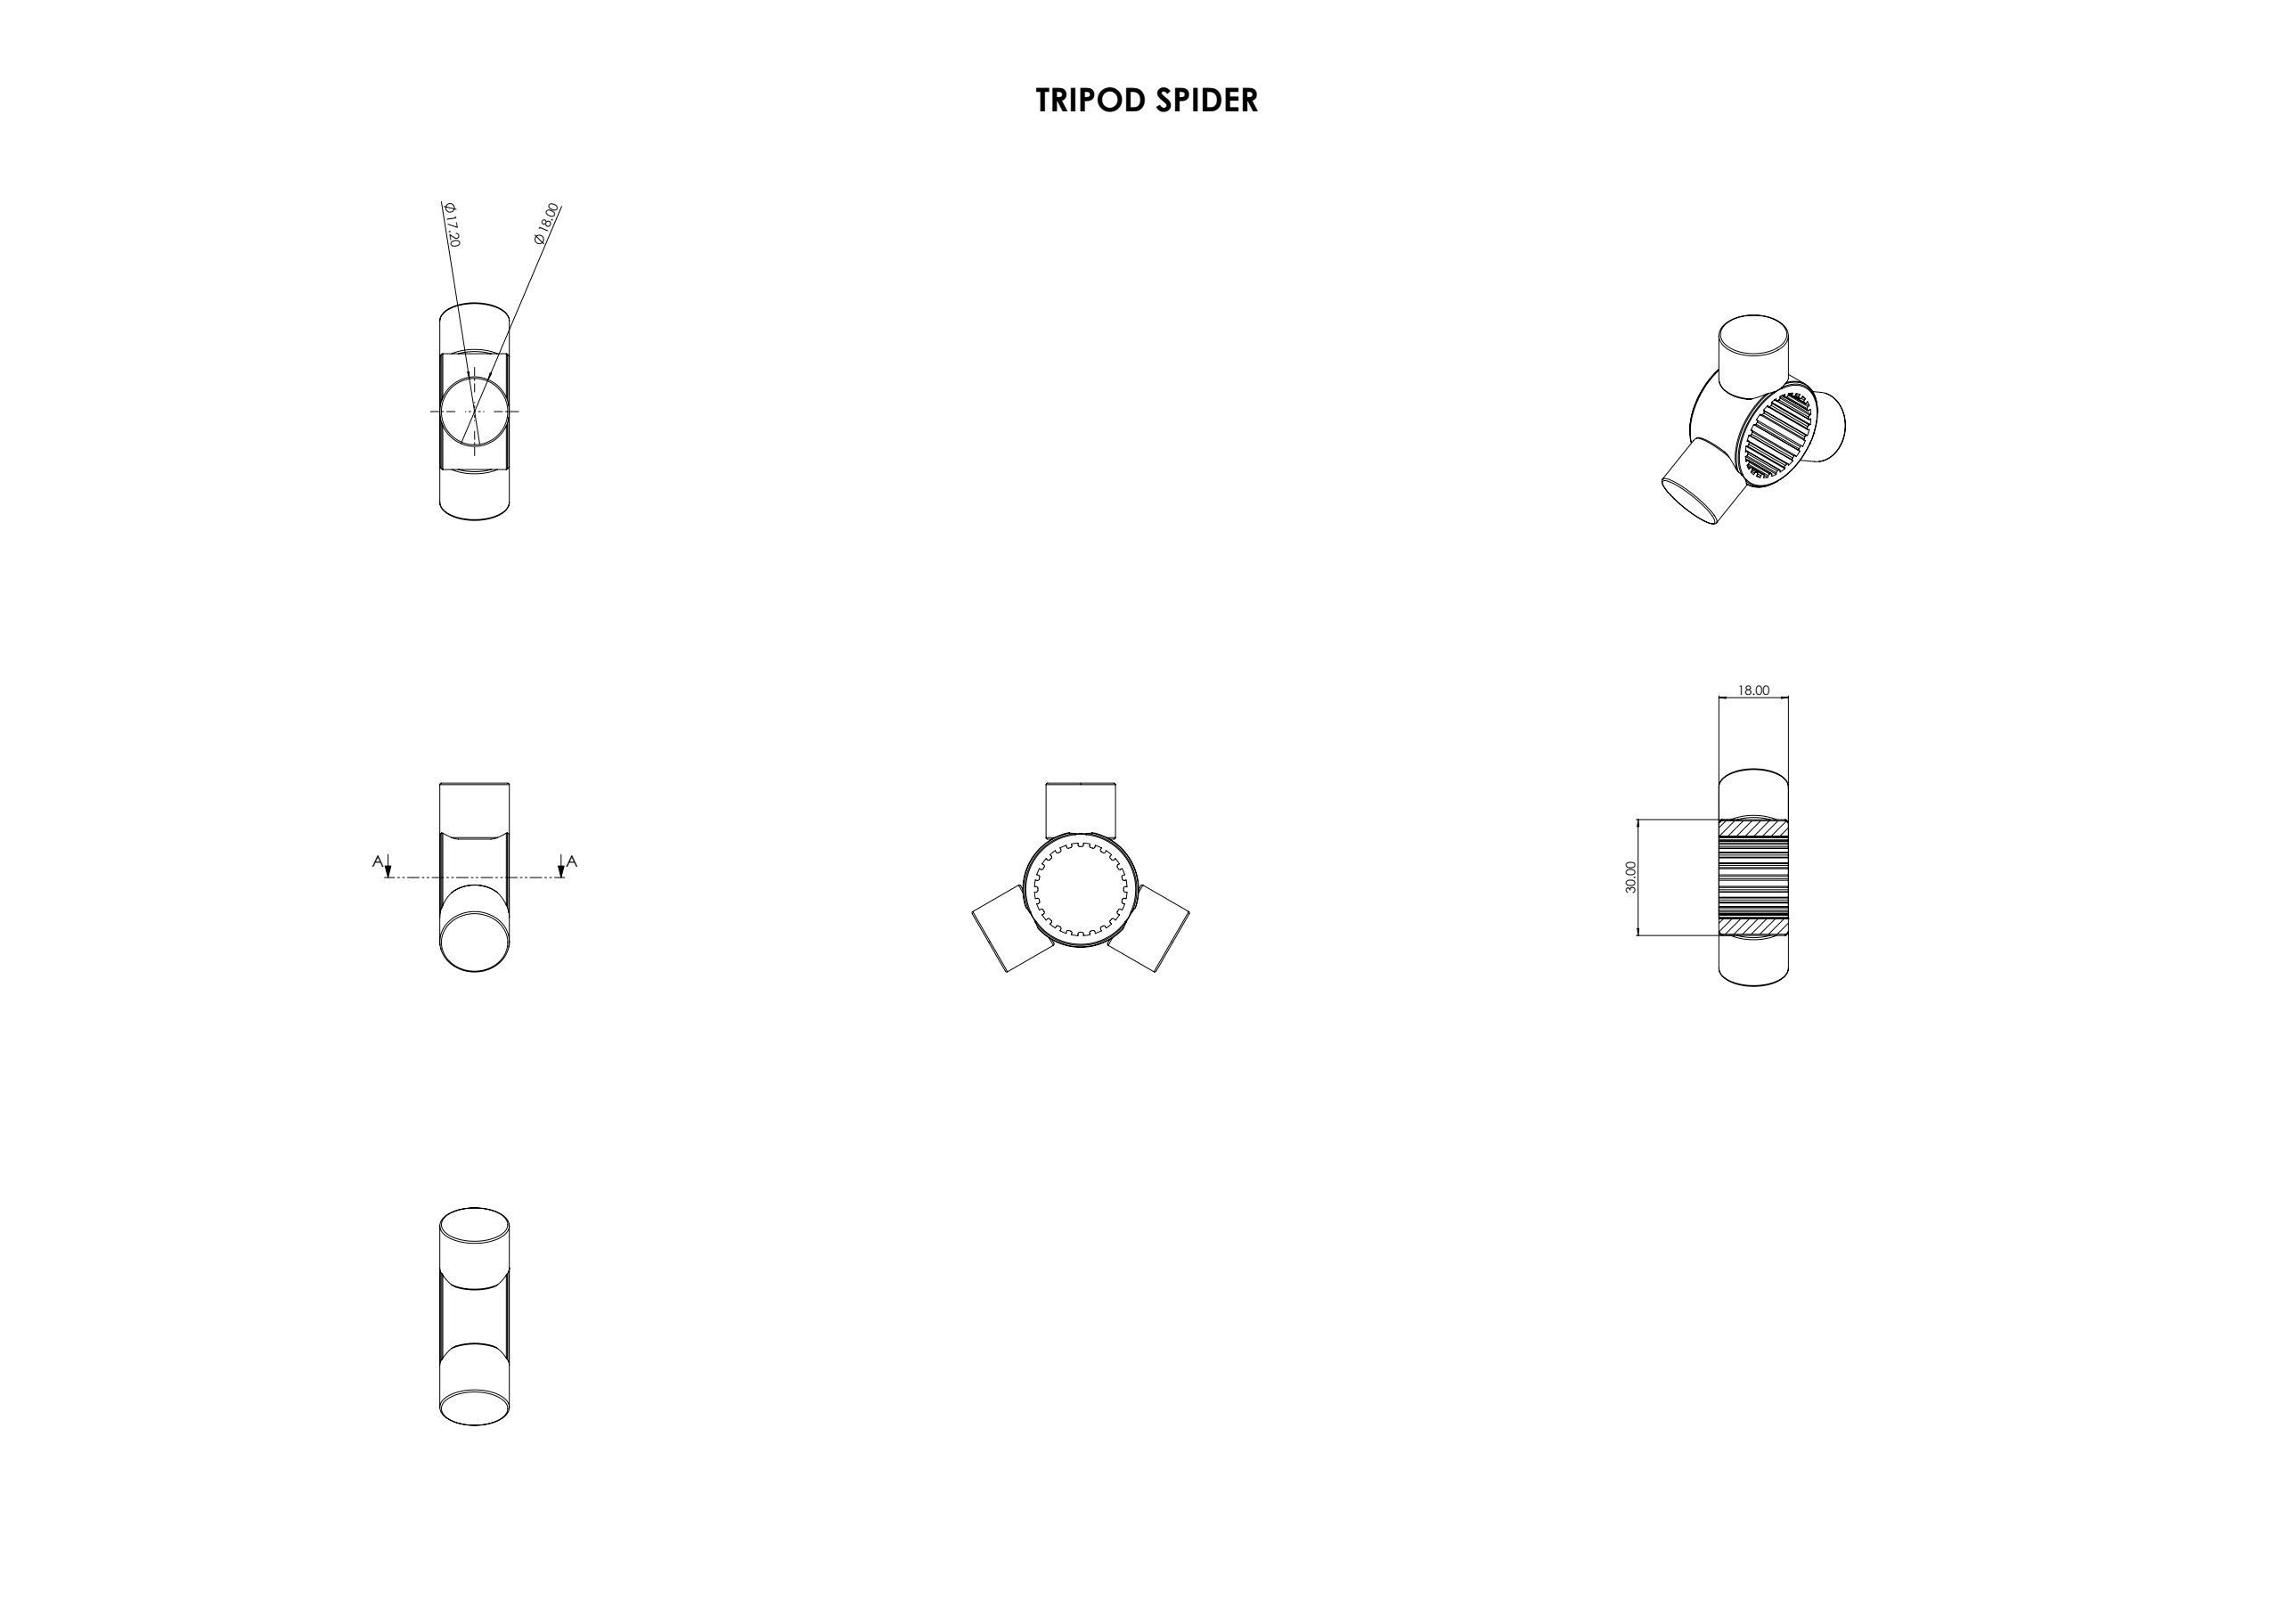
ISO-10303-21;
HEADER;
/* Generated by software containing ST-Developer
 * from STEP Tools, Inc. (www.steptools.com) 
 */

FILE_DESCRIPTION(
/* description */ (''),
/* implementation_level */ '2;1');

FILE_NAME(
/* name */ '14_Tripod_Spider.step',
/* time_stamp */ '2026-10-11T12:57:03-07:00',
/* author */ (''),
/* organization */ (''),
/* preprocessor_version */ 'ST-DEVELOPER v20.2',
/* originating_system */ 'Autodesk Translation Framework v15.15.0.0',
/* authorisation */ '');

FILE_SCHEMA (('AUTOMOTIVE_DESIGN { 1 0 10303 214 3 1 1 }'));
ENDSEC;

DATA;
#10=MECHANICAL_DESIGN_GEOMETRIC_PRESENTATION_REPRESENTATION('',(#269),#90374);
#235=SHAPE_REPRESENTATION_RELATIONSHIP('SRR','None',#90454,#252);
#252=ADVANCED_BREP_SHAPE_REPRESENTATION('',(#286),#90370);
#269=STYLED_ITEM('',(#90673),#286);
#286=MANIFOLD_SOLID_BREP('Body1',#40358);
#775=CONICAL_SURFACE('',#45071,14.7,0.78539816339743);
#776=CONICAL_SURFACE('',#45098,14.7,0.78539816339743);
#777=CONICAL_SURFACE('',#45102,14.7,0.78539816339743);
#778=CONICAL_SURFACE('',#45116,14.7,0.78539816339743);
#779=CONICAL_SURFACE('',#45117,14.7,0.78539816339743);
#780=CONICAL_SURFACE('',#45199,14.7,0.78539816339743);
#1010=TOROIDAL_SURFACE('',#44810,8.59999999999999,0.4);
#1011=TOROIDAL_SURFACE('',#44819,8.59999999999999,0.4);
#1012=TOROIDAL_SURFACE('',#44822,8.59999999999999,0.4);
#1013=TOROIDAL_SURFACE('',#44825,14.6,0.4);
#1014=TOROIDAL_SURFACE('',#44830,8.59999999999999,0.4);
#1015=TOROIDAL_SURFACE('',#44838,8.59999999999999,0.4);
#1016=TOROIDAL_SURFACE('',#44841,8.59999999999998,0.4);
#1017=TOROIDAL_SURFACE('',#44844,8.59999999999999,0.4);
#1018=TOROIDAL_SURFACE('',#44853,8.59999999999999,0.4);
#1019=TOROIDAL_SURFACE('',#44856,8.59999999999999,0.4);
#1020=TOROIDAL_SURFACE('',#45068,14.6,0.4);
#1021=TOROIDAL_SURFACE('',#45083,14.6,0.4);
#1022=TOROIDAL_SURFACE('',#45088,14.6,0.4);
#1023=TOROIDAL_SURFACE('',#45096,14.6,0.4);
#1024=TOROIDAL_SURFACE('',#45100,14.6,0.4);
#1025=TOROIDAL_SURFACE('',#45104,14.2343145750508,0.4);
#1026=TOROIDAL_SURFACE('',#45108,14.2343145750508,0.4);
#1027=TOROIDAL_SURFACE('',#45112,14.2343145750508,0.4);
#1028=TOROIDAL_SURFACE('',#45125,14.2343145750508,0.4);
#1029=TOROIDAL_SURFACE('',#45128,14.2343145750508,0.4);
#1030=TOROIDAL_SURFACE('',#45131,14.2343145750508,0.4);
#1108=FACE_BOUND('',#6808,.T.);
#1109=FACE_BOUND('',#6812,.T.);
#1736=PLANE('',#44818);
#1737=PLANE('',#44821);
#1738=PLANE('',#44824);
#1739=PLANE('',#44837);
#1740=PLANE('',#44840);
#1741=PLANE('',#44843);
#1742=PLANE('',#44852);
#1743=PLANE('',#44855);
#1744=PLANE('',#44858);
#1745=PLANE('',#44862);
#1746=PLANE('',#44863);
#1747=PLANE('',#44940);
#1748=PLANE('',#44941);
#1749=PLANE('',#45016);
#1750=PLANE('',#45019);
#1751=PLANE('',#45021);
#1752=PLANE('',#45023);
#1753=PLANE('',#45026);
#1754=PLANE('',#45029);
#1755=PLANE('',#45031);
#1756=PLANE('',#45033);
#1757=PLANE('',#45036);
#1758=PLANE('',#45039);
#1759=PLANE('',#45041);
#1760=PLANE('',#45043);
#1761=PLANE('',#45046);
#1762=PLANE('',#45049);
#1763=PLANE('',#45051);
#1764=PLANE('',#45053);
#1765=PLANE('',#45056);
#1766=PLANE('',#45059);
#1767=PLANE('',#45061);
#1768=PLANE('',#45063);
#1769=PLANE('',#45066);
#1770=PLANE('',#45074);
#1771=PLANE('',#45076);
#1772=PLANE('',#45078);
#1773=PLANE('',#45081);
#1774=PLANE('',#45093);
#1775=PLANE('',#45095);
#1776=PLANE('',#45119);
#1777=PLANE('',#45122);
#1778=PLANE('',#45124);
#1779=PLANE('',#45135);
#1780=PLANE('',#45137);
#1781=PLANE('',#45138);
#1782=PLANE('',#45141);
#1783=PLANE('',#45142);
#1784=PLANE('',#45143);
#1785=PLANE('',#45145);
#1786=PLANE('',#45148);
#1787=PLANE('',#45149);
#1788=PLANE('',#45150);
#1789=PLANE('',#45151);
#1790=PLANE('',#45153);
#1791=PLANE('',#45156);
#1792=PLANE('',#45157);
#1793=PLANE('',#45158);
#1794=PLANE('',#45159);
#1795=PLANE('',#45161);
#1796=PLANE('',#45164);
#1797=PLANE('',#45165);
#1798=PLANE('',#45166);
#1799=PLANE('',#45167);
#1800=PLANE('',#45169);
#1801=PLANE('',#45172);
#1802=PLANE('',#45173);
#1803=PLANE('',#45174);
#1804=PLANE('',#45175);
#1805=PLANE('',#45177);
#1806=PLANE('',#45180);
#1807=PLANE('',#45181);
#1808=PLANE('',#45182);
#1809=PLANE('',#45183);
#1810=PLANE('',#45185);
#1811=PLANE('',#45188);
#1812=PLANE('',#45189);
#1813=PLANE('',#45190);
#1814=PLANE('',#45191);
#1815=PLANE('',#45193);
#1816=PLANE('',#45196);
#1817=PLANE('',#45197);
#1818=PLANE('',#45198);
#2133=B_SPLINE_SURFACE_WITH_KNOTS('',3,3,((#89768,#89769,#89770,#89771,
#89772,#89773),(#89774,#89775,#89776,#89777,#89778,#89779),(#89780,#89781,
#89782,#89783,#89784,#89785),(#89786,#89787,#89788,#89789,#89790,#89791)),
 .UNSPECIFIED.,.F.,.F.,.F.,(4,4),(4,2,4),(0.,1.),(-0.340113319180834,-0.338813557833289,
-0.196228296217518),.UNSPECIFIED.);
#2134=B_SPLINE_SURFACE_WITH_KNOTS('',3,3,((#89792,#89793,#89794,#89795,
#89796,#89797),(#89798,#89799,#89800,#89801,#89802,#89803),(#89804,#89805,
#89806,#89807,#89808,#89809),(#89810,#89811,#89812,#89813,#89814,#89815)),
 .UNSPECIFIED.,.F.,.F.,.F.,(4,4),(4,2,4),(0.,1.),(-0.142585244788068,0.,
0.0012997781939584),.UNSPECIFIED.);
#2135=B_SPLINE_SURFACE_WITH_KNOTS('',3,3,((#89820,#89821,#89822,#89823,
#89824,#89825),(#89826,#89827,#89828,#89829,#89830,#89831),(#89832,#89833,
#89834,#89835,#89836,#89837),(#89838,#89839,#89840,#89841,#89842,#89843)),
 .UNSPECIFIED.,.F.,.F.,.F.,(4,4),(4,2,4),(0.,1.),(-0.340113319180884,-0.338813557833423,
-0.196228296217555),.UNSPECIFIED.);
#2136=B_SPLINE_SURFACE_WITH_KNOTS('',3,3,((#89844,#89845,#89846,#89847,
#89848,#89849),(#89850,#89851,#89852,#89853,#89854,#89855),(#89856,#89857,
#89858,#89859,#89860,#89861),(#89862,#89863,#89864,#89865,#89866,#89867)),
 .UNSPECIFIED.,.F.,.F.,.F.,(4,4),(4,2,4),(0.,1.),(-0.14258524478806,0.,
0.00129977819395902),.UNSPECIFIED.);
#2137=B_SPLINE_SURFACE_WITH_KNOTS('',3,3,((#89872,#89873,#89874,#89875,
#89876,#89877),(#89878,#89879,#89880,#89881,#89882,#89883),(#89884,#89885,
#89886,#89887,#89888,#89889),(#89890,#89891,#89892,#89893,#89894,#89895)),
 .UNSPECIFIED.,.F.,.F.,.F.,(4,4),(4,2,4),(0.,1.),(-0.340113319180875,-0.338813557833421,
-0.196228296217563),.UNSPECIFIED.);
#2138=B_SPLINE_SURFACE_WITH_KNOTS('',3,3,((#89896,#89897,#89898,#89899,
#89900,#89901),(#89902,#89903,#89904,#89905,#89906,#89907),(#89908,#89909,
#89910,#89911,#89912,#89913),(#89914,#89915,#89916,#89917,#89918,#89919)),
 .UNSPECIFIED.,.F.,.F.,.F.,(4,4),(4,2,4),(0.,1.),(-0.142585244788061,0.,
0.00129977819395621),.UNSPECIFIED.);
#2139=B_SPLINE_SURFACE_WITH_KNOTS('',3,3,((#89942,#89943,#89944,#89945,
#89946,#89947),(#89948,#89949,#89950,#89951,#89952,#89953),(#89954,#89955,
#89956,#89957,#89958,#89959),(#89960,#89961,#89962,#89963,#89964,#89965)),
 .UNSPECIFIED.,.F.,.F.,.F.,(4,4),(4,2,4),(0.,1.),(-0.142585233162139,0.,
0.00129978983276234),.UNSPECIFIED.);
#2140=B_SPLINE_SURFACE_WITH_KNOTS('',3,3,((#89966,#89967,#89968,#89969,
#89970,#89971),(#89972,#89973,#89974,#89975,#89976,#89977),(#89978,#89979,
#89980,#89981,#89982,#89983),(#89984,#89985,#89986,#89987,#89988,#89989)),
 .UNSPECIFIED.,.F.,.F.,.F.,(4,4),(4,2,4),(0.,1.),(-0.340113374972257,-0.338813601825611,
-0.19622835199583),.UNSPECIFIED.);
#2141=B_SPLINE_SURFACE_WITH_KNOTS('',3,3,((#89993,#89994,#89995,#89996,
#89997,#89998),(#89999,#90000,#90001,#90002,#90003,#90004),(#90005,#90006,
#90007,#90008,#90009,#90010),(#90011,#90012,#90013,#90014,#90015,#90016)),
 .UNSPECIFIED.,.F.,.F.,.F.,(4,4),(4,2,4),(0.,1.),(-0.142638931811887,0.,
0.00129978983275812),.UNSPECIFIED.);
#2142=B_SPLINE_SURFACE_WITH_KNOTS('',3,3,((#90017,#90018,#90019,#90020,
#90021,#90022),(#90023,#90024,#90025,#90026,#90027,#90028),(#90029,#90030,
#90031,#90032,#90033,#90034),(#90035,#90036,#90037,#90038,#90039,#90040)),
 .UNSPECIFIED.,.F.,.F.,.F.,(4,4),(4,2,4),(0.,1.),(-0.340113374972263,-0.338813601825613,
-0.196228351995831),.UNSPECIFIED.);
#2143=B_SPLINE_SURFACE_WITH_KNOTS('',3,3,((#90044,#90045,#90046,#90047,
#90048,#90049),(#90050,#90051,#90052,#90053,#90054,#90055),(#90056,#90057,
#90058,#90059,#90060,#90061),(#90062,#90063,#90064,#90065,#90066,#90067)),
 .UNSPECIFIED.,.F.,.F.,.F.,(4,4),(4,2,4),(0.,1.),(-0.142585233162046,0.,
0.00129978983284723),.UNSPECIFIED.);
#2144=B_SPLINE_SURFACE_WITH_KNOTS('',3,3,((#90068,#90069,#90070,#90071,
#90072,#90073),(#90074,#90075,#90076,#90077,#90078,#90079),(#90080,#90081,
#90082,#90083,#90084,#90085),(#90086,#90087,#90088,#90089,#90090,#90091)),
 .UNSPECIFIED.,.F.,.F.,.F.,(4,4),(4,2,4),(0.,1.),(-0.340113374972261,-0.338813601825616,
-0.196228351995834),.UNSPECIFIED.);
#4317=FACE_OUTER_BOUND('',#6782,.T.);
#4318=FACE_OUTER_BOUND('',#6783,.T.);
#4319=FACE_OUTER_BOUND('',#6784,.T.);
#4320=FACE_OUTER_BOUND('',#6785,.T.);
#4321=FACE_OUTER_BOUND('',#6786,.T.);
#4322=FACE_OUTER_BOUND('',#6787,.T.);
#4323=FACE_OUTER_BOUND('',#6788,.T.);
#4324=FACE_OUTER_BOUND('',#6789,.T.);
#4325=FACE_OUTER_BOUND('',#6790,.T.);
#4326=FACE_OUTER_BOUND('',#6791,.T.);
#4327=FACE_OUTER_BOUND('',#6792,.T.);
#4328=FACE_OUTER_BOUND('',#6793,.T.);
#4329=FACE_OUTER_BOUND('',#6794,.T.);
#4330=FACE_OUTER_BOUND('',#6795,.T.);
#4331=FACE_OUTER_BOUND('',#6796,.T.);
#4332=FACE_OUTER_BOUND('',#6797,.T.);
#4333=FACE_OUTER_BOUND('',#6798,.T.);
#4334=FACE_OUTER_BOUND('',#6799,.T.);
#4335=FACE_OUTER_BOUND('',#6800,.T.);
#4336=FACE_OUTER_BOUND('',#6801,.T.);
#4337=FACE_OUTER_BOUND('',#6802,.T.);
#4338=FACE_OUTER_BOUND('',#6803,.T.);
#4339=FACE_OUTER_BOUND('',#6804,.T.);
#4340=FACE_OUTER_BOUND('',#6805,.T.);
#4341=FACE_OUTER_BOUND('',#6806,.T.);
#4342=FACE_OUTER_BOUND('',#6807,.T.);
#4343=FACE_OUTER_BOUND('',#6809,.T.);
#4344=FACE_OUTER_BOUND('',#6810,.T.);
#4345=FACE_OUTER_BOUND('',#6811,.T.);
#4346=FACE_OUTER_BOUND('',#6813,.T.);
#4347=FACE_OUTER_BOUND('',#6814,.T.);
#4348=FACE_OUTER_BOUND('',#6815,.T.);
#4349=FACE_OUTER_BOUND('',#6816,.T.);
#4350=FACE_OUTER_BOUND('',#6817,.T.);
#4351=FACE_OUTER_BOUND('',#6818,.T.);
#4352=FACE_OUTER_BOUND('',#6819,.T.);
#4353=FACE_OUTER_BOUND('',#6820,.T.);
#4354=FACE_OUTER_BOUND('',#6821,.T.);
#4355=FACE_OUTER_BOUND('',#6822,.T.);
#4356=FACE_OUTER_BOUND('',#6823,.T.);
#4357=FACE_OUTER_BOUND('',#6824,.T.);
#4358=FACE_OUTER_BOUND('',#6825,.T.);
#4359=FACE_OUTER_BOUND('',#6826,.T.);
#4360=FACE_OUTER_BOUND('',#6827,.T.);
#4361=FACE_OUTER_BOUND('',#6828,.T.);
#4362=FACE_OUTER_BOUND('',#6829,.T.);
#4363=FACE_OUTER_BOUND('',#6830,.T.);
#4364=FACE_OUTER_BOUND('',#6831,.T.);
#4365=FACE_OUTER_BOUND('',#6832,.T.);
#4366=FACE_OUTER_BOUND('',#6833,.T.);
#4367=FACE_OUTER_BOUND('',#6834,.T.);
#4368=FACE_OUTER_BOUND('',#6835,.T.);
#4369=FACE_OUTER_BOUND('',#6836,.T.);
#4370=FACE_OUTER_BOUND('',#6837,.T.);
#4371=FACE_OUTER_BOUND('',#6838,.T.);
#4372=FACE_OUTER_BOUND('',#6839,.T.);
#4373=FACE_OUTER_BOUND('',#6840,.T.);
#4374=FACE_OUTER_BOUND('',#6841,.T.);
#4375=FACE_OUTER_BOUND('',#6842,.T.);
#4376=FACE_OUTER_BOUND('',#6843,.T.);
#4377=FACE_OUTER_BOUND('',#6844,.T.);
#4378=FACE_OUTER_BOUND('',#6845,.T.);
#4379=FACE_OUTER_BOUND('',#6846,.T.);
#4380=FACE_OUTER_BOUND('',#6847,.T.);
#4381=FACE_OUTER_BOUND('',#6848,.T.);
#4382=FACE_OUTER_BOUND('',#6849,.T.);
#4383=FACE_OUTER_BOUND('',#6850,.T.);
#4384=FACE_OUTER_BOUND('',#6851,.T.);
#4385=FACE_OUTER_BOUND('',#6852,.T.);
#4386=FACE_OUTER_BOUND('',#6853,.T.);
#4387=FACE_OUTER_BOUND('',#6854,.T.);
#4388=FACE_OUTER_BOUND('',#6855,.T.);
#4389=FACE_OUTER_BOUND('',#6856,.T.);
#4390=FACE_OUTER_BOUND('',#6857,.T.);
#4391=FACE_OUTER_BOUND('',#6858,.T.);
#4392=FACE_OUTER_BOUND('',#6859,.T.);
#4393=FACE_OUTER_BOUND('',#6860,.T.);
#4394=FACE_OUTER_BOUND('',#6861,.T.);
#4395=FACE_OUTER_BOUND('',#6862,.T.);
#4396=FACE_OUTER_BOUND('',#6863,.T.);
#4397=FACE_OUTER_BOUND('',#6864,.T.);
#4398=FACE_OUTER_BOUND('',#6865,.T.);
#4399=FACE_OUTER_BOUND('',#6866,.T.);
#4400=FACE_OUTER_BOUND('',#6867,.T.);
#4401=FACE_OUTER_BOUND('',#6868,.T.);
#4402=FACE_OUTER_BOUND('',#6869,.T.);
#4403=FACE_OUTER_BOUND('',#6870,.T.);
#4404=FACE_OUTER_BOUND('',#6871,.T.);
#4405=FACE_OUTER_BOUND('',#6872,.T.);
#4406=FACE_OUTER_BOUND('',#6873,.T.);
#4407=FACE_OUTER_BOUND('',#6874,.T.);
#4408=FACE_OUTER_BOUND('',#6875,.T.);
#4409=FACE_OUTER_BOUND('',#6876,.T.);
#4410=FACE_OUTER_BOUND('',#6877,.T.);
#4411=FACE_OUTER_BOUND('',#6878,.T.);
#4412=FACE_OUTER_BOUND('',#6879,.T.);
#4413=FACE_OUTER_BOUND('',#6880,.T.);
#4414=FACE_OUTER_BOUND('',#6881,.T.);
#4415=FACE_OUTER_BOUND('',#6882,.T.);
#4416=FACE_OUTER_BOUND('',#6883,.T.);
#4417=FACE_OUTER_BOUND('',#6884,.T.);
#4418=FACE_OUTER_BOUND('',#6885,.T.);
#4419=FACE_OUTER_BOUND('',#6886,.T.);
#4420=FACE_OUTER_BOUND('',#6887,.T.);
#4421=FACE_OUTER_BOUND('',#6888,.T.);
#4422=FACE_OUTER_BOUND('',#6889,.T.);
#4423=FACE_OUTER_BOUND('',#6890,.T.);
#4424=FACE_OUTER_BOUND('',#6891,.T.);
#4425=FACE_OUTER_BOUND('',#6892,.T.);
#4426=FACE_OUTER_BOUND('',#6893,.T.);
#4427=FACE_OUTER_BOUND('',#6894,.T.);
#4428=FACE_OUTER_BOUND('',#6895,.T.);
#4429=FACE_OUTER_BOUND('',#6896,.T.);
#4430=FACE_OUTER_BOUND('',#6897,.T.);
#4431=FACE_OUTER_BOUND('',#6898,.T.);
#4432=FACE_OUTER_BOUND('',#6899,.T.);
#4433=FACE_OUTER_BOUND('',#6900,.T.);
#4434=FACE_OUTER_BOUND('',#6901,.T.);
#4435=FACE_OUTER_BOUND('',#6902,.T.);
#4436=FACE_OUTER_BOUND('',#6903,.T.);
#4437=FACE_OUTER_BOUND('',#6904,.T.);
#4438=FACE_OUTER_BOUND('',#6905,.T.);
#4439=FACE_OUTER_BOUND('',#6906,.T.);
#4440=FACE_OUTER_BOUND('',#6907,.T.);
#4441=FACE_OUTER_BOUND('',#6908,.T.);
#4442=FACE_OUTER_BOUND('',#6909,.T.);
#4443=FACE_OUTER_BOUND('',#6910,.T.);
#4444=FACE_OUTER_BOUND('',#6911,.T.);
#4445=FACE_OUTER_BOUND('',#6912,.T.);
#4446=FACE_OUTER_BOUND('',#6913,.T.);
#4447=FACE_OUTER_BOUND('',#6914,.T.);
#4448=FACE_OUTER_BOUND('',#6915,.T.);
#4449=FACE_OUTER_BOUND('',#6916,.T.);
#4450=FACE_OUTER_BOUND('',#6917,.T.);
#4451=FACE_OUTER_BOUND('',#6918,.T.);
#4452=FACE_OUTER_BOUND('',#6919,.T.);
#4453=FACE_OUTER_BOUND('',#6920,.T.);
#4454=FACE_OUTER_BOUND('',#6921,.T.);
#4455=FACE_OUTER_BOUND('',#6922,.T.);
#4456=FACE_OUTER_BOUND('',#6923,.T.);
#4457=FACE_OUTER_BOUND('',#6924,.T.);
#4458=FACE_OUTER_BOUND('',#6925,.T.);
#4459=FACE_OUTER_BOUND('',#6926,.T.);
#4460=FACE_OUTER_BOUND('',#6927,.T.);
#4461=FACE_OUTER_BOUND('',#6928,.T.);
#4462=FACE_OUTER_BOUND('',#6929,.T.);
#4463=FACE_OUTER_BOUND('',#6930,.T.);
#4464=FACE_OUTER_BOUND('',#6931,.T.);
#4465=FACE_OUTER_BOUND('',#6932,.T.);
#4466=FACE_OUTER_BOUND('',#6933,.T.);
#4467=FACE_OUTER_BOUND('',#6934,.T.);
#4468=FACE_OUTER_BOUND('',#6935,.T.);
#4469=FACE_OUTER_BOUND('',#6936,.T.);
#4470=FACE_OUTER_BOUND('',#6937,.T.);
#4471=FACE_OUTER_BOUND('',#6938,.T.);
#4472=FACE_OUTER_BOUND('',#6939,.T.);
#4473=FACE_OUTER_BOUND('',#6940,.T.);
#4474=FACE_OUTER_BOUND('',#6941,.T.);
#4475=FACE_OUTER_BOUND('',#6942,.T.);
#4476=FACE_OUTER_BOUND('',#6943,.T.);
#4477=FACE_OUTER_BOUND('',#6944,.T.);
#4478=FACE_OUTER_BOUND('',#6945,.T.);
#4479=FACE_OUTER_BOUND('',#6946,.T.);
#4480=FACE_OUTER_BOUND('',#6947,.T.);
#4481=FACE_OUTER_BOUND('',#6948,.T.);
#4482=FACE_OUTER_BOUND('',#6949,.T.);
#4483=FACE_OUTER_BOUND('',#6950,.T.);
#4484=FACE_OUTER_BOUND('',#6951,.T.);
#4485=FACE_OUTER_BOUND('',#6952,.T.);
#4486=FACE_OUTER_BOUND('',#6953,.T.);
#4487=FACE_OUTER_BOUND('',#6954,.T.);
#4488=FACE_OUTER_BOUND('',#6955,.T.);
#4489=FACE_OUTER_BOUND('',#6956,.T.);
#4490=FACE_OUTER_BOUND('',#6957,.T.);
#4491=FACE_OUTER_BOUND('',#6958,.T.);
#4492=FACE_OUTER_BOUND('',#6959,.T.);
#4493=FACE_OUTER_BOUND('',#6960,.T.);
#4494=FACE_OUTER_BOUND('',#6961,.T.);
#4495=FACE_OUTER_BOUND('',#6962,.T.);
#4496=FACE_OUTER_BOUND('',#6963,.T.);
#4497=FACE_OUTER_BOUND('',#6964,.T.);
#4498=FACE_OUTER_BOUND('',#6965,.T.);
#4499=FACE_OUTER_BOUND('',#6966,.T.);
#4500=FACE_OUTER_BOUND('',#6967,.T.);
#4501=FACE_OUTER_BOUND('',#6968,.T.);
#4502=FACE_OUTER_BOUND('',#6969,.T.);
#4503=FACE_OUTER_BOUND('',#6970,.T.);
#4504=FACE_OUTER_BOUND('',#6971,.T.);
#4505=FACE_OUTER_BOUND('',#6972,.T.);
#4506=FACE_OUTER_BOUND('',#6973,.T.);
#4507=FACE_OUTER_BOUND('',#6974,.T.);
#4508=FACE_OUTER_BOUND('',#6975,.T.);
#4509=FACE_OUTER_BOUND('',#6976,.T.);
#4510=FACE_OUTER_BOUND('',#6977,.T.);
#4511=FACE_OUTER_BOUND('',#6978,.T.);
#4512=FACE_OUTER_BOUND('',#6979,.T.);
#4513=FACE_OUTER_BOUND('',#6980,.T.);
#4514=FACE_OUTER_BOUND('',#6981,.T.);
#4515=FACE_OUTER_BOUND('',#6982,.T.);
#4516=FACE_OUTER_BOUND('',#6983,.T.);
#6782=EDGE_LOOP('',(#35975,#35976,#35977,#35978,#35979));
#6783=EDGE_LOOP('',(#35980,#35981,#35982,#35983,#35984,#35985,#35986,#35987,
#35988,#35989,#35990,#35991,#35992,#35993,#35994,#35995,#35996,#35997,#35998,
#35999,#36000,#36001));
#6784=EDGE_LOOP('',(#36002));
#6785=EDGE_LOOP('',(#36003,#36004,#36005,#36006));
#6786=EDGE_LOOP('',(#36007,#36008));
#6787=EDGE_LOOP('',(#36009,#36010,#36011,#36012));
#6788=EDGE_LOOP('',(#36013,#36014));
#6789=EDGE_LOOP('',(#36015,#36016,#36017,#36018));
#6790=EDGE_LOOP('',(#36019,#36020,#36021,#36022,#36023,#36024,#36025,#36026,
#36027,#36028,#36029,#36030));
#6791=EDGE_LOOP('',(#36031,#36032,#36033,#36034));
#6792=EDGE_LOOP('',(#36035,#36036,#36037,#36038,#36039,#36040,#36041,#36042,
#36043,#36044,#36045,#36046,#36047,#36048,#36049,#36050,#36051,#36052,#36053,
#36054,#36055));
#6793=EDGE_LOOP('',(#36056));
#6794=EDGE_LOOP('',(#36057,#36058,#36059,#36060));
#6795=EDGE_LOOP('',(#36061,#36062));
#6796=EDGE_LOOP('',(#36063,#36064,#36065,#36066));
#6797=EDGE_LOOP('',(#36067,#36068));
#6798=EDGE_LOOP('',(#36069,#36070,#36071,#36072,#36073));
#6799=EDGE_LOOP('',(#36074,#36075,#36076,#36077,#36078,#36079,#36080,#36081,
#36082,#36083,#36084,#36085,#36086,#36087,#36088,#36089,#36090,#36091,#36092,
#36093,#36094,#36095));
#6800=EDGE_LOOP('',(#36096));
#6801=EDGE_LOOP('',(#36097,#36098,#36099,#36100));
#6802=EDGE_LOOP('',(#36101,#36102));
#6803=EDGE_LOOP('',(#36103,#36104,#36105,#36106));
#6804=EDGE_LOOP('',(#36107,#36108));
#6805=EDGE_LOOP('',(#36109,#36110,#36111,#36112));
#6806=EDGE_LOOP('',(#36113,#36114,#36115,#36116));
#6807=EDGE_LOOP('',(#36117,#36118,#36119,#36120,#36121,#36122,#36123,#36124,
#36125));
#6808=EDGE_LOOP('',(#36126,#36127,#36128,#36129,#36130,#36131,#36132,#36133,
#36134,#36135,#36136,#36137,#36138,#36139,#36140,#36141,#36142,#36143,#36144,
#36145,#36146,#36147,#36148,#36149,#36150,#36151,#36152,#36153,#36154,#36155,
#36156,#36157,#36158,#36159,#36160,#36161,#36162,#36163,#36164,#36165,#36166,
#36167,#36168,#36169,#36170,#36171,#36172,#36173,#36174,#36175,#36176,#36177,
#36178,#36179,#36180,#36181,#36182,#36183,#36184,#36185,#36186,#36187,#36188,
#36189,#36190,#36191,#36192,#36193,#36194,#36195,#36196,#36197,#36198,#36199,
#36200,#36201,#36202,#36203,#36204,#36205,#36206,#36207,#36208,#36209,#36210,
#36211,#36212,#36213,#36214,#36215,#36216,#36217,#36218,#36219,#36220,#36221,
#36222,#36223,#36224,#36225,#36226,#36227,#36228,#36229,#36230,#36231,#36232,
#36233,#36234,#36235,#36236,#36237,#36238,#36239,#36240,#36241,#36242,#36243,
#36244,#36245,#36246,#36247,#36248,#36249,#36250,#36251,#36252,#36253,#36254,
#36255,#36256,#36257,#36258,#36259,#36260,#36261,#36262,#36263,#36264,#36265,
#36266,#36267,#36268,#36269));
#6809=EDGE_LOOP('',(#36270,#36271,#36272,#36273));
#6810=EDGE_LOOP('',(#36274,#36275,#36276,#36277));
#6811=EDGE_LOOP('',(#36278,#36279,#36280,#36281,#36282,#36283,#36284,#36285,
#36286));
#6812=EDGE_LOOP('',(#36287,#36288,#36289,#36290,#36291,#36292,#36293,#36294,
#36295,#36296,#36297,#36298,#36299,#36300,#36301,#36302,#36303,#36304,#36305,
#36306,#36307,#36308,#36309,#36310,#36311,#36312,#36313,#36314,#36315,#36316,
#36317,#36318,#36319,#36320,#36321,#36322,#36323,#36324,#36325,#36326,#36327,
#36328,#36329,#36330,#36331,#36332,#36333,#36334,#36335,#36336,#36337,#36338,
#36339,#36340,#36341,#36342,#36343,#36344,#36345,#36346,#36347,#36348,#36349,
#36350,#36351,#36352,#36353,#36354,#36355,#36356,#36357,#36358,#36359,#36360,
#36361,#36362,#36363,#36364,#36365,#36366,#36367,#36368,#36369,#36370,#36371,
#36372,#36373,#36374,#36375,#36376,#36377,#36378,#36379,#36380,#36381,#36382,
#36383,#36384,#36385,#36386,#36387,#36388,#36389,#36390,#36391,#36392,#36393,
#36394,#36395,#36396,#36397,#36398,#36399,#36400,#36401,#36402,#36403,#36404,
#36405,#36406,#36407,#36408,#36409,#36410,#36411,#36412,#36413,#36414,#36415,
#36416,#36417,#36418,#36419,#36420,#36421,#36422,#36423,#36424,#36425,#36426,
#36427,#36428,#36429,#36430));
#6813=EDGE_LOOP('',(#36431,#36432,#36433,#36434));
#6814=EDGE_LOOP('',(#36435,#36436,#36437,#36438));
#6815=EDGE_LOOP('',(#36439,#36440,#36441,#36442));
#6816=EDGE_LOOP('',(#36443,#36444,#36445,#36446));
#6817=EDGE_LOOP('',(#36447,#36448,#36449,#36450));
#6818=EDGE_LOOP('',(#36451,#36452,#36453,#36454));
#6819=EDGE_LOOP('',(#36455,#36456,#36457,#36458));
#6820=EDGE_LOOP('',(#36459,#36460,#36461,#36462));
#6821=EDGE_LOOP('',(#36463,#36464,#36465,#36466));
#6822=EDGE_LOOP('',(#36467,#36468,#36469,#36470));
#6823=EDGE_LOOP('',(#36471,#36472,#36473,#36474));
#6824=EDGE_LOOP('',(#36475,#36476,#36477,#36478));
#6825=EDGE_LOOP('',(#36479,#36480,#36481,#36482));
#6826=EDGE_LOOP('',(#36483,#36484,#36485,#36486));
#6827=EDGE_LOOP('',(#36487,#36488,#36489,#36490));
#6828=EDGE_LOOP('',(#36491,#36492,#36493,#36494));
#6829=EDGE_LOOP('',(#36495,#36496,#36497,#36498));
#6830=EDGE_LOOP('',(#36499,#36500,#36501,#36502));
#6831=EDGE_LOOP('',(#36503,#36504,#36505,#36506));
#6832=EDGE_LOOP('',(#36507,#36508,#36509,#36510));
#6833=EDGE_LOOP('',(#36511,#36512,#36513,#36514));
#6834=EDGE_LOOP('',(#36515,#36516,#36517,#36518));
#6835=EDGE_LOOP('',(#36519,#36520,#36521,#36522));
#6836=EDGE_LOOP('',(#36523,#36524,#36525,#36526));
#6837=EDGE_LOOP('',(#36527,#36528,#36529,#36530));
#6838=EDGE_LOOP('',(#36531,#36532,#36533,#36534));
#6839=EDGE_LOOP('',(#36535,#36536,#36537,#36538));
#6840=EDGE_LOOP('',(#36539,#36540,#36541,#36542));
#6841=EDGE_LOOP('',(#36543,#36544,#36545,#36546));
#6842=EDGE_LOOP('',(#36547,#36548,#36549,#36550));
#6843=EDGE_LOOP('',(#36551,#36552,#36553,#36554));
#6844=EDGE_LOOP('',(#36555,#36556,#36557,#36558));
#6845=EDGE_LOOP('',(#36559,#36560,#36561,#36562));
#6846=EDGE_LOOP('',(#36563,#36564,#36565,#36566));
#6847=EDGE_LOOP('',(#36567,#36568,#36569,#36570));
#6848=EDGE_LOOP('',(#36571,#36572,#36573,#36574));
#6849=EDGE_LOOP('',(#36575,#36576,#36577,#36578));
#6850=EDGE_LOOP('',(#36579,#36580,#36581,#36582));
#6851=EDGE_LOOP('',(#36583,#36584,#36585,#36586));
#6852=EDGE_LOOP('',(#36587,#36588,#36589,#36590));
#6853=EDGE_LOOP('',(#36591,#36592,#36593,#36594));
#6854=EDGE_LOOP('',(#36595,#36596,#36597,#36598));
#6855=EDGE_LOOP('',(#36599,#36600,#36601,#36602));
#6856=EDGE_LOOP('',(#36603,#36604,#36605,#36606));
#6857=EDGE_LOOP('',(#36607,#36608,#36609,#36610));
#6858=EDGE_LOOP('',(#36611,#36612,#36613,#36614));
#6859=EDGE_LOOP('',(#36615,#36616,#36617,#36618));
#6860=EDGE_LOOP('',(#36619,#36620,#36621,#36622));
#6861=EDGE_LOOP('',(#36623,#36624,#36625,#36626));
#6862=EDGE_LOOP('',(#36627,#36628,#36629,#36630));
#6863=EDGE_LOOP('',(#36631,#36632,#36633,#36634));
#6864=EDGE_LOOP('',(#36635,#36636,#36637,#36638));
#6865=EDGE_LOOP('',(#36639,#36640,#36641,#36642));
#6866=EDGE_LOOP('',(#36643,#36644,#36645,#36646));
#6867=EDGE_LOOP('',(#36647,#36648,#36649,#36650));
#6868=EDGE_LOOP('',(#36651,#36652,#36653,#36654));
#6869=EDGE_LOOP('',(#36655,#36656,#36657,#36658));
#6870=EDGE_LOOP('',(#36659,#36660,#36661,#36662));
#6871=EDGE_LOOP('',(#36663,#36664,#36665,#36666));
#6872=EDGE_LOOP('',(#36667,#36668,#36669,#36670));
#6873=EDGE_LOOP('',(#36671,#36672,#36673,#36674));
#6874=EDGE_LOOP('',(#36675,#36676,#36677,#36678));
#6875=EDGE_LOOP('',(#36679,#36680,#36681,#36682));
#6876=EDGE_LOOP('',(#36683,#36684,#36685,#36686));
#6877=EDGE_LOOP('',(#36687,#36688,#36689,#36690));
#6878=EDGE_LOOP('',(#36691,#36692,#36693,#36694));
#6879=EDGE_LOOP('',(#36695,#36696,#36697,#36698,#36699,#36700,#36701,#36702,
#36703,#36704,#36705,#36706));
#6880=EDGE_LOOP('',(#36707,#36708,#36709,#36710));
#6881=EDGE_LOOP('',(#36711,#36712,#36713,#36714,#36715,#36716,#36717,#36718,
#36719,#36720,#36721,#36722));
#6882=EDGE_LOOP('',(#36723,#36724,#36725,#36726));
#6883=EDGE_LOOP('',(#36727,#36728,#36729,#36730));
#6884=EDGE_LOOP('',(#36731,#36732,#36733,#36734));
#6885=EDGE_LOOP('',(#36735,#36736,#36737,#36738));
#6886=EDGE_LOOP('',(#36739,#36740,#36741,#36742));
#6887=EDGE_LOOP('',(#36743,#36744,#36745,#36746));
#6888=EDGE_LOOP('',(#36747,#36748,#36749,#36750));
#6889=EDGE_LOOP('',(#36751,#36752,#36753,#36754));
#6890=EDGE_LOOP('',(#36755,#36756,#36757,#36758));
#6891=EDGE_LOOP('',(#36759,#36760,#36761));
#6892=EDGE_LOOP('',(#36762,#36763,#36764));
#6893=EDGE_LOOP('',(#36765,#36766,#36767,#36768));
#6894=EDGE_LOOP('',(#36769,#36770,#36771));
#6895=EDGE_LOOP('',(#36772,#36773,#36774));
#6896=EDGE_LOOP('',(#36775,#36776,#36777,#36778));
#6897=EDGE_LOOP('',(#36779,#36780,#36781));
#6898=EDGE_LOOP('',(#36782,#36783,#36784));
#6899=EDGE_LOOP('',(#36785,#36786,#36787,#36788));
#6900=EDGE_LOOP('',(#36789,#36790,#36791,#36792));
#6901=EDGE_LOOP('',(#36793,#36794,#36795,#36796));
#6902=EDGE_LOOP('',(#36797,#36798,#36799,#36800));
#6903=EDGE_LOOP('',(#36801,#36802,#36803,#36804));
#6904=EDGE_LOOP('',(#36805,#36806,#36807,#36808));
#6905=EDGE_LOOP('',(#36809,#36810,#36811,#36812));
#6906=EDGE_LOOP('',(#36813,#36814,#36815,#36816));
#6907=EDGE_LOOP('',(#36817,#36818,#36819,#36820));
#6908=EDGE_LOOP('',(#36821,#36822,#36823,#36824));
#6909=EDGE_LOOP('',(#36825,#36826,#36827));
#6910=EDGE_LOOP('',(#36828,#36829,#36830));
#6911=EDGE_LOOP('',(#36831,#36832,#36833,#36834));
#6912=EDGE_LOOP('',(#36835,#36836,#36837));
#6913=EDGE_LOOP('',(#36838,#36839,#36840));
#6914=EDGE_LOOP('',(#36841,#36842,#36843,#36844));
#6915=EDGE_LOOP('',(#36845,#36846,#36847));
#6916=EDGE_LOOP('',(#36848,#36849,#36850));
#6917=EDGE_LOOP('',(#36851,#36852,#36853,#36854));
#6918=EDGE_LOOP('',(#36855,#36856,#36857,#36858));
#6919=EDGE_LOOP('',(#36859,#36860,#36861,#36862));
#6920=EDGE_LOOP('',(#36863,#36864,#36865,#36866));
#6921=EDGE_LOOP('',(#36867,#36868,#36869,#36870));
#6922=EDGE_LOOP('',(#36871,#36872,#36873,#36874));
#6923=EDGE_LOOP('',(#36875,#36876,#36877,#36878));
#6924=EDGE_LOOP('',(#36879,#36880,#36881,#36882));
#6925=EDGE_LOOP('',(#36883,#36884,#36885,#36886));
#6926=EDGE_LOOP('',(#36887,#36888,#36889,#36890));
#6927=EDGE_LOOP('',(#36891,#36892,#36893,#36894));
#6928=EDGE_LOOP('',(#36895,#36896,#36897,#36898));
#6929=EDGE_LOOP('',(#36899,#36900,#36901,#36902));
#6930=EDGE_LOOP('',(#36903,#36904,#36905,#36906));
#6931=EDGE_LOOP('',(#36907,#36908,#36909,#36910));
#6932=EDGE_LOOP('',(#36911,#36912,#36913,#36914));
#6933=EDGE_LOOP('',(#36915,#36916,#36917,#36918));
#6934=EDGE_LOOP('',(#36919,#36920,#36921,#36922));
#6935=EDGE_LOOP('',(#36923,#36924,#36925,#36926));
#6936=EDGE_LOOP('',(#36927,#36928,#36929,#36930));
#6937=EDGE_LOOP('',(#36931,#36932,#36933,#36934));
#6938=EDGE_LOOP('',(#36935,#36936,#36937,#36938));
#6939=EDGE_LOOP('',(#36939,#36940,#36941,#36942));
#6940=EDGE_LOOP('',(#36943,#36944,#36945,#36946));
#6941=EDGE_LOOP('',(#36947,#36948,#36949,#36950));
#6942=EDGE_LOOP('',(#36951,#36952,#36953,#36954));
#6943=EDGE_LOOP('',(#36955,#36956,#36957,#36958));
#6944=EDGE_LOOP('',(#36959,#36960,#36961,#36962));
#6945=EDGE_LOOP('',(#36963,#36964,#36965,#36966));
#6946=EDGE_LOOP('',(#36967,#36968,#36969,#36970));
#6947=EDGE_LOOP('',(#36971,#36972,#36973,#36974));
#6948=EDGE_LOOP('',(#36975,#36976,#36977,#36978));
#6949=EDGE_LOOP('',(#36979,#36980,#36981,#36982));
#6950=EDGE_LOOP('',(#36983,#36984,#36985,#36986));
#6951=EDGE_LOOP('',(#36987,#36988,#36989,#36990));
#6952=EDGE_LOOP('',(#36991,#36992,#36993,#36994));
#6953=EDGE_LOOP('',(#36995,#36996,#36997,#36998));
#6954=EDGE_LOOP('',(#36999,#37000,#37001,#37002));
#6955=EDGE_LOOP('',(#37003,#37004,#37005,#37006));
#6956=EDGE_LOOP('',(#37007,#37008,#37009,#37010));
#6957=EDGE_LOOP('',(#37011,#37012,#37013,#37014));
#6958=EDGE_LOOP('',(#37015,#37016,#37017,#37018));
#6959=EDGE_LOOP('',(#37019,#37020,#37021,#37022));
#6960=EDGE_LOOP('',(#37023,#37024,#37025,#37026));
#6961=EDGE_LOOP('',(#37027,#37028,#37029,#37030));
#6962=EDGE_LOOP('',(#37031,#37032,#37033,#37034));
#6963=EDGE_LOOP('',(#37035,#37036,#37037,#37038));
#6964=EDGE_LOOP('',(#37039,#37040,#37041,#37042));
#6965=EDGE_LOOP('',(#37043,#37044,#37045,#37046));
#6966=EDGE_LOOP('',(#37047,#37048,#37049,#37050));
#6967=EDGE_LOOP('',(#37051,#37052,#37053,#37054));
#6968=EDGE_LOOP('',(#37055,#37056,#37057,#37058));
#6969=EDGE_LOOP('',(#37059,#37060,#37061,#37062));
#6970=EDGE_LOOP('',(#37063,#37064,#37065,#37066));
#6971=EDGE_LOOP('',(#37067,#37068,#37069,#37070));
#6972=EDGE_LOOP('',(#37071,#37072,#37073,#37074));
#6973=EDGE_LOOP('',(#37075,#37076,#37077,#37078));
#6974=EDGE_LOOP('',(#37079,#37080,#37081,#37082));
#6975=EDGE_LOOP('',(#37083,#37084,#37085,#37086));
#6976=EDGE_LOOP('',(#37087,#37088,#37089,#37090));
#6977=EDGE_LOOP('',(#37091,#37092,#37093,#37094));
#6978=EDGE_LOOP('',(#37095,#37096,#37097,#37098));
#6979=EDGE_LOOP('',(#37099,#37100,#37101,#37102));
#6980=EDGE_LOOP('',(#37103,#37104,#37105,#37106));
#6981=EDGE_LOOP('',(#37107,#37108,#37109,#37110));
#6982=EDGE_LOOP('',(#37111,#37112,#37113,#37114));
#6983=EDGE_LOOP('',(#37115,#37116,#37117,#37118));
#9179=CIRCLE('',#44811,8.59999999999999);
#9180=CIRCLE('',#44812,0.4);
#9181=CIRCLE('',#44813,8.99999999999999);
#9182=CIRCLE('',#44814,8.99999999999999);
#9183=CIRCLE('',#44816,8.99999999999999);
#9184=CIRCLE('',#44817,8.99999999999999);
#9185=CIRCLE('',#44820,8.59999999999999);
#9186=CIRCLE('',#44823,8.59999999999999);
#9187=CIRCLE('',#44826,15.);
#9188=CIRCLE('',#44827,14.8828427124746);
#9189=CIRCLE('',#44829,15.);
#9190=CIRCLE('',#44831,8.59999999999999);
#9191=CIRCLE('',#44832,0.4);
#9192=CIRCLE('',#44833,8.99999999999999);
#9193=CIRCLE('',#44835,8.99999999999999);
#9194=CIRCLE('',#44836,8.99999999999999);
#9195=CIRCLE('',#44839,8.59999999999999);
#9196=CIRCLE('',#44842,8.59999999999999);
#9197=CIRCLE('',#44845,8.59999999999999);
#9198=CIRCLE('',#44846,0.4);
#9199=CIRCLE('',#44847,8.99999999999999);
#9200=CIRCLE('',#44848,8.99999999999999);
#9201=CIRCLE('',#44850,8.99999999999999);
#9202=CIRCLE('',#44851,8.99999999999999);
#9203=CIRCLE('',#44854,8.59999999999998);
#9204=CIRCLE('',#44857,8.59999999999998);
#9205=CIRCLE('',#44860,0.4);
#9206=CIRCLE('',#44861,0.4);
#9207=CIRCLE('',#44864,14.2343145750508);
#9208=CIRCLE('',#44865,14.2343145750508);
#9209=CIRCLE('',#44866,14.2343145750508);
#9210=CIRCLE('',#44867,0.4);
#9211=CIRCLE('',#44868,12.);
#9212=CIRCLE('',#44869,0.4);
#9213=CIRCLE('',#44870,0.4);
#9214=CIRCLE('',#44871,12.);
#9215=CIRCLE('',#44872,0.4);
#9216=CIRCLE('',#44873,0.4);
#9217=CIRCLE('',#44874,12.);
#9218=CIRCLE('',#44875,0.4);
#9219=CIRCLE('',#44876,0.4);
#9220=CIRCLE('',#44877,12.);
#9221=CIRCLE('',#44878,0.4);
#9222=CIRCLE('',#44879,0.4);
#9223=CIRCLE('',#44880,12.);
#9224=CIRCLE('',#44881,0.4);
#9225=CIRCLE('',#44882,0.4);
#9226=CIRCLE('',#44883,12.);
#9227=CIRCLE('',#44884,0.4);
#9228=CIRCLE('',#44885,0.4);
#9229=CIRCLE('',#44886,12.);
#9230=CIRCLE('',#44887,0.4);
#9231=CIRCLE('',#44888,0.4);
#9232=CIRCLE('',#44889,12.);
#9233=CIRCLE('',#44890,0.4);
#9234=CIRCLE('',#44891,0.4);
#9235=CIRCLE('',#44892,12.);
#9236=CIRCLE('',#44893,0.4);
#9237=CIRCLE('',#44894,0.4);
#9238=CIRCLE('',#44895,12.);
#9239=CIRCLE('',#44896,0.4);
#9240=CIRCLE('',#44897,0.4);
#9241=CIRCLE('',#44898,12.);
#9242=CIRCLE('',#44899,0.4);
#9243=CIRCLE('',#44900,0.4);
#9244=CIRCLE('',#44901,12.);
#9245=CIRCLE('',#44902,0.4);
#9246=CIRCLE('',#44903,0.4);
#9247=CIRCLE('',#44904,12.);
#9248=CIRCLE('',#44905,0.4);
#9249=CIRCLE('',#44906,0.4);
#9250=CIRCLE('',#44907,12.);
#9251=CIRCLE('',#44908,0.4);
#9252=CIRCLE('',#44909,0.4);
#9253=CIRCLE('',#44910,12.);
#9254=CIRCLE('',#44911,0.4);
#9255=CIRCLE('',#44912,0.4);
#9256=CIRCLE('',#44913,12.);
#9257=CIRCLE('',#44914,0.4);
#9258=CIRCLE('',#44915,0.4);
#9259=CIRCLE('',#44916,12.);
#9260=CIRCLE('',#44917,0.4);
#9261=CIRCLE('',#44918,0.4);
#9262=CIRCLE('',#44919,12.);
#9263=CIRCLE('',#44920,0.4);
#9264=CIRCLE('',#44921,0.4);
#9265=CIRCLE('',#44922,12.);
#9266=CIRCLE('',#44923,0.4);
#9267=CIRCLE('',#44924,0.4);
#9268=CIRCLE('',#44925,12.);
#9269=CIRCLE('',#44926,0.4);
#9270=CIRCLE('',#44927,0.4);
#9271=CIRCLE('',#44928,12.);
#9272=CIRCLE('',#44929,0.4);
#9273=CIRCLE('',#44930,0.4);
#9274=CIRCLE('',#44931,12.);
#9275=CIRCLE('',#44932,0.4);
#9276=CIRCLE('',#44933,0.4);
#9277=CIRCLE('',#44934,12.);
#9278=CIRCLE('',#44935,0.4);
#9279=CIRCLE('',#44936,0.4);
#9280=CIRCLE('',#44937,12.);
#9281=CIRCLE('',#44939,0.4);
#9282=CIRCLE('',#44942,14.2343145750508);
#9283=CIRCLE('',#44943,14.2343145750508);
#9284=CIRCLE('',#44944,14.2343145750508);
#9285=CIRCLE('',#44945,12.);
#9286=CIRCLE('',#44946,0.4);
#9287=CIRCLE('',#44947,0.4);
#9288=CIRCLE('',#44948,12.);
#9289=CIRCLE('',#44949,0.4);
#9290=CIRCLE('',#44950,0.4);
#9291=CIRCLE('',#44951,12.);
#9292=CIRCLE('',#44952,0.4);
#9293=CIRCLE('',#44953,0.4);
#9294=CIRCLE('',#44954,12.);
#9295=CIRCLE('',#44955,0.4);
#9296=CIRCLE('',#44956,0.4);
#9297=CIRCLE('',#44957,12.);
#9298=CIRCLE('',#44958,0.4);
#9299=CIRCLE('',#44959,0.4);
#9300=CIRCLE('',#44960,12.);
#9301=CIRCLE('',#44961,0.4);
#9302=CIRCLE('',#44962,0.4);
#9303=CIRCLE('',#44963,12.);
#9304=CIRCLE('',#44964,0.4);
#9305=CIRCLE('',#44965,0.4);
#9306=CIRCLE('',#44966,12.);
#9307=CIRCLE('',#44967,0.4);
#9308=CIRCLE('',#44968,0.4);
#9309=CIRCLE('',#44969,12.);
#9310=CIRCLE('',#44970,0.4);
#9311=CIRCLE('',#44971,0.4);
#9312=CIRCLE('',#44972,12.);
#9313=CIRCLE('',#44973,0.4);
#9314=CIRCLE('',#44974,0.4);
#9315=CIRCLE('',#44975,12.);
#9316=CIRCLE('',#44976,0.4);
#9317=CIRCLE('',#44977,0.4);
#9318=CIRCLE('',#44978,12.);
#9319=CIRCLE('',#44979,0.4);
#9320=CIRCLE('',#44980,0.4);
#9321=CIRCLE('',#44981,12.);
#9322=CIRCLE('',#44982,0.4);
#9323=CIRCLE('',#44983,0.4);
#9324=CIRCLE('',#44984,12.);
#9325=CIRCLE('',#44985,0.4);
#9326=CIRCLE('',#44986,0.4);
#9327=CIRCLE('',#44987,12.);
#9328=CIRCLE('',#44988,0.4);
#9329=CIRCLE('',#44989,0.4);
#9330=CIRCLE('',#44990,12.);
#9331=CIRCLE('',#44991,0.4);
#9332=CIRCLE('',#44992,0.4);
#9333=CIRCLE('',#44993,12.);
#9334=CIRCLE('',#44994,0.4);
#9335=CIRCLE('',#44995,0.4);
#9336=CIRCLE('',#44996,12.);
#9337=CIRCLE('',#44997,0.4);
#9338=CIRCLE('',#44998,0.4);
#9339=CIRCLE('',#44999,12.);
#9340=CIRCLE('',#45000,0.4);
#9341=CIRCLE('',#45001,0.4);
#9342=CIRCLE('',#45002,12.);
#9343=CIRCLE('',#45003,0.4);
#9344=CIRCLE('',#45004,0.4);
#9345=CIRCLE('',#45005,12.);
#9346=CIRCLE('',#45006,0.4);
#9347=CIRCLE('',#45007,0.4);
#9348=CIRCLE('',#45008,12.);
#9349=CIRCLE('',#45009,0.4);
#9350=CIRCLE('',#45010,0.4);
#9351=CIRCLE('',#45011,12.);
#9352=CIRCLE('',#45012,0.4);
#9353=CIRCLE('',#45013,0.4);
#9354=CIRCLE('',#45014,12.);
#9355=CIRCLE('',#45069,14.8828427124746);
#9356=CIRCLE('',#45070,15.);
#9357=CIRCLE('',#45072,14.5171572875254);
#9358=CIRCLE('',#45084,15.);
#9359=CIRCLE('',#45085,14.8828427124746);
#9360=CIRCLE('',#45087,15.);
#9361=CIRCLE('',#45089,15.);
#9362=CIRCLE('',#45090,14.8828427124746);
#9363=CIRCLE('',#45097,14.8828427124746);
#9364=CIRCLE('',#45099,14.5171572875254);
#9365=CIRCLE('',#45101,14.8828427124746);
#9366=CIRCLE('',#45103,14.5171572875254);
#9367=CIRCLE('',#45105,0.399999999999991);
#9368=CIRCLE('',#45106,14.5171572875254);
#9369=CIRCLE('',#45107,0.400000000016502);
#9370=CIRCLE('',#45109,0.399999999999991);
#9371=CIRCLE('',#45110,14.5171572875254);
#9372=CIRCLE('',#45111,0.400000000016491);
#9373=CIRCLE('',#45113,0.399999999999991);
#9374=CIRCLE('',#45114,14.5171572875254);
#9375=CIRCLE('',#45115,0.400000000016493);
#9376=CIRCLE('',#45126,0.400000000016552);
#9377=CIRCLE('',#45127,0.399999999999991);
#9378=CIRCLE('',#45129,0.400000000016541);
#9379=CIRCLE('',#45130,0.399999999999991);
#9380=CIRCLE('',#45132,0.400000000016552);
#9381=CIRCLE('',#45133,0.399999999999991);
#10286=B_SPLINE_CURVE_WITH_KNOTS('',3,(#88387,#88388,#88389,#88390,#88391,
#88392,#88393),.UNSPECIFIED.,.F.,.F.,(4,3,4),(1.85983528421837,1.99900405382463,
2.00027269958661),.UNSPECIFIED.);
#10287=B_SPLINE_CURVE_WITH_KNOTS('',3,(#88395,#88396,#88397,#88398,#88399,
#88400),.UNSPECIFIED.,.F.,.F.,(4,2,4),(1.71839792902956,1.75157791747321,
1.85983528421837),.UNSPECIFIED.);
#10288=B_SPLINE_CURVE_WITH_KNOTS('',3,(#88402,#88403,#88404,#88405,#88406,
#88407),.UNSPECIFIED.,.F.,.F.,(4,2,4),(0.630914500179572,0.632798132766552,
0.718060933072034),.UNSPECIFIED.);
#10289=B_SPLINE_CURVE_WITH_KNOTS('',3,(#88409,#88410,#88411,#88412,#88413,
#88414),.UNSPECIFIED.,.F.,.F.,(4,2,4),(0.644405970934536,0.70175945659085,
1.03496766822937),.UNSPECIFIED.);
#10290=B_SPLINE_CURVE_WITH_KNOTS('',3,(#88418,#88419,#88420,#88421,#88422,
#88423),.UNSPECIFIED.,.F.,.F.,(4,2,4),(4.56099667124857,4.89420488288709,
4.95155836854339),.UNSPECIFIED.);
#10291=B_SPLINE_CURVE_WITH_KNOTS('',3,(#88425,#88426,#88427,#88428),
 .UNSPECIFIED.,.F.,.F.,(4,4),(0.,0.0866295070301289),.UNSPECIFIED.);
#10292=B_SPLINE_CURVE_WITH_KNOTS('',3,(#88430,#88431,#88432,#88433,#88434,
#88435),.UNSPECIFIED.,.F.,.F.,(4,2,4),(2.14071011495495,2.24896748170002,
2.28214747014369),.UNSPECIFIED.);
#10293=B_SPLINE_CURVE_WITH_KNOTS('',3,(#88437,#88438,#88439,#88440,#88441,
#88442,#88443),.UNSPECIFIED.,.F.,.F.,(4,3,4),(2.00027269958662,2.0015413175462,
2.14071011495495),.UNSPECIFIED.);
#10294=B_SPLINE_CURVE_WITH_KNOTS('',3,(#88445,#88446,#88447,#88448,#88449,
#88450,#88451),.UNSPECIFIED.,.F.,.F.,(4,3,4),(1.85983528421834,1.99900406518446,
2.00027269958662),.UNSPECIFIED.);
#10295=B_SPLINE_CURVE_WITH_KNOTS('',3,(#88453,#88454,#88455,#88456,#88457,
#88458),.UNSPECIFIED.,.F.,.F.,(4,2,4),(1.71839792902957,1.75157791747323,
1.85983528421834),.UNSPECIFIED.);
#10296=B_SPLINE_CURVE_WITH_KNOTS('',3,(#88460,#88461,#88462,#88463,#88464,
#88465),.UNSPECIFIED.,.F.,.F.,(4,2,4),(0.630914500166066,0.632798132753113,
0.718060933058547),.UNSPECIFIED.);
#10297=B_SPLINE_CURVE_WITH_KNOTS('',3,(#88467,#88468,#88469,#88470,#88471,
#88472),.UNSPECIFIED.,.F.,.F.,(4,2,4),(3.44238814067351,3.49974162632982,
3.83294983796833),.UNSPECIFIED.);
#10298=B_SPLINE_CURVE_WITH_KNOTS('',3,(#88476,#88477,#88478,#88479,#88480,
#88481),.UNSPECIFIED.,.F.,.F.,(4,2,4),(1.76301450150958,2.09622271314812,
2.15357619880444),.UNSPECIFIED.);
#10299=B_SPLINE_CURVE_WITH_KNOTS('',3,(#88483,#88484,#88485,#88486),
 .UNSPECIFIED.,.F.,.F.,(4,4),(0.,0.0866295070300163),.UNSPECIFIED.);
#10300=B_SPLINE_CURVE_WITH_KNOTS('',3,(#88488,#88489,#88490,#88491,#88492,
#88493),.UNSPECIFIED.,.F.,.F.,(4,2,4),(2.14071011495488,2.24896748170001,
2.28214747014365),.UNSPECIFIED.);
#10301=B_SPLINE_CURVE_WITH_KNOTS('',3,(#88494,#88495,#88496,#88497,#88498,
#88499,#88500),.UNSPECIFIED.,.F.,.F.,(4,3,4),(2.00027269958661,2.00154132906246,
2.14071011495488),.UNSPECIFIED.);
#10302=B_SPLINE_CURVE_WITH_KNOTS('',3,(#88504,#88505,#88506,#88507,#88508,
#88509,#88510,#88511,#88512,#88513),.UNSPECIFIED.,.F.,.F.,(4,2,2,2,4),(0.583234222022198,
0.585431861880819,0.649885567114863,0.734087500025299,0.810665904148401),
 .UNSPECIFIED.);
#10303=B_SPLINE_CURVE_WITH_KNOTS('',3,(#88516,#88517,#88518,#88519,#88520,
#88521,#88522,#88523),.UNSPECIFIED.,.F.,.F.,(4,2,2,4),(0.,0.111246430521639,
0.182410640433451,0.207305864120085),.UNSPECIFIED.);
#10304=B_SPLINE_CURVE_WITH_KNOTS('',3,(#88528,#88529,#88530,#88531,#88532,
#88533,#88534,#88535,#88536,#88537),.UNSPECIFIED.,.F.,.F.,(4,2,2,2,4),(0.583234221969361,
0.585431861828122,0.649885567064887,0.734087499976625,0.810665904099694),
 .UNSPECIFIED.);
#10305=B_SPLINE_CURVE_WITH_KNOTS('',3,(#88540,#88541,#88542,#88543,#88544,
#88545,#88546,#88547),.UNSPECIFIED.,.F.,.F.,(4,2,2,4),(0.,0.111246430522183,
0.182410640434968,0.207305864122133),.UNSPECIFIED.);
#10306=B_SPLINE_CURVE_WITH_KNOTS('',3,(#88554,#88555,#88556,#88557,#88558,
#88559),.UNSPECIFIED.,.F.,.F.,(4,2,4),(0.626226208466124,0.628605257115929,
0.713361672035043),.UNSPECIFIED.);
#10307=B_SPLINE_CURVE_WITH_KNOTS('',3,(#88565,#88566,#88567,#88568,#88569,
#88570),.UNSPECIFIED.,.F.,.F.,(4,2,4),(1.76301450150958,2.09622271314812,
2.15357619880443),.UNSPECIFIED.);
#10308=B_SPLINE_CURVE_WITH_KNOTS('',3,(#88572,#88573,#88574,#88575,#88576,
#88577,#88578,#88579),.UNSPECIFIED.,.F.,.F.,(4,2,2,4),(0.,0.111246430523028,
0.182410640437555,0.20730586412578),.UNSPECIFIED.);
#10309=B_SPLINE_CURVE_WITH_KNOTS('',3,(#88583,#88584,#88585,#88586,#88587,
#88588,#88589,#88590,#88591,#88592),.UNSPECIFIED.,.F.,.F.,(4,2,2,2,4),(0.583234221969814,
0.585431861828592,0.64988556706566,0.734087499977432,0.810665904100495),
 .UNSPECIFIED.);
#10310=B_SPLINE_CURVE_WITH_KNOTS('',3,(#88593,#88594,#88595,#88596,#88597,
#88598),.UNSPECIFIED.,.F.,.F.,(4,2,4),(3.44238814067351,3.49974162632982,
3.83294983796834),.UNSPECIFIED.);
#10311=B_SPLINE_CURVE_WITH_KNOTS('',3,(#88609,#88610,#88611,#88612,#88613,
#88614,#88615),.UNSPECIFIED.,.F.,.F.,(4,3,4),(2.61858533223862,2.75775410184484,
2.75902274760691),.UNSPECIFIED.);
#10312=B_SPLINE_CURVE_WITH_KNOTS('',3,(#88617,#88618,#88619,#88620,#88621,
#88622),.UNSPECIFIED.,.F.,.F.,(4,2,4),(2.47714797704988,2.51032796549351,
2.61858533223862),.UNSPECIFIED.);
#10313=B_SPLINE_CURVE_WITH_KNOTS('',3,(#88624,#88625,#88626,#88627,#88628,
#88629),.UNSPECIFIED.,.F.,.F.,(4,2,4),(0.669395998132427,0.670313715959972,
0.756562801675098),.UNSPECIFIED.);
#10314=B_SPLINE_CURVE_WITH_KNOTS('',3,(#88631,#88632,#88633,#88634,#88635,
#88636),.UNSPECIFIED.,.F.,.F.,(4,2,4),(0.644405970934543,0.70175945659085,
1.03496766822938),.UNSPECIFIED.);
#10315=B_SPLINE_CURVE_WITH_KNOTS('',3,(#88640,#88641,#88642,#88643,#88644,
#88645),.UNSPECIFIED.,.F.,.F.,(4,2,4),(4.56099667124858,4.89420488288709,
4.95155836854339),.UNSPECIFIED.);
#10316=B_SPLINE_CURVE_WITH_KNOTS('',3,(#88647,#88648,#88649,#88650),
 .UNSPECIFIED.,.F.,.F.,(4,4),(0.,0.0866134072258944),.UNSPECIFIED.);
#10317=B_SPLINE_CURVE_WITH_KNOTS('',3,(#88652,#88653,#88654,#88655,#88656,
#88657),.UNSPECIFIED.,.F.,.F.,(4,2,4),(2.8994601629752,3.00771752972032,
3.04089751816399),.UNSPECIFIED.);
#10318=B_SPLINE_CURVE_WITH_KNOTS('',3,(#88659,#88660,#88661,#88662,#88663,
#88664,#88665),.UNSPECIFIED.,.F.,.F.,(4,3,4),(2.75902274760692,2.76029136556641,
2.8994601629752),.UNSPECIFIED.);
#10319=B_SPLINE_CURVE_WITH_KNOTS('',3,(#88667,#88668,#88669,#88670,#88671,
#88672,#88673),.UNSPECIFIED.,.F.,.F.,(4,3,4),(2.61858533223864,2.75775411320476,
2.75902274760692),.UNSPECIFIED.);
#10320=B_SPLINE_CURVE_WITH_KNOTS('',3,(#88674,#88675,#88676,#88677,#88678,
#88679),.UNSPECIFIED.,.F.,.F.,(4,2,4),(2.47714797704987,2.51032796549352,
2.61858533223864),.UNSPECIFIED.);
#10321=B_SPLINE_CURVE_WITH_KNOTS('',3,(#88682,#88683,#88684,#88685),
 .UNSPECIFIED.,.F.,.F.,(4,4),(0.,0.0866364281750408),.UNSPECIFIED.);
#10322=B_SPLINE_CURVE_WITH_KNOTS('',3,(#88687,#88688,#88689,#88690,#88691,
#88692),.UNSPECIFIED.,.F.,.F.,(4,2,4),(2.89946016297517,3.00771752972031,
3.04089751816395),.UNSPECIFIED.);
#10323=B_SPLINE_CURVE_WITH_KNOTS('',3,(#88693,#88694,#88695,#88696,#88697,
#88698,#88699),.UNSPECIFIED.,.F.,.F.,(4,3,4),(2.75902274760691,2.76029137708275,
2.89946016297517),.UNSPECIFIED.);
#10324=B_SPLINE_CURVE_WITH_KNOTS('',3,(#88706,#88707,#88708,#88709,#88710,
#88711,#88712,#88713,#88714,#88715),.UNSPECIFIED.,.F.,.F.,(4,2,2,2,4),(0.5832342220102,
0.585431861868939,0.649885567105413,0.734087500016793,0.810665904139813),
 .UNSPECIFIED.);
#10325=B_SPLINE_CURVE_WITH_KNOTS('',3,(#88718,#88719,#88720,#88721,#88722,
#88723,#88724,#88725),.UNSPECIFIED.,.F.,.F.,(4,2,2,4),(0.,0.111246430521943,
0.182410640434217,0.207305864121051),.UNSPECIFIED.);
#10326=B_SPLINE_CURVE_WITH_KNOTS('',3,(#88740,#88741,#88742,#88743,#88744,
#88745,#88746),.UNSPECIFIED.,.F.,.F.,(4,3,4),(2.61858533223868,2.7577545751336,
2.75902274760691),.UNSPECIFIED.);
#10327=B_SPLINE_CURVE_WITH_KNOTS('',3,(#88748,#88749,#88750,#88751,#88752,
#88753),.UNSPECIFIED.,.F.,.F.,(4,2,4),(2.47714797704988,2.51032796549352,
2.61858533223868),.UNSPECIFIED.);
#10328=B_SPLINE_CURVE_WITH_KNOTS('',3,(#88755,#88756,#88757,#88758,#88759,
#88760),.UNSPECIFIED.,.F.,.F.,(4,2,4),(0.626226208455071,0.628605257104885,
0.713361672024136),.UNSPECIFIED.);
#10329=B_SPLINE_CURVE_WITH_KNOTS('',3,(#88762,#88763,#88764,#88765,#88766,
#88767),.UNSPECIFIED.,.F.,.F.,(4,2,4),(0.644405970934541,0.701759456590849,
1.03496766822939),.UNSPECIFIED.);
#10330=B_SPLINE_CURVE_WITH_KNOTS('',3,(#88771,#88772,#88773,#88774,#88775,
#88776),.UNSPECIFIED.,.F.,.F.,(4,2,4),(-1.03496766822936,-0.70175945659085,
-0.644405970934541),.UNSPECIFIED.);
#10331=B_SPLINE_CURVE_WITH_KNOTS('',3,(#88778,#88779,#88780,#88781),
 .UNSPECIFIED.,.F.,.F.,(4,4),(0.,0.0866364281738437),.UNSPECIFIED.);
#10332=B_SPLINE_CURVE_WITH_KNOTS('',3,(#88783,#88784,#88785,#88786,#88787,
#88788),.UNSPECIFIED.,.F.,.F.,(4,2,4),(2.8994601629752,3.00771752972032,
3.04089751816397),.UNSPECIFIED.);
#10333=B_SPLINE_CURVE_WITH_KNOTS('',3,(#88790,#88791,#88792,#88793,#88794,
#88795,#88796),.UNSPECIFIED.,.F.,.F.,(4,3,4),(2.75902274760692,2.7602913655664,
2.8994601629752),.UNSPECIFIED.);
#10334=B_SPLINE_CURVE_WITH_KNOTS('',3,(#88798,#88799,#88800,#88801,#88802,
#88803,#88804),.UNSPECIFIED.,.F.,.F.,(4,3,4),(2.61858533223864,2.75775411320475,
2.75902274760692),.UNSPECIFIED.);
#10335=B_SPLINE_CURVE_WITH_KNOTS('',3,(#88806,#88807,#88808,#88809,#88810,
#88811),.UNSPECIFIED.,.F.,.F.,(4,2,4),(2.47714797704986,2.51032796549352,
2.61858533223864),.UNSPECIFIED.);
#10336=B_SPLINE_CURVE_WITH_KNOTS('',3,(#88813,#88814,#88815,#88816,#88817,
#88818),.UNSPECIFIED.,.F.,.F.,(4,2,4),(0.669395998120173,0.670313715947721,
0.756562801662947),.UNSPECIFIED.);
#10337=B_SPLINE_CURVE_WITH_KNOTS('',3,(#88820,#88821,#88822,#88823,#88824,
#88825),.UNSPECIFIED.,.F.,.F.,(4,2,4),(-2.15357620101586,-2.09622271314812,
-1.7630145015096),.UNSPECIFIED.);
#10338=B_SPLINE_CURVE_WITH_KNOTS('',3,(#88829,#88830,#88831,#88832,#88833,
#88834),.UNSPECIFIED.,.F.,.F.,(4,2,4),(1.76301450150958,2.09622271314812,
2.15357619880443),.UNSPECIFIED.);
#10339=B_SPLINE_CURVE_WITH_KNOTS('',3,(#88836,#88837,#88838,#88839),
 .UNSPECIFIED.,.F.,.F.,(4,4),(0.,0.0866134072248542),.UNSPECIFIED.);
#10340=B_SPLINE_CURVE_WITH_KNOTS('',3,(#88841,#88842,#88843,#88844,#88845,
#88846),.UNSPECIFIED.,.F.,.F.,(4,2,4),(2.89946016297518,3.00771752972031,
3.04089751816395),.UNSPECIFIED.);
#10341=B_SPLINE_CURVE_WITH_KNOTS('',3,(#88847,#88848,#88849,#88850,#88851,
#88852,#88853),.UNSPECIFIED.,.F.,.F.,(4,3,4),(2.75902274760691,2.76029137708276,
2.89946016297518),.UNSPECIFIED.);
#10342=B_SPLINE_CURVE_WITH_KNOTS('',3,(#88857,#88858,#88859,#88860,#88861,
#88862,#88863,#88864,#88865,#88866),.UNSPECIFIED.,.F.,.F.,(4,2,2,2,4),(0.583234221992704,
0.58543186185144,0.649885567087875,0.734087499999534,0.810665904122571),
 .UNSPECIFIED.);
#10343=B_SPLINE_CURVE_WITH_KNOTS('',3,(#88869,#88870,#88871,#88872,#88873,
#88874,#88875,#88876),.UNSPECIFIED.,.F.,.F.,(4,2,2,4),(0.,0.111246430522522,
0.182410640435861,0.207305864123323),.UNSPECIFIED.);
#10344=B_SPLINE_CURVE_WITH_KNOTS('',3,(#88881,#88882,#88883,#88884,#88885,
#88886,#88887,#88888,#88889,#88890),.UNSPECIFIED.,.F.,.F.,(4,2,2,2,4),(0.583234221991165,
0.585431861849779,0.649885567085203,0.734087499996366,0.810665904119391),
 .UNSPECIFIED.);
#10345=B_SPLINE_CURVE_WITH_KNOTS('',3,(#88893,#88894,#88895,#88896,#88897,
#88898,#88899,#88900),.UNSPECIFIED.,.F.,.F.,(4,2,2,4),(0.,0.111246430522045,
0.182410640434902,0.207305864122096),.UNSPECIFIED.);
#10346=B_SPLINE_CURVE_WITH_KNOTS('',3,(#88920,#88921,#88922,#88923,#88924,
#88925),.UNSPECIFIED.,.F.,.F.,(4,2,4),(0.196228296217563,0.338813557833421,
0.340113319180875),.UNSPECIFIED.);
#10347=B_SPLINE_CURVE_WITH_KNOTS('',3,(#88928,#88929,#88930,#88931,#88932,
#88933),.UNSPECIFIED.,.F.,.F.,(4,2,4),(-0.00129977819395621,0.,0.142585244788061),
 .UNSPECIFIED.);
#10348=B_SPLINE_CURVE_WITH_KNOTS('',3,(#88935,#88936,#88937,#88938,#88939,
#88940),.UNSPECIFIED.,.F.,.F.,(4,2,4),(0.196228296217555,0.338813557833423,
0.340113319180884),.UNSPECIFIED.);
#10349=B_SPLINE_CURVE_WITH_KNOTS('',3,(#88943,#88944,#88945,#88946,#88947,
#88948),.UNSPECIFIED.,.F.,.F.,(4,2,4),(-0.00129977819395902,0.,0.14258524478806),
 .UNSPECIFIED.);
#10350=B_SPLINE_CURVE_WITH_KNOTS('',3,(#88950,#88951,#88952,#88953,#88954,
#88955),.UNSPECIFIED.,.F.,.F.,(4,2,4),(0.196228296217518,0.338813557833289,
0.340113319180834),.UNSPECIFIED.);
#10351=B_SPLINE_CURVE_WITH_KNOTS('',3,(#88958,#88959,#88960,#88961,#88962,
#88963),.UNSPECIFIED.,.F.,.F.,(4,2,4),(-0.0012997781939584,0.,0.142585244788068),
 .UNSPECIFIED.);
#10352=B_SPLINE_CURVE_WITH_KNOTS('',3,(#89259,#89260,#89261,#89262,#89263,
#89264),.UNSPECIFIED.,.F.,.F.,(4,2,4),(0.196228351995834,0.338813601825616,
0.340113374972261),.UNSPECIFIED.);
#10353=B_SPLINE_CURVE_WITH_KNOTS('',3,(#89267,#89268,#89269,#89270,#89271,
#89272),.UNSPECIFIED.,.F.,.F.,(4,2,4),(-0.00129978983284723,0.,0.142585233162046),
 .UNSPECIFIED.);
#10354=B_SPLINE_CURVE_WITH_KNOTS('',3,(#89274,#89275,#89276,#89277,#89278,
#89279),.UNSPECIFIED.,.F.,.F.,(4,2,4),(0.19622835199583,0.338813601825611,
0.340113374972257),.UNSPECIFIED.);
#10355=B_SPLINE_CURVE_WITH_KNOTS('',3,(#89282,#89283,#89284,#89285,#89286,
#89287),.UNSPECIFIED.,.F.,.F.,(4,2,4),(-0.00129978983276234,0.,0.142585233162139),
 .UNSPECIFIED.);
#10356=B_SPLINE_CURVE_WITH_KNOTS('',3,(#89289,#89290,#89291,#89292,#89293,
#89294),.UNSPECIFIED.,.F.,.F.,(4,2,4),(0.196228351995831,0.338813601825613,
0.340113374972263),.UNSPECIFIED.);
#10357=B_SPLINE_CURVE_WITH_KNOTS('',3,(#89297,#89298,#89299,#89300,#89301,
#89302),.UNSPECIFIED.,.F.,.F.,(4,2,4),(-0.00129978983275812,0.,0.142638931811887),
 .UNSPECIFIED.);
#12543=LINE('',#88385,#15037);
#12544=LINE('',#88525,#15038);
#12545=LINE('',#88549,#15039);
#12546=LINE('',#88581,#15040);
#12547=LINE('',#88607,#15041);
#12548=LINE('',#88727,#15042);
#12549=LINE('',#88738,#15043);
#12550=LINE('',#88878,#15044);
#12551=LINE('',#88902,#15045);
#12552=LINE('',#88908,#15046);
#12553=LINE('',#88911,#15047);
#12554=LINE('',#88914,#15048);
#12555=LINE('',#88916,#15049);
#12556=LINE('',#88917,#15050);
#12557=LINE('',#88965,#15051);
#12558=LINE('',#88969,#15052);
#12559=LINE('',#88973,#15053);
#12560=LINE('',#88977,#15054);
#12561=LINE('',#88981,#15055);
#12562=LINE('',#88985,#15056);
#12563=LINE('',#88989,#15057);
#12564=LINE('',#88993,#15058);
#12565=LINE('',#88997,#15059);
#12566=LINE('',#89001,#15060);
#12567=LINE('',#89005,#15061);
#12568=LINE('',#89009,#15062);
#12569=LINE('',#89013,#15063);
#12570=LINE('',#89017,#15064);
#12571=LINE('',#89021,#15065);
#12572=LINE('',#89025,#15066);
#12573=LINE('',#89029,#15067);
#12574=LINE('',#89033,#15068);
#12575=LINE('',#89037,#15069);
#12576=LINE('',#89041,#15070);
#12577=LINE('',#89045,#15071);
#12578=LINE('',#89049,#15072);
#12579=LINE('',#89053,#15073);
#12580=LINE('',#89057,#15074);
#12581=LINE('',#89061,#15075);
#12582=LINE('',#89065,#15076);
#12583=LINE('',#89069,#15077);
#12584=LINE('',#89073,#15078);
#12585=LINE('',#89077,#15079);
#12586=LINE('',#89081,#15080);
#12587=LINE('',#89085,#15081);
#12588=LINE('',#89089,#15082);
#12589=LINE('',#89093,#15083);
#12590=LINE('',#89097,#15084);
#12591=LINE('',#89101,#15085);
#12592=LINE('',#89105,#15086);
#12593=LINE('',#89109,#15087);
#12594=LINE('',#89113,#15088);
#12595=LINE('',#89117,#15089);
#12596=LINE('',#89121,#15090);
#12597=LINE('',#89125,#15091);
#12598=LINE('',#89129,#15092);
#12599=LINE('',#89133,#15093);
#12600=LINE('',#89137,#15094);
#12601=LINE('',#89141,#15095);
#12602=LINE('',#89145,#15096);
#12603=LINE('',#89149,#15097);
#12604=LINE('',#89153,#15098);
#12605=LINE('',#89157,#15099);
#12606=LINE('',#89161,#15100);
#12607=LINE('',#89165,#15101);
#12608=LINE('',#89169,#15102);
#12609=LINE('',#89173,#15103);
#12610=LINE('',#89177,#15104);
#12611=LINE('',#89181,#15105);
#12612=LINE('',#89185,#15106);
#12613=LINE('',#89189,#15107);
#12614=LINE('',#89193,#15108);
#12615=LINE('',#89197,#15109);
#12616=LINE('',#89201,#15110);
#12617=LINE('',#89205,#15111);
#12618=LINE('',#89209,#15112);
#12619=LINE('',#89213,#15113);
#12620=LINE('',#89217,#15114);
#12621=LINE('',#89221,#15115);
#12622=LINE('',#89225,#15116);
#12623=LINE('',#89229,#15117);
#12624=LINE('',#89233,#15118);
#12625=LINE('',#89237,#15119);
#12626=LINE('',#89241,#15120);
#12627=LINE('',#89245,#15121);
#12628=LINE('',#89249,#15122);
#12629=LINE('',#89252,#15123);
#12630=LINE('',#89255,#15124);
#12631=LINE('',#89256,#15125);
#12632=LINE('',#89306,#15126);
#12633=LINE('',#89310,#15127);
#12634=LINE('',#89314,#15128);
#12635=LINE('',#89318,#15129);
#12636=LINE('',#89322,#15130);
#12637=LINE('',#89326,#15131);
#12638=LINE('',#89330,#15132);
#12639=LINE('',#89334,#15133);
#12640=LINE('',#89338,#15134);
#12641=LINE('',#89342,#15135);
#12642=LINE('',#89346,#15136);
#12643=LINE('',#89350,#15137);
#12644=LINE('',#89354,#15138);
#12645=LINE('',#89358,#15139);
#12646=LINE('',#89362,#15140);
#12647=LINE('',#89366,#15141);
#12648=LINE('',#89370,#15142);
#12649=LINE('',#89374,#15143);
#12650=LINE('',#89378,#15144);
#12651=LINE('',#89382,#15145);
#12652=LINE('',#89386,#15146);
#12653=LINE('',#89390,#15147);
#12654=LINE('',#89394,#15148);
#12655=LINE('',#89398,#15149);
#12656=LINE('',#89402,#15150);
#12657=LINE('',#89406,#15151);
#12658=LINE('',#89410,#15152);
#12659=LINE('',#89414,#15153);
#12660=LINE('',#89418,#15154);
#12661=LINE('',#89422,#15155);
#12662=LINE('',#89426,#15156);
#12663=LINE('',#89430,#15157);
#12664=LINE('',#89434,#15158);
#12665=LINE('',#89438,#15159);
#12666=LINE('',#89442,#15160);
#12667=LINE('',#89446,#15161);
#12668=LINE('',#89450,#15162);
#12669=LINE('',#89454,#15163);
#12670=LINE('',#89458,#15164);
#12671=LINE('',#89462,#15165);
#12672=LINE('',#89466,#15166);
#12673=LINE('',#89470,#15167);
#12674=LINE('',#89474,#15168);
#12675=LINE('',#89478,#15169);
#12676=LINE('',#89482,#15170);
#12677=LINE('',#89486,#15171);
#12678=LINE('',#89490,#15172);
#12679=LINE('',#89494,#15173);
#12680=LINE('',#89498,#15174);
#12681=LINE('',#89502,#15175);
#12682=LINE('',#89506,#15176);
#12683=LINE('',#89510,#15177);
#12684=LINE('',#89514,#15178);
#12685=LINE('',#89518,#15179);
#12686=LINE('',#89522,#15180);
#12687=LINE('',#89526,#15181);
#12688=LINE('',#89530,#15182);
#12689=LINE('',#89534,#15183);
#12690=LINE('',#89538,#15184);
#12691=LINE('',#89542,#15185);
#12692=LINE('',#89546,#15186);
#12693=LINE('',#89550,#15187);
#12694=LINE('',#89554,#15188);
#12695=LINE('',#89558,#15189);
#12696=LINE('',#89562,#15190);
#12697=LINE('',#89566,#15191);
#12698=LINE('',#89570,#15192);
#12699=LINE('',#89574,#15193);
#12700=LINE('',#89578,#15194);
#12701=LINE('',#89580,#15195);
#12702=LINE('',#89582,#15196);
#12703=LINE('',#89583,#15197);
#12704=LINE('',#89585,#15198);
#12705=LINE('',#89587,#15199);
#12706=LINE('',#89589,#15200);
#12707=LINE('',#89590,#15201);
#12708=LINE('',#89592,#15202);
#12709=LINE('',#89594,#15203);
#12710=LINE('',#89595,#15204);
#12711=LINE('',#89597,#15205);
#12712=LINE('',#89599,#15206);
#12713=LINE('',#89600,#15207);
#12714=LINE('',#89602,#15208);
#12715=LINE('',#89604,#15209);
#12716=LINE('',#89606,#15210);
#12717=LINE('',#89607,#15211);
#12718=LINE('',#89609,#15212);
#12719=LINE('',#89611,#15213);
#12720=LINE('',#89613,#15214);
#12721=LINE('',#89614,#15215);
#12722=LINE('',#89616,#15216);
#12723=LINE('',#89618,#15217);
#12724=LINE('',#89619,#15218);
#12725=LINE('',#89621,#15219);
#12726=LINE('',#89623,#15220);
#12727=LINE('',#89624,#15221);
#12728=LINE('',#89626,#15222);
#12729=LINE('',#89628,#15223);
#12730=LINE('',#89630,#15224);
#12731=LINE('',#89631,#15225);
#12732=LINE('',#89633,#15226);
#12733=LINE('',#89635,#15227);
#12734=LINE('',#89637,#15228);
#12735=LINE('',#89638,#15229);
#12736=LINE('',#89640,#15230);
#12737=LINE('',#89642,#15231);
#12738=LINE('',#89643,#15232);
#12739=LINE('',#89645,#15233);
#12740=LINE('',#89647,#15234);
#12741=LINE('',#89648,#15235);
#12742=LINE('',#89650,#15236);
#12743=LINE('',#89652,#15237);
#12744=LINE('',#89654,#15238);
#12745=LINE('',#89655,#15239);
#12746=LINE('',#89657,#15240);
#12747=LINE('',#89659,#15241);
#12748=LINE('',#89661,#15242);
#12749=LINE('',#89662,#15243);
#12750=LINE('',#89664,#15244);
#12751=LINE('',#89666,#15245);
#12752=LINE('',#89667,#15246);
#12753=LINE('',#89669,#15247);
#12754=LINE('',#89671,#15248);
#12755=LINE('',#89672,#15249);
#12756=LINE('',#89674,#15250);
#12757=LINE('',#89676,#15251);
#12758=LINE('',#89678,#15252);
#12759=LINE('',#89679,#15253);
#12760=LINE('',#89681,#15254);
#12761=LINE('',#89683,#15255);
#12762=LINE('',#89685,#15256);
#12763=LINE('',#89686,#15257);
#12764=LINE('',#89688,#15258);
#12765=LINE('',#89690,#15259);
#12766=LINE('',#89691,#15260);
#12767=LINE('',#89693,#15261);
#12768=LINE('',#89695,#15262);
#12769=LINE('',#89696,#15263);
#12770=LINE('',#89698,#15264);
#12771=LINE('',#89700,#15265);
#12772=LINE('',#89702,#15266);
#12773=LINE('',#89703,#15267);
#12774=LINE('',#89705,#15268);
#12775=LINE('',#89707,#15269);
#12776=LINE('',#89714,#15270);
#12777=LINE('',#89715,#15271);
#12778=LINE('',#89717,#15272);
#12779=LINE('',#89719,#15273);
#12780=LINE('',#89720,#15274);
#12781=LINE('',#89722,#15275);
#12782=LINE('',#89724,#15276);
#12783=LINE('',#89725,#15277);
#12784=LINE('',#89727,#15278);
#12785=LINE('',#89729,#15279);
#12786=LINE('',#89731,#15280);
#12787=LINE('',#89732,#15281);
#12788=LINE('',#89734,#15282);
#12789=LINE('',#89736,#15283);
#12790=LINE('',#89747,#15284);
#12791=LINE('',#89748,#15285);
#12792=LINE('',#89750,#15286);
#12793=LINE('',#89752,#15287);
#12794=LINE('',#89753,#15288);
#12795=LINE('',#89755,#15289);
#12796=LINE('',#89923,#15290);
#12797=LINE('',#89924,#15291);
#12798=LINE('',#89926,#15292);
#12799=LINE('',#89928,#15293);
#12800=LINE('',#89930,#15294);
#12801=LINE('',#89931,#15295);
#12802=LINE('',#89933,#15296);
#12803=LINE('',#89935,#15297);
#12804=LINE('',#89936,#15298);
#12805=LINE('',#89938,#15299);
#12806=LINE('',#90093,#15300);
#12807=LINE('',#90094,#15301);
#12808=LINE('',#90096,#15302);
#12809=LINE('',#90098,#15303);
#12810=LINE('',#90100,#15304);
#12811=LINE('',#90102,#15305);
#12812=LINE('',#90107,#15306);
#12813=LINE('',#90109,#15307);
#12814=LINE('',#90114,#15308);
#12815=LINE('',#90116,#15309);
#12816=LINE('',#90119,#15310);
#12817=LINE('',#90121,#15311);
#12818=LINE('',#90126,#15312);
#12819=LINE('',#90128,#15313);
#12820=LINE('',#90131,#15314);
#12821=LINE('',#90133,#15315);
#12822=LINE('',#90138,#15316);
#12823=LINE('',#90140,#15317);
#12824=LINE('',#90143,#15318);
#12825=LINE('',#90145,#15319);
#12826=LINE('',#90150,#15320);
#12827=LINE('',#90152,#15321);
#12828=LINE('',#90155,#15322);
#12829=LINE('',#90157,#15323);
#12830=LINE('',#90162,#15324);
#12831=LINE('',#90164,#15325);
#12832=LINE('',#90167,#15326);
#12833=LINE('',#90169,#15327);
#12834=LINE('',#90174,#15328);
#12835=LINE('',#90176,#15329);
#12836=LINE('',#90179,#15330);
#12837=LINE('',#90181,#15331);
#12838=LINE('',#90186,#15332);
#12839=LINE('',#90188,#15333);
#15037=VECTOR('',#56013,8.99999999999999);
#15038=VECTOR('',#56026,10.);
#15039=VECTOR('',#56033,10.);
#15040=VECTOR('',#56044,10.);
#15041=VECTOR('',#56055,8.99999999999999);
#15042=VECTOR('',#56074,10.);
#15043=VECTOR('',#56087,8.99999999999999);
#15044=VECTOR('',#56100,10.);
#15045=VECTOR('',#56107,10.);
#15046=VECTOR('',#56112,10.);
#15047=VECTOR('',#56115,10.);
#15048=VECTOR('',#56118,10.);
#15049=VECTOR('',#56119,10.);
#15050=VECTOR('',#56120,10.);
#15051=VECTOR('',#56129,10.);
#15052=VECTOR('',#56132,10.);
#15053=VECTOR('',#56135,10.);
#15054=VECTOR('',#56138,10.);
#15055=VECTOR('',#56141,10.);
#15056=VECTOR('',#56144,10.);
#15057=VECTOR('',#56147,10.);
#15058=VECTOR('',#56150,10.);
#15059=VECTOR('',#56153,10.);
#15060=VECTOR('',#56156,10.);
#15061=VECTOR('',#56159,10.);
#15062=VECTOR('',#56162,10.);
#15063=VECTOR('',#56165,10.);
#15064=VECTOR('',#56168,10.);
#15065=VECTOR('',#56171,10.);
#15066=VECTOR('',#56174,10.);
#15067=VECTOR('',#56177,10.);
#15068=VECTOR('',#56180,10.);
#15069=VECTOR('',#56183,10.);
#15070=VECTOR('',#56186,10.);
#15071=VECTOR('',#56189,10.);
#15072=VECTOR('',#56192,10.);
#15073=VECTOR('',#56195,10.);
#15074=VECTOR('',#56198,10.);
#15075=VECTOR('',#56201,10.);
#15076=VECTOR('',#56204,10.);
#15077=VECTOR('',#56207,10.);
#15078=VECTOR('',#56210,10.);
#15079=VECTOR('',#56213,10.);
#15080=VECTOR('',#56216,10.);
#15081=VECTOR('',#56219,10.);
#15082=VECTOR('',#56222,10.);
#15083=VECTOR('',#56225,10.);
#15084=VECTOR('',#56228,10.);
#15085=VECTOR('',#56231,10.);
#15086=VECTOR('',#56234,10.);
#15087=VECTOR('',#56237,10.);
#15088=VECTOR('',#56240,10.);
#15089=VECTOR('',#56243,10.);
#15090=VECTOR('',#56246,10.);
#15091=VECTOR('',#56249,10.);
#15092=VECTOR('',#56252,10.);
#15093=VECTOR('',#56255,10.);
#15094=VECTOR('',#56258,10.);
#15095=VECTOR('',#56261,10.);
#15096=VECTOR('',#56264,10.);
#15097=VECTOR('',#56267,10.);
#15098=VECTOR('',#56270,10.);
#15099=VECTOR('',#56273,10.);
#15100=VECTOR('',#56276,10.);
#15101=VECTOR('',#56279,10.);
#15102=VECTOR('',#56282,10.);
#15103=VECTOR('',#56285,10.);
#15104=VECTOR('',#56288,10.);
#15105=VECTOR('',#56291,10.);
#15106=VECTOR('',#56294,10.);
#15107=VECTOR('',#56297,10.);
#15108=VECTOR('',#56300,10.);
#15109=VECTOR('',#56303,10.);
#15110=VECTOR('',#56306,10.);
#15111=VECTOR('',#56309,10.);
#15112=VECTOR('',#56312,10.);
#15113=VECTOR('',#56315,10.);
#15114=VECTOR('',#56318,10.);
#15115=VECTOR('',#56321,10.);
#15116=VECTOR('',#56324,10.);
#15117=VECTOR('',#56327,10.);
#15118=VECTOR('',#56330,10.);
#15119=VECTOR('',#56333,10.);
#15120=VECTOR('',#56336,10.);
#15121=VECTOR('',#56339,10.);
#15122=VECTOR('',#56344,10.);
#15123=VECTOR('',#56347,10.);
#15124=VECTOR('',#56350,10.);
#15125=VECTOR('',#56351,10.);
#15126=VECTOR('',#56362,10.);
#15127=VECTOR('',#56365,10.);
#15128=VECTOR('',#56368,10.);
#15129=VECTOR('',#56371,10.);
#15130=VECTOR('',#56374,10.);
#15131=VECTOR('',#56377,10.);
#15132=VECTOR('',#56380,10.);
#15133=VECTOR('',#56383,10.);
#15134=VECTOR('',#56386,10.);
#15135=VECTOR('',#56389,10.);
#15136=VECTOR('',#56392,10.);
#15137=VECTOR('',#56395,10.);
#15138=VECTOR('',#56398,10.);
#15139=VECTOR('',#56401,10.);
#15140=VECTOR('',#56404,10.);
#15141=VECTOR('',#56407,10.);
#15142=VECTOR('',#56410,10.);
#15143=VECTOR('',#56413,10.);
#15144=VECTOR('',#56416,10.);
#15145=VECTOR('',#56419,10.);
#15146=VECTOR('',#56422,10.);
#15147=VECTOR('',#56425,10.);
#15148=VECTOR('',#56428,10.);
#15149=VECTOR('',#56431,10.);
#15150=VECTOR('',#56434,10.);
#15151=VECTOR('',#56437,10.);
#15152=VECTOR('',#56440,10.);
#15153=VECTOR('',#56443,10.);
#15154=VECTOR('',#56446,10.);
#15155=VECTOR('',#56449,10.);
#15156=VECTOR('',#56452,10.);
#15157=VECTOR('',#56455,10.);
#15158=VECTOR('',#56458,10.);
#15159=VECTOR('',#56461,10.);
#15160=VECTOR('',#56464,10.);
#15161=VECTOR('',#56467,10.);
#15162=VECTOR('',#56470,10.);
#15163=VECTOR('',#56473,10.);
#15164=VECTOR('',#56476,10.);
#15165=VECTOR('',#56479,10.);
#15166=VECTOR('',#56482,10.);
#15167=VECTOR('',#56485,10.);
#15168=VECTOR('',#56488,10.);
#15169=VECTOR('',#56491,10.);
#15170=VECTOR('',#56494,10.);
#15171=VECTOR('',#56497,10.);
#15172=VECTOR('',#56500,10.);
#15173=VECTOR('',#56503,10.);
#15174=VECTOR('',#56506,10.);
#15175=VECTOR('',#56509,10.);
#15176=VECTOR('',#56512,10.);
#15177=VECTOR('',#56515,10.);
#15178=VECTOR('',#56518,10.);
#15179=VECTOR('',#56521,10.);
#15180=VECTOR('',#56524,10.);
#15181=VECTOR('',#56527,10.);
#15182=VECTOR('',#56530,10.);
#15183=VECTOR('',#56533,10.);
#15184=VECTOR('',#56536,10.);
#15185=VECTOR('',#56539,10.);
#15186=VECTOR('',#56542,10.);
#15187=VECTOR('',#56545,10.);
#15188=VECTOR('',#56548,10.);
#15189=VECTOR('',#56551,10.);
#15190=VECTOR('',#56554,10.);
#15191=VECTOR('',#56557,10.);
#15192=VECTOR('',#56560,10.);
#15193=VECTOR('',#56563,10.);
#15194=VECTOR('',#56566,10.);
#15195=VECTOR('',#56569,10.);
#15196=VECTOR('',#56572,10.);
#15197=VECTOR('',#56573,10.);
#15198=VECTOR('',#56576,10.);
#15199=VECTOR('',#56579,10.);
#15200=VECTOR('',#56582,10.);
#15201=VECTOR('',#56583,10.);
#15202=VECTOR('',#56586,10.);
#15203=VECTOR('',#56589,10.);
#15204=VECTOR('',#56590,10.);
#15205=VECTOR('',#56593,10.);
#15206=VECTOR('',#56596,10.);
#15207=VECTOR('',#56597,10.);
#15208=VECTOR('',#56600,10.);
#15209=VECTOR('',#56603,10.);
#15210=VECTOR('',#56606,10.);
#15211=VECTOR('',#56607,10.);
#15212=VECTOR('',#56610,10.);
#15213=VECTOR('',#56613,10.);
#15214=VECTOR('',#56616,10.);
#15215=VECTOR('',#56617,10.);
#15216=VECTOR('',#56620,10.);
#15217=VECTOR('',#56623,10.);
#15218=VECTOR('',#56624,10.);
#15219=VECTOR('',#56627,10.);
#15220=VECTOR('',#56630,10.);
#15221=VECTOR('',#56631,10.);
#15222=VECTOR('',#56634,10.);
#15223=VECTOR('',#56637,10.);
#15224=VECTOR('',#56640,10.);
#15225=VECTOR('',#56641,10.);
#15226=VECTOR('',#56644,10.);
#15227=VECTOR('',#56647,10.);
#15228=VECTOR('',#56650,10.);
#15229=VECTOR('',#56651,10.);
#15230=VECTOR('',#56654,10.);
#15231=VECTOR('',#56657,10.);
#15232=VECTOR('',#56658,10.);
#15233=VECTOR('',#56661,10.);
#15234=VECTOR('',#56664,10.);
#15235=VECTOR('',#56665,10.);
#15236=VECTOR('',#56668,10.);
#15237=VECTOR('',#56671,10.);
#15238=VECTOR('',#56674,10.);
#15239=VECTOR('',#56675,10.);
#15240=VECTOR('',#56678,10.);
#15241=VECTOR('',#56681,10.);
#15242=VECTOR('',#56684,10.);
#15243=VECTOR('',#56685,10.);
#15244=VECTOR('',#56688,10.);
#15245=VECTOR('',#56691,10.);
#15246=VECTOR('',#56692,10.);
#15247=VECTOR('',#56695,10.);
#15248=VECTOR('',#56698,10.);
#15249=VECTOR('',#56699,10.);
#15250=VECTOR('',#56702,10.);
#15251=VECTOR('',#56705,10.);
#15252=VECTOR('',#56708,10.);
#15253=VECTOR('',#56709,10.);
#15254=VECTOR('',#56712,10.);
#15255=VECTOR('',#56715,10.);
#15256=VECTOR('',#56718,10.);
#15257=VECTOR('',#56719,10.);
#15258=VECTOR('',#56722,10.);
#15259=VECTOR('',#56725,10.);
#15260=VECTOR('',#56726,10.);
#15261=VECTOR('',#56729,10.);
#15262=VECTOR('',#56732,10.);
#15263=VECTOR('',#56733,10.);
#15264=VECTOR('',#56736,10.);
#15265=VECTOR('',#56739,10.);
#15266=VECTOR('',#56742,10.);
#15267=VECTOR('',#56743,10.);
#15268=VECTOR('',#56746,10.);
#15269=VECTOR('',#56749,10.);
#15270=VECTOR('',#56762,10.);
#15271=VECTOR('',#56763,10.);
#15272=VECTOR('',#56766,10.);
#15273=VECTOR('',#56769,10.);
#15274=VECTOR('',#56770,10.);
#15275=VECTOR('',#56773,10.);
#15276=VECTOR('',#56776,10.);
#15277=VECTOR('',#56777,10.);
#15278=VECTOR('',#56780,10.);
#15279=VECTOR('',#56783,10.);
#15280=VECTOR('',#56786,10.);
#15281=VECTOR('',#56787,10.);
#15282=VECTOR('',#56790,10.);
#15283=VECTOR('',#56793,10.);
#15284=VECTOR('',#56814,10.);
#15285=VECTOR('',#56815,10.);
#15286=VECTOR('',#56818,10.);
#15287=VECTOR('',#56821,10.);
#15288=VECTOR('',#56822,10.);
#15289=VECTOR('',#56825,10.);
#15290=VECTOR('',#56872,10.);
#15291=VECTOR('',#56873,10.);
#15292=VECTOR('',#56876,10.);
#15293=VECTOR('',#56879,10.);
#15294=VECTOR('',#56882,10.);
#15295=VECTOR('',#56883,10.);
#15296=VECTOR('',#56886,10.);
#15297=VECTOR('',#56889,10.);
#15298=VECTOR('',#56890,10.);
#15299=VECTOR('',#56893,10.);
#15300=VECTOR('',#56914,10.);
#15301=VECTOR('',#56915,10.);
#15302=VECTOR('',#56918,10.);
#15303=VECTOR('',#56921,10.);
#15304=VECTOR('',#56924,10.);
#15305=VECTOR('',#56927,10.);
#15306=VECTOR('',#56936,10.);
#15307=VECTOR('',#56939,10.);
#15308=VECTOR('',#56948,10.);
#15309=VECTOR('',#56951,10.);
#15310=VECTOR('',#56956,10.);
#15311=VECTOR('',#56959,10.);
#15312=VECTOR('',#56968,10.);
#15313=VECTOR('',#56971,10.);
#15314=VECTOR('',#56976,10.);
#15315=VECTOR('',#56979,10.);
#15316=VECTOR('',#56988,10.);
#15317=VECTOR('',#56991,10.);
#15318=VECTOR('',#56996,10.);
#15319=VECTOR('',#56999,10.);
#15320=VECTOR('',#57008,10.);
#15321=VECTOR('',#57011,10.);
#15322=VECTOR('',#57016,10.);
#15323=VECTOR('',#57019,10.);
#15324=VECTOR('',#57028,10.);
#15325=VECTOR('',#57031,10.);
#15326=VECTOR('',#57036,10.);
#15327=VECTOR('',#57039,10.);
#15328=VECTOR('',#57048,10.);
#15329=VECTOR('',#57051,10.);
#15330=VECTOR('',#57056,10.);
#15331=VECTOR('',#57059,10.);
#15332=VECTOR('',#57068,10.);
#15333=VECTOR('',#57071,10.);
#18663=VERTEX_POINT('',#88376);
#18664=VERTEX_POINT('',#88378);
#18665=VERTEX_POINT('',#88380);
#18666=VERTEX_POINT('',#88384);
#18667=VERTEX_POINT('',#88386);
#18668=VERTEX_POINT('',#88394);
#18669=VERTEX_POINT('',#88401);
#18670=VERTEX_POINT('',#88408);
#18671=VERTEX_POINT('',#88415);
#18672=VERTEX_POINT('',#88417);
#18673=VERTEX_POINT('',#88424);
#18674=VERTEX_POINT('',#88429);
#18675=VERTEX_POINT('',#88436);
#18676=VERTEX_POINT('',#88444);
#18677=VERTEX_POINT('',#88452);
#18678=VERTEX_POINT('',#88459);
#18679=VERTEX_POINT('',#88466);
#18680=VERTEX_POINT('',#88473);
#18681=VERTEX_POINT('',#88475);
#18682=VERTEX_POINT('',#88482);
#18683=VERTEX_POINT('',#88487);
#18684=VERTEX_POINT('',#88503);
#18685=VERTEX_POINT('',#88514);
#18686=VERTEX_POINT('',#88527);
#18687=VERTEX_POINT('',#88538);
#18688=VERTEX_POINT('',#88551);
#18689=VERTEX_POINT('',#88553);
#18690=VERTEX_POINT('',#88562);
#18691=VERTEX_POINT('',#88564);
#18692=VERTEX_POINT('',#88571);
#18693=VERTEX_POINT('',#88580);
#18694=VERTEX_POINT('',#88582);
#18695=VERTEX_POINT('',#88600);
#18696=VERTEX_POINT('',#88602);
#18697=VERTEX_POINT('',#88606);
#18698=VERTEX_POINT('',#88608);
#18699=VERTEX_POINT('',#88616);
#18700=VERTEX_POINT('',#88623);
#18701=VERTEX_POINT('',#88630);
#18702=VERTEX_POINT('',#88637);
#18703=VERTEX_POINT('',#88639);
#18704=VERTEX_POINT('',#88646);
#18705=VERTEX_POINT('',#88651);
#18706=VERTEX_POINT('',#88658);
#18707=VERTEX_POINT('',#88666);
#18708=VERTEX_POINT('',#88681);
#18709=VERTEX_POINT('',#88686);
#18710=VERTEX_POINT('',#88705);
#18711=VERTEX_POINT('',#88716);
#18712=VERTEX_POINT('',#88729);
#18713=VERTEX_POINT('',#88731);
#18714=VERTEX_POINT('',#88733);
#18715=VERTEX_POINT('',#88737);
#18716=VERTEX_POINT('',#88739);
#18717=VERTEX_POINT('',#88747);
#18718=VERTEX_POINT('',#88754);
#18719=VERTEX_POINT('',#88761);
#18720=VERTEX_POINT('',#88768);
#18721=VERTEX_POINT('',#88770);
#18722=VERTEX_POINT('',#88777);
#18723=VERTEX_POINT('',#88782);
#18724=VERTEX_POINT('',#88789);
#18725=VERTEX_POINT('',#88797);
#18726=VERTEX_POINT('',#88805);
#18727=VERTEX_POINT('',#88812);
#18728=VERTEX_POINT('',#88819);
#18729=VERTEX_POINT('',#88826);
#18730=VERTEX_POINT('',#88828);
#18731=VERTEX_POINT('',#88835);
#18732=VERTEX_POINT('',#88840);
#18733=VERTEX_POINT('',#88856);
#18734=VERTEX_POINT('',#88867);
#18735=VERTEX_POINT('',#88880);
#18736=VERTEX_POINT('',#88891);
#18737=VERTEX_POINT('',#88904);
#18738=VERTEX_POINT('',#88905);
#18739=VERTEX_POINT('',#88907);
#18740=VERTEX_POINT('',#88909);
#18741=VERTEX_POINT('',#88913);
#18742=VERTEX_POINT('',#88915);
#18743=VERTEX_POINT('',#88919);
#18744=VERTEX_POINT('',#88926);
#18745=VERTEX_POINT('',#88934);
#18746=VERTEX_POINT('',#88941);
#18747=VERTEX_POINT('',#88949);
#18748=VERTEX_POINT('',#88956);
#18749=VERTEX_POINT('',#88964);
#18750=VERTEX_POINT('',#88966);
#18751=VERTEX_POINT('',#88968);
#18752=VERTEX_POINT('',#88970);
#18753=VERTEX_POINT('',#88972);
#18754=VERTEX_POINT('',#88974);
#18755=VERTEX_POINT('',#88976);
#18756=VERTEX_POINT('',#88978);
#18757=VERTEX_POINT('',#88980);
#18758=VERTEX_POINT('',#88982);
#18759=VERTEX_POINT('',#88984);
#18760=VERTEX_POINT('',#88986);
#18761=VERTEX_POINT('',#88988);
#18762=VERTEX_POINT('',#88990);
#18763=VERTEX_POINT('',#88992);
#18764=VERTEX_POINT('',#88994);
#18765=VERTEX_POINT('',#88996);
#18766=VERTEX_POINT('',#88998);
#18767=VERTEX_POINT('',#89000);
#18768=VERTEX_POINT('',#89002);
#18769=VERTEX_POINT('',#89004);
#18770=VERTEX_POINT('',#89006);
#18771=VERTEX_POINT('',#89008);
#18772=VERTEX_POINT('',#89010);
#18773=VERTEX_POINT('',#89012);
#18774=VERTEX_POINT('',#89014);
#18775=VERTEX_POINT('',#89016);
#18776=VERTEX_POINT('',#89018);
#18777=VERTEX_POINT('',#89020);
#18778=VERTEX_POINT('',#89022);
#18779=VERTEX_POINT('',#89024);
#18780=VERTEX_POINT('',#89026);
#18781=VERTEX_POINT('',#89028);
#18782=VERTEX_POINT('',#89030);
#18783=VERTEX_POINT('',#89032);
#18784=VERTEX_POINT('',#89034);
#18785=VERTEX_POINT('',#89036);
#18786=VERTEX_POINT('',#89038);
#18787=VERTEX_POINT('',#89040);
#18788=VERTEX_POINT('',#89042);
#18789=VERTEX_POINT('',#89044);
#18790=VERTEX_POINT('',#89046);
#18791=VERTEX_POINT('',#89048);
#18792=VERTEX_POINT('',#89050);
#18793=VERTEX_POINT('',#89052);
#18794=VERTEX_POINT('',#89054);
#18795=VERTEX_POINT('',#89056);
#18796=VERTEX_POINT('',#89058);
#18797=VERTEX_POINT('',#89060);
#18798=VERTEX_POINT('',#89062);
#18799=VERTEX_POINT('',#89064);
#18800=VERTEX_POINT('',#89066);
#18801=VERTEX_POINT('',#89068);
#18802=VERTEX_POINT('',#89070);
#18803=VERTEX_POINT('',#89072);
#18804=VERTEX_POINT('',#89074);
#18805=VERTEX_POINT('',#89076);
#18806=VERTEX_POINT('',#89078);
#18807=VERTEX_POINT('',#89080);
#18808=VERTEX_POINT('',#89082);
#18809=VERTEX_POINT('',#89084);
#18810=VERTEX_POINT('',#89086);
#18811=VERTEX_POINT('',#89088);
#18812=VERTEX_POINT('',#89090);
#18813=VERTEX_POINT('',#89092);
#18814=VERTEX_POINT('',#89094);
#18815=VERTEX_POINT('',#89096);
#18816=VERTEX_POINT('',#89098);
#18817=VERTEX_POINT('',#89100);
#18818=VERTEX_POINT('',#89102);
#18819=VERTEX_POINT('',#89104);
#18820=VERTEX_POINT('',#89106);
#18821=VERTEX_POINT('',#89108);
#18822=VERTEX_POINT('',#89110);
#18823=VERTEX_POINT('',#89112);
#18824=VERTEX_POINT('',#89114);
#18825=VERTEX_POINT('',#89116);
#18826=VERTEX_POINT('',#89118);
#18827=VERTEX_POINT('',#89120);
#18828=VERTEX_POINT('',#89122);
#18829=VERTEX_POINT('',#89124);
#18830=VERTEX_POINT('',#89126);
#18831=VERTEX_POINT('',#89128);
#18832=VERTEX_POINT('',#89130);
#18833=VERTEX_POINT('',#89132);
#18834=VERTEX_POINT('',#89134);
#18835=VERTEX_POINT('',#89136);
#18836=VERTEX_POINT('',#89138);
#18837=VERTEX_POINT('',#89140);
#18838=VERTEX_POINT('',#89142);
#18839=VERTEX_POINT('',#89144);
#18840=VERTEX_POINT('',#89146);
#18841=VERTEX_POINT('',#89148);
#18842=VERTEX_POINT('',#89150);
#18843=VERTEX_POINT('',#89152);
#18844=VERTEX_POINT('',#89154);
#18845=VERTEX_POINT('',#89156);
#18846=VERTEX_POINT('',#89158);
#18847=VERTEX_POINT('',#89160);
#18848=VERTEX_POINT('',#89162);
#18849=VERTEX_POINT('',#89164);
#18850=VERTEX_POINT('',#89166);
#18851=VERTEX_POINT('',#89168);
#18852=VERTEX_POINT('',#89170);
#18853=VERTEX_POINT('',#89172);
#18854=VERTEX_POINT('',#89174);
#18855=VERTEX_POINT('',#89176);
#18856=VERTEX_POINT('',#89178);
#18857=VERTEX_POINT('',#89180);
#18858=VERTEX_POINT('',#89182);
#18859=VERTEX_POINT('',#89184);
#18860=VERTEX_POINT('',#89186);
#18861=VERTEX_POINT('',#89188);
#18862=VERTEX_POINT('',#89190);
#18863=VERTEX_POINT('',#89192);
#18864=VERTEX_POINT('',#89194);
#18865=VERTEX_POINT('',#89196);
#18866=VERTEX_POINT('',#89198);
#18867=VERTEX_POINT('',#89200);
#18868=VERTEX_POINT('',#89202);
#18869=VERTEX_POINT('',#89204);
#18870=VERTEX_POINT('',#89206);
#18871=VERTEX_POINT('',#89208);
#18872=VERTEX_POINT('',#89210);
#18873=VERTEX_POINT('',#89212);
#18874=VERTEX_POINT('',#89214);
#18875=VERTEX_POINT('',#89216);
#18876=VERTEX_POINT('',#89218);
#18877=VERTEX_POINT('',#89220);
#18878=VERTEX_POINT('',#89222);
#18879=VERTEX_POINT('',#89224);
#18880=VERTEX_POINT('',#89226);
#18881=VERTEX_POINT('',#89228);
#18882=VERTEX_POINT('',#89230);
#18883=VERTEX_POINT('',#89232);
#18884=VERTEX_POINT('',#89234);
#18885=VERTEX_POINT('',#89236);
#18886=VERTEX_POINT('',#89238);
#18887=VERTEX_POINT('',#89240);
#18888=VERTEX_POINT('',#89242);
#18889=VERTEX_POINT('',#89244);
#18890=VERTEX_POINT('',#89248);
#18891=VERTEX_POINT('',#89250);
#18892=VERTEX_POINT('',#89254);
#18893=VERTEX_POINT('',#89258);
#18894=VERTEX_POINT('',#89265);
#18895=VERTEX_POINT('',#89273);
#18896=VERTEX_POINT('',#89280);
#18897=VERTEX_POINT('',#89288);
#18898=VERTEX_POINT('',#89295);
#18899=VERTEX_POINT('',#89303);
#18900=VERTEX_POINT('',#89305);
#18901=VERTEX_POINT('',#89307);
#18902=VERTEX_POINT('',#89309);
#18903=VERTEX_POINT('',#89311);
#18904=VERTEX_POINT('',#89313);
#18905=VERTEX_POINT('',#89315);
#18906=VERTEX_POINT('',#89317);
#18907=VERTEX_POINT('',#89319);
#18908=VERTEX_POINT('',#89321);
#18909=VERTEX_POINT('',#89323);
#18910=VERTEX_POINT('',#89325);
#18911=VERTEX_POINT('',#89327);
#18912=VERTEX_POINT('',#89329);
#18913=VERTEX_POINT('',#89331);
#18914=VERTEX_POINT('',#89333);
#18915=VERTEX_POINT('',#89335);
#18916=VERTEX_POINT('',#89337);
#18917=VERTEX_POINT('',#89339);
#18918=VERTEX_POINT('',#89341);
#18919=VERTEX_POINT('',#89343);
#18920=VERTEX_POINT('',#89345);
#18921=VERTEX_POINT('',#89347);
#18922=VERTEX_POINT('',#89349);
#18923=VERTEX_POINT('',#89351);
#18924=VERTEX_POINT('',#89353);
#18925=VERTEX_POINT('',#89355);
#18926=VERTEX_POINT('',#89357);
#18927=VERTEX_POINT('',#89359);
#18928=VERTEX_POINT('',#89361);
#18929=VERTEX_POINT('',#89363);
#18930=VERTEX_POINT('',#89365);
#18931=VERTEX_POINT('',#89367);
#18932=VERTEX_POINT('',#89369);
#18933=VERTEX_POINT('',#89371);
#18934=VERTEX_POINT('',#89373);
#18935=VERTEX_POINT('',#89375);
#18936=VERTEX_POINT('',#89377);
#18937=VERTEX_POINT('',#89379);
#18938=VERTEX_POINT('',#89381);
#18939=VERTEX_POINT('',#89383);
#18940=VERTEX_POINT('',#89385);
#18941=VERTEX_POINT('',#89387);
#18942=VERTEX_POINT('',#89389);
#18943=VERTEX_POINT('',#89391);
#18944=VERTEX_POINT('',#89393);
#18945=VERTEX_POINT('',#89395);
#18946=VERTEX_POINT('',#89397);
#18947=VERTEX_POINT('',#89399);
#18948=VERTEX_POINT('',#89401);
#18949=VERTEX_POINT('',#89403);
#18950=VERTEX_POINT('',#89405);
#18951=VERTEX_POINT('',#89407);
#18952=VERTEX_POINT('',#89409);
#18953=VERTEX_POINT('',#89411);
#18954=VERTEX_POINT('',#89413);
#18955=VERTEX_POINT('',#89415);
#18956=VERTEX_POINT('',#89417);
#18957=VERTEX_POINT('',#89419);
#18958=VERTEX_POINT('',#89421);
#18959=VERTEX_POINT('',#89423);
#18960=VERTEX_POINT('',#89425);
#18961=VERTEX_POINT('',#89427);
#18962=VERTEX_POINT('',#89429);
#18963=VERTEX_POINT('',#89431);
#18964=VERTEX_POINT('',#89433);
#18965=VERTEX_POINT('',#89435);
#18966=VERTEX_POINT('',#89437);
#18967=VERTEX_POINT('',#89439);
#18968=VERTEX_POINT('',#89441);
#18969=VERTEX_POINT('',#89443);
#18970=VERTEX_POINT('',#89445);
#18971=VERTEX_POINT('',#89447);
#18972=VERTEX_POINT('',#89449);
#18973=VERTEX_POINT('',#89451);
#18974=VERTEX_POINT('',#89453);
#18975=VERTEX_POINT('',#89455);
#18976=VERTEX_POINT('',#89457);
#18977=VERTEX_POINT('',#89459);
#18978=VERTEX_POINT('',#89461);
#18979=VERTEX_POINT('',#89463);
#18980=VERTEX_POINT('',#89465);
#18981=VERTEX_POINT('',#89467);
#18982=VERTEX_POINT('',#89469);
#18983=VERTEX_POINT('',#89471);
#18984=VERTEX_POINT('',#89473);
#18985=VERTEX_POINT('',#89475);
#18986=VERTEX_POINT('',#89477);
#18987=VERTEX_POINT('',#89479);
#18988=VERTEX_POINT('',#89481);
#18989=VERTEX_POINT('',#89483);
#18990=VERTEX_POINT('',#89485);
#18991=VERTEX_POINT('',#89487);
#18992=VERTEX_POINT('',#89489);
#18993=VERTEX_POINT('',#89491);
#18994=VERTEX_POINT('',#89493);
#18995=VERTEX_POINT('',#89495);
#18996=VERTEX_POINT('',#89497);
#18997=VERTEX_POINT('',#89499);
#18998=VERTEX_POINT('',#89501);
#18999=VERTEX_POINT('',#89503);
#19000=VERTEX_POINT('',#89505);
#19001=VERTEX_POINT('',#89507);
#19002=VERTEX_POINT('',#89509);
#19003=VERTEX_POINT('',#89511);
#19004=VERTEX_POINT('',#89513);
#19005=VERTEX_POINT('',#89515);
#19006=VERTEX_POINT('',#89517);
#19007=VERTEX_POINT('',#89519);
#19008=VERTEX_POINT('',#89521);
#19009=VERTEX_POINT('',#89523);
#19010=VERTEX_POINT('',#89525);
#19011=VERTEX_POINT('',#89527);
#19012=VERTEX_POINT('',#89529);
#19013=VERTEX_POINT('',#89531);
#19014=VERTEX_POINT('',#89533);
#19015=VERTEX_POINT('',#89535);
#19016=VERTEX_POINT('',#89537);
#19017=VERTEX_POINT('',#89539);
#19018=VERTEX_POINT('',#89541);
#19019=VERTEX_POINT('',#89543);
#19020=VERTEX_POINT('',#89545);
#19021=VERTEX_POINT('',#89547);
#19022=VERTEX_POINT('',#89549);
#19023=VERTEX_POINT('',#89551);
#19024=VERTEX_POINT('',#89553);
#19025=VERTEX_POINT('',#89555);
#19026=VERTEX_POINT('',#89557);
#19027=VERTEX_POINT('',#89559);
#19028=VERTEX_POINT('',#89561);
#19029=VERTEX_POINT('',#89563);
#19030=VERTEX_POINT('',#89565);
#19031=VERTEX_POINT('',#89567);
#19032=VERTEX_POINT('',#89569);
#19033=VERTEX_POINT('',#89571);
#19034=VERTEX_POINT('',#89573);
#19035=VERTEX_POINT('',#89575);
#19036=VERTEX_POINT('',#89577);
#24499=EDGE_CURVE('',#18663,#18663,#9179,.T.);
#24500=EDGE_CURVE('',#18663,#18664,#9180,.T.);
#24501=EDGE_CURVE('',#18664,#18665,#9181,.T.);
#24502=EDGE_CURVE('',#18665,#18664,#9182,.T.);
#24503=EDGE_CURVE('',#18665,#18666,#12543,.T.);
#24504=EDGE_CURVE('',#18667,#18666,#10286,.T.);
#24505=EDGE_CURVE('',#18668,#18667,#10287,.T.);
#24506=EDGE_CURVE('',#18669,#18668,#10288,.F.);
#24507=EDGE_CURVE('',#18670,#18669,#10289,.T.);
#24508=EDGE_CURVE('',#18671,#18670,#9183,.T.);
#24509=EDGE_CURVE('',#18672,#18671,#10290,.T.);
#24510=EDGE_CURVE('',#18673,#18672,#10291,.F.);
#24511=EDGE_CURVE('',#18674,#18673,#10292,.T.);
#24512=EDGE_CURVE('',#18675,#18674,#10293,.T.);
#24513=EDGE_CURVE('',#18676,#18675,#10294,.T.);
#24514=EDGE_CURVE('',#18677,#18676,#10295,.T.);
#24515=EDGE_CURVE('',#18678,#18677,#10296,.F.);
#24516=EDGE_CURVE('',#18679,#18678,#10297,.T.);
#24517=EDGE_CURVE('',#18680,#18679,#9184,.T.);
#24518=EDGE_CURVE('',#18681,#18680,#10298,.T.);
#24519=EDGE_CURVE('',#18682,#18681,#10299,.F.);
#24520=EDGE_CURVE('',#18683,#18682,#10300,.T.);
#24521=EDGE_CURVE('',#18666,#18683,#10301,.T.);
#24522=EDGE_CURVE('',#18670,#18684,#10302,.F.);
#24523=EDGE_CURVE('',#18684,#18685,#9185,.T.);
#24524=EDGE_CURVE('',#18685,#18671,#10303,.F.);
#24525=EDGE_CURVE('',#18685,#18684,#12544,.T.);
#24526=EDGE_CURVE('',#18679,#18686,#10304,.F.);
#24527=EDGE_CURVE('',#18686,#18687,#9186,.T.);
#24528=EDGE_CURVE('',#18687,#18680,#10305,.F.);
#24529=EDGE_CURVE('',#18687,#18686,#12545,.T.);
#24530=EDGE_CURVE('',#18672,#18688,#9187,.T.);
#24531=EDGE_CURVE('',#18688,#18689,#10306,.F.);
#24532=EDGE_CURVE('',#18689,#18673,#9188,.T.);
#24533=EDGE_CURVE('',#18690,#18669,#9189,.T.);
#24534=EDGE_CURVE('',#18690,#18691,#10307,.T.);
#24535=EDGE_CURVE('',#18692,#18691,#10308,.F.);
#24536=EDGE_CURVE('',#18692,#18693,#12546,.T.);
#24537=EDGE_CURVE('',#18694,#18693,#10309,.F.);
#24538=EDGE_CURVE('',#18694,#18688,#10310,.T.);
#24539=EDGE_CURVE('',#18695,#18695,#9190,.T.);
#24540=EDGE_CURVE('',#18695,#18696,#9191,.T.);
#24541=EDGE_CURVE('',#18696,#18696,#9192,.T.);
#24542=EDGE_CURVE('',#18696,#18697,#12547,.T.);
#24543=EDGE_CURVE('',#18698,#18697,#10311,.T.);
#24544=EDGE_CURVE('',#18699,#18698,#10312,.T.);
#24545=EDGE_CURVE('',#18700,#18699,#10313,.F.);
#24546=EDGE_CURVE('',#18701,#18700,#10314,.T.);
#24547=EDGE_CURVE('',#18702,#18701,#9193,.T.);
#24548=EDGE_CURVE('',#18703,#18702,#10315,.T.);
#24549=EDGE_CURVE('',#18704,#18703,#10316,.F.);
#24550=EDGE_CURVE('',#18705,#18704,#10317,.T.);
#24551=EDGE_CURVE('',#18706,#18705,#10318,.T.);
#24552=EDGE_CURVE('',#18707,#18706,#10319,.T.);
#24553=EDGE_CURVE('',#18689,#18707,#10320,.T.);
#24554=EDGE_CURVE('',#18691,#18694,#9194,.T.);
#24555=EDGE_CURVE('',#18708,#18690,#10321,.F.);
#24556=EDGE_CURVE('',#18709,#18708,#10322,.T.);
#24557=EDGE_CURVE('',#18697,#18709,#10323,.T.);
#24558=EDGE_CURVE('',#18693,#18692,#9195,.T.);
#24559=EDGE_CURVE('',#18701,#18710,#10324,.F.);
#24560=EDGE_CURVE('',#18710,#18711,#9196,.T.);
#24561=EDGE_CURVE('',#18711,#18702,#10325,.F.);
#24562=EDGE_CURVE('',#18711,#18710,#12548,.T.);
#24563=EDGE_CURVE('',#18712,#18712,#9197,.T.);
#24564=EDGE_CURVE('',#18712,#18713,#9198,.T.);
#24565=EDGE_CURVE('',#18713,#18714,#9199,.T.);
#24566=EDGE_CURVE('',#18714,#18713,#9200,.T.);
#24567=EDGE_CURVE('',#18714,#18715,#12549,.T.);
#24568=EDGE_CURVE('',#18716,#18715,#10326,.T.);
#24569=EDGE_CURVE('',#18717,#18716,#10327,.T.);
#24570=EDGE_CURVE('',#18718,#18717,#10328,.F.);
#24571=EDGE_CURVE('',#18719,#18718,#10329,.T.);
#24572=EDGE_CURVE('',#18720,#18719,#9201,.T.);
#24573=EDGE_CURVE('',#18721,#18720,#10330,.T.);
#24574=EDGE_CURVE('',#18722,#18721,#10331,.F.);
#24575=EDGE_CURVE('',#18723,#18722,#10332,.T.);
#24576=EDGE_CURVE('',#18724,#18723,#10333,.T.);
#24577=EDGE_CURVE('',#18725,#18724,#10334,.T.);
#24578=EDGE_CURVE('',#18726,#18725,#10335,.T.);
#24579=EDGE_CURVE('',#18727,#18726,#10336,.F.);
#24580=EDGE_CURVE('',#18728,#18727,#10337,.T.);
#24581=EDGE_CURVE('',#18729,#18728,#9202,.T.);
#24582=EDGE_CURVE('',#18730,#18729,#10338,.T.);
#24583=EDGE_CURVE('',#18731,#18730,#10339,.F.);
#24584=EDGE_CURVE('',#18732,#18731,#10340,.T.);
#24585=EDGE_CURVE('',#18715,#18732,#10341,.T.);
#24586=EDGE_CURVE('',#18719,#18733,#10342,.F.);
#24587=EDGE_CURVE('',#18733,#18734,#9203,.T.);
#24588=EDGE_CURVE('',#18734,#18720,#10343,.F.);
#24589=EDGE_CURVE('',#18734,#18733,#12550,.T.);
#24590=EDGE_CURVE('',#18728,#18735,#10344,.F.);
#24591=EDGE_CURVE('',#18735,#18736,#9204,.T.);
#24592=EDGE_CURVE('',#18736,#18729,#10345,.F.);
#24593=EDGE_CURVE('',#18736,#18735,#12551,.T.);
#24594=EDGE_CURVE('',#18737,#18738,#9205,.T.);
#24595=EDGE_CURVE('',#18738,#18739,#12552,.T.);
#24596=EDGE_CURVE('',#18739,#18740,#9206,.T.);
#24597=EDGE_CURVE('',#18740,#18737,#12553,.T.);
#24598=EDGE_CURVE('',#18741,#18738,#12554,.T.);
#24599=EDGE_CURVE('',#18742,#18741,#12555,.T.);
#24600=EDGE_CURVE('',#18742,#18739,#12556,.T.);
#24601=EDGE_CURVE('',#18743,#18706,#10346,.T.);
#24602=EDGE_CURVE('',#18744,#18743,#9207,.T.);
#24603=EDGE_CURVE('',#18724,#18744,#10347,.T.);
#24604=EDGE_CURVE('',#18745,#18724,#10348,.T.);
#24605=EDGE_CURVE('',#18746,#18745,#9208,.T.);
#24606=EDGE_CURVE('',#18675,#18746,#10349,.T.);
#24607=EDGE_CURVE('',#18747,#18675,#10350,.T.);
#24608=EDGE_CURVE('',#18748,#18747,#9209,.T.);
#24609=EDGE_CURVE('',#18706,#18748,#10351,.T.);
#24610=EDGE_CURVE('',#18737,#18749,#12557,.T.);
#24611=EDGE_CURVE('',#18750,#18749,#9210,.T.);
#24612=EDGE_CURVE('',#18750,#18751,#12558,.T.);
#24613=EDGE_CURVE('',#18752,#18751,#9211,.T.);
#24614=EDGE_CURVE('',#18752,#18753,#12559,.T.);
#24615=EDGE_CURVE('',#18754,#18753,#9212,.T.);
#24616=EDGE_CURVE('',#18754,#18755,#12560,.T.);
#24617=EDGE_CURVE('',#18756,#18755,#9213,.T.);
#24618=EDGE_CURVE('',#18756,#18757,#12561,.T.);
#24619=EDGE_CURVE('',#18758,#18757,#9214,.T.);
#24620=EDGE_CURVE('',#18758,#18759,#12562,.T.);
#24621=EDGE_CURVE('',#18760,#18759,#9215,.T.);
#24622=EDGE_CURVE('',#18760,#18761,#12563,.T.);
#24623=EDGE_CURVE('',#18762,#18761,#9216,.T.);
#24624=EDGE_CURVE('',#18762,#18763,#12564,.T.);
#24625=EDGE_CURVE('',#18764,#18763,#9217,.T.);
#24626=EDGE_CURVE('',#18764,#18765,#12565,.T.);
#24627=EDGE_CURVE('',#18766,#18765,#9218,.T.);
#24628=EDGE_CURVE('',#18766,#18767,#12566,.T.);
#24629=EDGE_CURVE('',#18768,#18767,#9219,.T.);
#24630=EDGE_CURVE('',#18768,#18769,#12567,.T.);
#24631=EDGE_CURVE('',#18770,#18769,#9220,.T.);
#24632=EDGE_CURVE('',#18770,#18771,#12568,.T.);
#24633=EDGE_CURVE('',#18772,#18771,#9221,.T.);
#24634=EDGE_CURVE('',#18772,#18773,#12569,.T.);
#24635=EDGE_CURVE('',#18774,#18773,#9222,.T.);
#24636=EDGE_CURVE('',#18774,#18775,#12570,.T.);
#24637=EDGE_CURVE('',#18776,#18775,#9223,.T.);
#24638=EDGE_CURVE('',#18776,#18777,#12571,.T.);
#24639=EDGE_CURVE('',#18778,#18777,#9224,.T.);
#24640=EDGE_CURVE('',#18778,#18779,#12572,.T.);
#24641=EDGE_CURVE('',#18780,#18779,#9225,.T.);
#24642=EDGE_CURVE('',#18780,#18781,#12573,.T.);
#24643=EDGE_CURVE('',#18782,#18781,#9226,.T.);
#24644=EDGE_CURVE('',#18782,#18783,#12574,.T.);
#24645=EDGE_CURVE('',#18784,#18783,#9227,.T.);
#24646=EDGE_CURVE('',#18784,#18785,#12575,.T.);
#24647=EDGE_CURVE('',#18786,#18785,#9228,.T.);
#24648=EDGE_CURVE('',#18786,#18787,#12576,.T.);
#24649=EDGE_CURVE('',#18788,#18787,#9229,.T.);
#24650=EDGE_CURVE('',#18788,#18789,#12577,.T.);
#24651=EDGE_CURVE('',#18790,#18789,#9230,.T.);
#24652=EDGE_CURVE('',#18790,#18791,#12578,.T.);
#24653=EDGE_CURVE('',#18792,#18791,#9231,.T.);
#24654=EDGE_CURVE('',#18792,#18793,#12579,.T.);
#24655=EDGE_CURVE('',#18794,#18793,#9232,.T.);
#24656=EDGE_CURVE('',#18794,#18795,#12580,.T.);
#24657=EDGE_CURVE('',#18796,#18795,#9233,.T.);
#24658=EDGE_CURVE('',#18796,#18797,#12581,.T.);
#24659=EDGE_CURVE('',#18798,#18797,#9234,.T.);
#24660=EDGE_CURVE('',#18798,#18799,#12582,.T.);
#24661=EDGE_CURVE('',#18800,#18799,#9235,.T.);
#24662=EDGE_CURVE('',#18800,#18801,#12583,.T.);
#24663=EDGE_CURVE('',#18802,#18801,#9236,.T.);
#24664=EDGE_CURVE('',#18802,#18803,#12584,.T.);
#24665=EDGE_CURVE('',#18804,#18803,#9237,.T.);
#24666=EDGE_CURVE('',#18804,#18805,#12585,.T.);
#24667=EDGE_CURVE('',#18806,#18805,#9238,.T.);
#24668=EDGE_CURVE('',#18806,#18807,#12586,.T.);
#24669=EDGE_CURVE('',#18808,#18807,#9239,.T.);
#24670=EDGE_CURVE('',#18808,#18809,#12587,.T.);
#24671=EDGE_CURVE('',#18810,#18809,#9240,.T.);
#24672=EDGE_CURVE('',#18810,#18811,#12588,.T.);
#24673=EDGE_CURVE('',#18812,#18811,#9241,.T.);
#24674=EDGE_CURVE('',#18812,#18813,#12589,.T.);
#24675=EDGE_CURVE('',#18814,#18813,#9242,.T.);
#24676=EDGE_CURVE('',#18814,#18815,#12590,.T.);
#24677=EDGE_CURVE('',#18816,#18815,#9243,.T.);
#24678=EDGE_CURVE('',#18816,#18817,#12591,.T.);
#24679=EDGE_CURVE('',#18818,#18817,#9244,.T.);
#24680=EDGE_CURVE('',#18818,#18819,#12592,.T.);
#24681=EDGE_CURVE('',#18820,#18819,#9245,.T.);
#24682=EDGE_CURVE('',#18820,#18821,#12593,.T.);
#24683=EDGE_CURVE('',#18822,#18821,#9246,.T.);
#24684=EDGE_CURVE('',#18822,#18823,#12594,.T.);
#24685=EDGE_CURVE('',#18824,#18823,#9247,.T.);
#24686=EDGE_CURVE('',#18824,#18825,#12595,.T.);
#24687=EDGE_CURVE('',#18826,#18825,#9248,.T.);
#24688=EDGE_CURVE('',#18826,#18827,#12596,.T.);
#24689=EDGE_CURVE('',#18828,#18827,#9249,.T.);
#24690=EDGE_CURVE('',#18828,#18829,#12597,.T.);
#24691=EDGE_CURVE('',#18830,#18829,#9250,.T.);
#24692=EDGE_CURVE('',#18830,#18831,#12598,.T.);
#24693=EDGE_CURVE('',#18832,#18831,#9251,.T.);
#24694=EDGE_CURVE('',#18832,#18833,#12599,.T.);
#24695=EDGE_CURVE('',#18834,#18833,#9252,.T.);
#24696=EDGE_CURVE('',#18834,#18835,#12600,.T.);
#24697=EDGE_CURVE('',#18836,#18835,#9253,.T.);
#24698=EDGE_CURVE('',#18836,#18837,#12601,.T.);
#24699=EDGE_CURVE('',#18838,#18837,#9254,.T.);
#24700=EDGE_CURVE('',#18838,#18839,#12602,.T.);
#24701=EDGE_CURVE('',#18840,#18839,#9255,.T.);
#24702=EDGE_CURVE('',#18840,#18841,#12603,.T.);
#24703=EDGE_CURVE('',#18842,#18841,#9256,.T.);
#24704=EDGE_CURVE('',#18842,#18843,#12604,.T.);
#24705=EDGE_CURVE('',#18844,#18843,#9257,.T.);
#24706=EDGE_CURVE('',#18844,#18845,#12605,.T.);
#24707=EDGE_CURVE('',#18846,#18845,#9258,.T.);
#24708=EDGE_CURVE('',#18846,#18847,#12606,.T.);
#24709=EDGE_CURVE('',#18848,#18847,#9259,.T.);
#24710=EDGE_CURVE('',#18848,#18849,#12607,.T.);
#24711=EDGE_CURVE('',#18850,#18849,#9260,.T.);
#24712=EDGE_CURVE('',#18850,#18851,#12608,.T.);
#24713=EDGE_CURVE('',#18852,#18851,#9261,.T.);
#24714=EDGE_CURVE('',#18852,#18853,#12609,.T.);
#24715=EDGE_CURVE('',#18854,#18853,#9262,.T.);
#24716=EDGE_CURVE('',#18854,#18855,#12610,.T.);
#24717=EDGE_CURVE('',#18856,#18855,#9263,.T.);
#24718=EDGE_CURVE('',#18856,#18857,#12611,.T.);
#24719=EDGE_CURVE('',#18858,#18857,#9264,.T.);
#24720=EDGE_CURVE('',#18858,#18859,#12612,.T.);
#24721=EDGE_CURVE('',#18860,#18859,#9265,.T.);
#24722=EDGE_CURVE('',#18860,#18861,#12613,.T.);
#24723=EDGE_CURVE('',#18862,#18861,#9266,.T.);
#24724=EDGE_CURVE('',#18862,#18863,#12614,.T.);
#24725=EDGE_CURVE('',#18864,#18863,#9267,.T.);
#24726=EDGE_CURVE('',#18864,#18865,#12615,.T.);
#24727=EDGE_CURVE('',#18866,#18865,#9268,.T.);
#24728=EDGE_CURVE('',#18866,#18867,#12616,.T.);
#24729=EDGE_CURVE('',#18868,#18867,#9269,.T.);
#24730=EDGE_CURVE('',#18868,#18869,#12617,.T.);
#24731=EDGE_CURVE('',#18870,#18869,#9270,.T.);
#24732=EDGE_CURVE('',#18870,#18871,#12618,.T.);
#24733=EDGE_CURVE('',#18872,#18871,#9271,.T.);
#24734=EDGE_CURVE('',#18872,#18873,#12619,.T.);
#24735=EDGE_CURVE('',#18874,#18873,#9272,.T.);
#24736=EDGE_CURVE('',#18874,#18875,#12620,.T.);
#24737=EDGE_CURVE('',#18876,#18875,#9273,.T.);
#24738=EDGE_CURVE('',#18876,#18877,#12621,.T.);
#24739=EDGE_CURVE('',#18878,#18877,#9274,.T.);
#24740=EDGE_CURVE('',#18878,#18879,#12622,.T.);
#24741=EDGE_CURVE('',#18880,#18879,#9275,.T.);
#24742=EDGE_CURVE('',#18880,#18881,#12623,.T.);
#24743=EDGE_CURVE('',#18882,#18881,#9276,.T.);
#24744=EDGE_CURVE('',#18882,#18883,#12624,.T.);
#24745=EDGE_CURVE('',#18884,#18883,#9277,.T.);
#24746=EDGE_CURVE('',#18884,#18885,#12625,.T.);
#24747=EDGE_CURVE('',#18886,#18885,#9278,.T.);
#24748=EDGE_CURVE('',#18886,#18887,#12626,.T.);
#24749=EDGE_CURVE('',#18888,#18887,#9279,.T.);
#24750=EDGE_CURVE('',#18888,#18889,#12627,.T.);
#24751=EDGE_CURVE('',#18741,#18889,#9280,.T.);
#24752=EDGE_CURVE('',#18749,#18890,#12628,.T.);
#24753=EDGE_CURVE('',#18890,#18891,#9281,.T.);
#24754=EDGE_CURVE('',#18891,#18750,#12629,.T.);
#24755=EDGE_CURVE('',#18891,#18892,#12630,.T.);
#24756=EDGE_CURVE('',#18751,#18892,#12631,.T.);
#24757=EDGE_CURVE('',#18893,#18715,#10352,.T.);
#24758=EDGE_CURVE('',#18894,#18893,#9282,.T.);
#24759=EDGE_CURVE('',#18697,#18894,#10353,.T.);
#24760=EDGE_CURVE('',#18895,#18697,#10354,.T.);
#24761=EDGE_CURVE('',#18896,#18895,#9283,.T.);
#24762=EDGE_CURVE('',#18666,#18896,#10355,.T.);
#24763=EDGE_CURVE('',#18897,#18666,#10356,.T.);
#24764=EDGE_CURVE('',#18898,#18897,#9284,.T.);
#24765=EDGE_CURVE('',#18715,#18898,#10357,.T.);
#24766=EDGE_CURVE('',#18742,#18899,#9285,.T.);
#24767=EDGE_CURVE('',#18900,#18899,#12632,.T.);
#24768=EDGE_CURVE('',#18901,#18900,#9286,.T.);
#24769=EDGE_CURVE('',#18902,#18901,#12633,.T.);
#24770=EDGE_CURVE('',#18903,#18902,#9287,.T.);
#24771=EDGE_CURVE('',#18904,#18903,#12634,.T.);
#24772=EDGE_CURVE('',#18904,#18905,#9288,.T.);
#24773=EDGE_CURVE('',#18906,#18905,#12635,.T.);
#24774=EDGE_CURVE('',#18907,#18906,#9289,.T.);
#24775=EDGE_CURVE('',#18908,#18907,#12636,.T.);
#24776=EDGE_CURVE('',#18909,#18908,#9290,.T.);
#24777=EDGE_CURVE('',#18910,#18909,#12637,.T.);
#24778=EDGE_CURVE('',#18910,#18911,#9291,.T.);
#24779=EDGE_CURVE('',#18912,#18911,#12638,.T.);
#24780=EDGE_CURVE('',#18913,#18912,#9292,.T.);
#24781=EDGE_CURVE('',#18914,#18913,#12639,.T.);
#24782=EDGE_CURVE('',#18915,#18914,#9293,.T.);
#24783=EDGE_CURVE('',#18916,#18915,#12640,.T.);
#24784=EDGE_CURVE('',#18916,#18917,#9294,.T.);
#24785=EDGE_CURVE('',#18918,#18917,#12641,.T.);
#24786=EDGE_CURVE('',#18919,#18918,#9295,.T.);
#24787=EDGE_CURVE('',#18920,#18919,#12642,.T.);
#24788=EDGE_CURVE('',#18921,#18920,#9296,.T.);
#24789=EDGE_CURVE('',#18922,#18921,#12643,.T.);
#24790=EDGE_CURVE('',#18922,#18923,#9297,.T.);
#24791=EDGE_CURVE('',#18924,#18923,#12644,.T.);
#24792=EDGE_CURVE('',#18925,#18924,#9298,.T.);
#24793=EDGE_CURVE('',#18926,#18925,#12645,.T.);
#24794=EDGE_CURVE('',#18927,#18926,#9299,.T.);
#24795=EDGE_CURVE('',#18928,#18927,#12646,.T.);
#24796=EDGE_CURVE('',#18928,#18929,#9300,.T.);
#24797=EDGE_CURVE('',#18930,#18929,#12647,.T.);
#24798=EDGE_CURVE('',#18931,#18930,#9301,.T.);
#24799=EDGE_CURVE('',#18932,#18931,#12648,.T.);
#24800=EDGE_CURVE('',#18933,#18932,#9302,.T.);
#24801=EDGE_CURVE('',#18934,#18933,#12649,.T.);
#24802=EDGE_CURVE('',#18934,#18935,#9303,.T.);
#24803=EDGE_CURVE('',#18936,#18935,#12650,.T.);
#24804=EDGE_CURVE('',#18937,#18936,#9304,.T.);
#24805=EDGE_CURVE('',#18938,#18937,#12651,.T.);
#24806=EDGE_CURVE('',#18939,#18938,#9305,.T.);
#24807=EDGE_CURVE('',#18940,#18939,#12652,.T.);
#24808=EDGE_CURVE('',#18940,#18941,#9306,.T.);
#24809=EDGE_CURVE('',#18942,#18941,#12653,.T.);
#24810=EDGE_CURVE('',#18943,#18942,#9307,.T.);
#24811=EDGE_CURVE('',#18944,#18943,#12654,.T.);
#24812=EDGE_CURVE('',#18945,#18944,#9308,.T.);
#24813=EDGE_CURVE('',#18946,#18945,#12655,.T.);
#24814=EDGE_CURVE('',#18946,#18947,#9309,.T.);
#24815=EDGE_CURVE('',#18948,#18947,#12656,.T.);
#24816=EDGE_CURVE('',#18949,#18948,#9310,.T.);
#24817=EDGE_CURVE('',#18950,#18949,#12657,.T.);
#24818=EDGE_CURVE('',#18951,#18950,#9311,.T.);
#24819=EDGE_CURVE('',#18952,#18951,#12658,.T.);
#24820=EDGE_CURVE('',#18952,#18953,#9312,.T.);
#24821=EDGE_CURVE('',#18954,#18953,#12659,.T.);
#24822=EDGE_CURVE('',#18955,#18954,#9313,.T.);
#24823=EDGE_CURVE('',#18956,#18955,#12660,.T.);
#24824=EDGE_CURVE('',#18957,#18956,#9314,.T.);
#24825=EDGE_CURVE('',#18958,#18957,#12661,.T.);
#24826=EDGE_CURVE('',#18958,#18959,#9315,.T.);
#24827=EDGE_CURVE('',#18960,#18959,#12662,.T.);
#24828=EDGE_CURVE('',#18961,#18960,#9316,.T.);
#24829=EDGE_CURVE('',#18962,#18961,#12663,.T.);
#24830=EDGE_CURVE('',#18963,#18962,#9317,.T.);
#24831=EDGE_CURVE('',#18964,#18963,#12664,.T.);
#24832=EDGE_CURVE('',#18964,#18965,#9318,.T.);
#24833=EDGE_CURVE('',#18966,#18965,#12665,.T.);
#24834=EDGE_CURVE('',#18967,#18966,#9319,.T.);
#24835=EDGE_CURVE('',#18968,#18967,#12666,.T.);
#24836=EDGE_CURVE('',#18969,#18968,#9320,.T.);
#24837=EDGE_CURVE('',#18970,#18969,#12667,.T.);
#24838=EDGE_CURVE('',#18970,#18971,#9321,.T.);
#24839=EDGE_CURVE('',#18972,#18971,#12668,.T.);
#24840=EDGE_CURVE('',#18973,#18972,#9322,.T.);
#24841=EDGE_CURVE('',#18974,#18973,#12669,.T.);
#24842=EDGE_CURVE('',#18975,#18974,#9323,.T.);
#24843=EDGE_CURVE('',#18976,#18975,#12670,.T.);
#24844=EDGE_CURVE('',#18976,#18977,#9324,.T.);
#24845=EDGE_CURVE('',#18978,#18977,#12671,.T.);
#24846=EDGE_CURVE('',#18979,#18978,#9325,.T.);
#24847=EDGE_CURVE('',#18980,#18979,#12672,.T.);
#24848=EDGE_CURVE('',#18981,#18980,#9326,.T.);
#24849=EDGE_CURVE('',#18982,#18981,#12673,.T.);
#24850=EDGE_CURVE('',#18982,#18983,#9327,.T.);
#24851=EDGE_CURVE('',#18984,#18983,#12674,.T.);
#24852=EDGE_CURVE('',#18985,#18984,#9328,.T.);
#24853=EDGE_CURVE('',#18986,#18985,#12675,.T.);
#24854=EDGE_CURVE('',#18987,#18986,#9329,.T.);
#24855=EDGE_CURVE('',#18988,#18987,#12676,.T.);
#24856=EDGE_CURVE('',#18988,#18989,#9330,.T.);
#24857=EDGE_CURVE('',#18990,#18989,#12677,.T.);
#24858=EDGE_CURVE('',#18991,#18990,#9331,.T.);
#24859=EDGE_CURVE('',#18992,#18991,#12678,.T.);
#24860=EDGE_CURVE('',#18993,#18992,#9332,.T.);
#24861=EDGE_CURVE('',#18994,#18993,#12679,.T.);
#24862=EDGE_CURVE('',#18994,#18995,#9333,.T.);
#24863=EDGE_CURVE('',#18996,#18995,#12680,.T.);
#24864=EDGE_CURVE('',#18997,#18996,#9334,.T.);
#24865=EDGE_CURVE('',#18998,#18997,#12681,.T.);
#24866=EDGE_CURVE('',#18999,#18998,#9335,.T.);
#24867=EDGE_CURVE('',#19000,#18999,#12682,.T.);
#24868=EDGE_CURVE('',#19000,#19001,#9336,.T.);
#24869=EDGE_CURVE('',#19002,#19001,#12683,.T.);
#24870=EDGE_CURVE('',#19003,#19002,#9337,.T.);
#24871=EDGE_CURVE('',#19004,#19003,#12684,.T.);
#24872=EDGE_CURVE('',#19005,#19004,#9338,.T.);
#24873=EDGE_CURVE('',#19006,#19005,#12685,.T.);
#24874=EDGE_CURVE('',#19006,#19007,#9339,.T.);
#24875=EDGE_CURVE('',#19008,#19007,#12686,.T.);
#24876=EDGE_CURVE('',#19009,#19008,#9340,.T.);
#24877=EDGE_CURVE('',#19010,#19009,#12687,.T.);
#24878=EDGE_CURVE('',#19011,#19010,#9341,.T.);
#24879=EDGE_CURVE('',#19012,#19011,#12688,.T.);
#24880=EDGE_CURVE('',#19012,#19013,#9342,.T.);
#24881=EDGE_CURVE('',#19014,#19013,#12689,.T.);
#24882=EDGE_CURVE('',#19015,#19014,#9343,.T.);
#24883=EDGE_CURVE('',#19016,#19015,#12690,.T.);
#24884=EDGE_CURVE('',#19017,#19016,#9344,.T.);
#24885=EDGE_CURVE('',#19018,#19017,#12691,.T.);
#24886=EDGE_CURVE('',#19018,#19019,#9345,.T.);
#24887=EDGE_CURVE('',#19020,#19019,#12692,.T.);
#24888=EDGE_CURVE('',#19021,#19020,#9346,.T.);
#24889=EDGE_CURVE('',#19022,#19021,#12693,.T.);
#24890=EDGE_CURVE('',#19023,#19022,#9347,.T.);
#24891=EDGE_CURVE('',#19024,#19023,#12694,.T.);
#24892=EDGE_CURVE('',#19024,#19025,#9348,.T.);
#24893=EDGE_CURVE('',#19026,#19025,#12695,.T.);
#24894=EDGE_CURVE('',#19027,#19026,#9349,.T.);
#24895=EDGE_CURVE('',#19028,#19027,#12696,.T.);
#24896=EDGE_CURVE('',#19029,#19028,#9350,.T.);
#24897=EDGE_CURVE('',#19030,#19029,#12697,.T.);
#24898=EDGE_CURVE('',#19030,#19031,#9351,.T.);
#24899=EDGE_CURVE('',#19032,#19031,#12698,.T.);
#24900=EDGE_CURVE('',#19033,#19032,#9352,.T.);
#24901=EDGE_CURVE('',#19034,#19033,#12699,.T.);
#24902=EDGE_CURVE('',#19035,#19034,#9353,.T.);
#24903=EDGE_CURVE('',#19036,#19035,#12700,.T.);
#24904=EDGE_CURVE('',#19036,#18892,#9354,.T.);
#24905=EDGE_CURVE('',#18740,#18890,#12701,.T.);
#24906=EDGE_CURVE('',#18885,#18903,#12702,.T.);
#24907=EDGE_CURVE('',#18902,#18886,#12703,.T.);
#24908=EDGE_CURVE('',#18887,#18901,#12704,.T.);
#24909=EDGE_CURVE('',#18900,#18888,#12705,.T.);
#24910=EDGE_CURVE('',#18881,#18907,#12706,.T.);
#24911=EDGE_CURVE('',#18906,#18882,#12707,.T.);
#24912=EDGE_CURVE('',#18883,#18905,#12708,.T.);
#24913=EDGE_CURVE('',#18879,#18909,#12709,.T.);
#24914=EDGE_CURVE('',#18908,#18880,#12710,.T.);
#24915=EDGE_CURVE('',#18910,#18878,#12711,.T.);
#24916=EDGE_CURVE('',#18875,#18913,#12712,.T.);
#24917=EDGE_CURVE('',#18912,#18876,#12713,.T.);
#24918=EDGE_CURVE('',#18914,#18874,#12714,.T.);
#24919=EDGE_CURVE('',#18873,#18915,#12715,.T.);
#24920=EDGE_CURVE('',#18867,#18921,#12716,.T.);
#24921=EDGE_CURVE('',#18920,#18868,#12717,.T.);
#24922=EDGE_CURVE('',#18869,#18919,#12718,.T.);
#24923=EDGE_CURVE('',#18918,#18870,#12719,.T.);
#24924=EDGE_CURVE('',#18863,#18925,#12720,.T.);
#24925=EDGE_CURVE('',#18924,#18864,#12721,.T.);
#24926=EDGE_CURVE('',#18865,#18923,#12722,.T.);
#24927=EDGE_CURVE('',#18861,#18927,#12723,.T.);
#24928=EDGE_CURVE('',#18926,#18862,#12724,.T.);
#24929=EDGE_CURVE('',#18928,#18860,#12725,.T.);
#24930=EDGE_CURVE('',#18857,#18931,#12726,.T.);
#24931=EDGE_CURVE('',#18930,#18858,#12727,.T.);
#24932=EDGE_CURVE('',#18932,#18856,#12728,.T.);
#24933=EDGE_CURVE('',#18855,#18933,#12729,.T.);
#24934=EDGE_CURVE('',#18849,#18939,#12730,.T.);
#24935=EDGE_CURVE('',#18938,#18850,#12731,.T.);
#24936=EDGE_CURVE('',#18851,#18937,#12732,.T.);
#24937=EDGE_CURVE('',#18936,#18852,#12733,.T.);
#24938=EDGE_CURVE('',#18845,#18943,#12734,.T.);
#24939=EDGE_CURVE('',#18942,#18846,#12735,.T.);
#24940=EDGE_CURVE('',#18847,#18941,#12736,.T.);
#24941=EDGE_CURVE('',#18843,#18945,#12737,.T.);
#24942=EDGE_CURVE('',#18944,#18844,#12738,.T.);
#24943=EDGE_CURVE('',#18946,#18842,#12739,.T.);
#24944=EDGE_CURVE('',#18839,#18949,#12740,.T.);
#24945=EDGE_CURVE('',#18948,#18840,#12741,.T.);
#24946=EDGE_CURVE('',#18950,#18838,#12742,.T.);
#24947=EDGE_CURVE('',#18837,#18951,#12743,.T.);
#24948=EDGE_CURVE('',#18831,#18957,#12744,.T.);
#24949=EDGE_CURVE('',#18956,#18832,#12745,.T.);
#24950=EDGE_CURVE('',#18833,#18955,#12746,.T.);
#24951=EDGE_CURVE('',#18954,#18834,#12747,.T.);
#24952=EDGE_CURVE('',#18827,#18961,#12748,.T.);
#24953=EDGE_CURVE('',#18960,#18828,#12749,.T.);
#24954=EDGE_CURVE('',#18829,#18959,#12750,.T.);
#24955=EDGE_CURVE('',#18825,#18963,#12751,.T.);
#24956=EDGE_CURVE('',#18962,#18826,#12752,.T.);
#24957=EDGE_CURVE('',#18964,#18824,#12753,.T.);
#24958=EDGE_CURVE('',#18821,#18967,#12754,.T.);
#24959=EDGE_CURVE('',#18966,#18822,#12755,.T.);
#24960=EDGE_CURVE('',#18968,#18820,#12756,.T.);
#24961=EDGE_CURVE('',#18819,#18969,#12757,.T.);
#24962=EDGE_CURVE('',#18813,#18975,#12758,.T.);
#24963=EDGE_CURVE('',#18974,#18814,#12759,.T.);
#24964=EDGE_CURVE('',#18815,#18973,#12760,.T.);
#24965=EDGE_CURVE('',#18972,#18816,#12761,.T.);
#24966=EDGE_CURVE('',#18809,#18979,#12762,.T.);
#24967=EDGE_CURVE('',#18978,#18810,#12763,.T.);
#24968=EDGE_CURVE('',#18811,#18977,#12764,.T.);
#24969=EDGE_CURVE('',#18807,#18981,#12765,.T.);
#24970=EDGE_CURVE('',#18980,#18808,#12766,.T.);
#24971=EDGE_CURVE('',#18982,#18806,#12767,.T.);
#24972=EDGE_CURVE('',#18803,#18985,#12768,.T.);
#24973=EDGE_CURVE('',#18984,#18804,#12769,.T.);
#24974=EDGE_CURVE('',#18986,#18802,#12770,.T.);
#24975=EDGE_CURVE('',#18801,#18987,#12771,.T.);
#24976=EDGE_CURVE('',#18795,#18993,#12772,.T.);
#24977=EDGE_CURVE('',#18992,#18796,#12773,.T.);
#24978=EDGE_CURVE('',#18797,#18991,#12774,.T.);
#24979=EDGE_CURVE('',#18990,#18798,#12775,.T.);
#24980=EDGE_CURVE('',#18717,#18682,#9355,.T.);
#24981=EDGE_CURVE('',#18681,#18718,#9356,.T.);
#24982=EDGE_CURVE('',#18683,#18716,#9357,.T.);
#24983=EDGE_CURVE('',#18791,#18997,#12776,.T.);
#24984=EDGE_CURVE('',#18996,#18792,#12777,.T.);
#24985=EDGE_CURVE('',#18793,#18995,#12778,.T.);
#24986=EDGE_CURVE('',#18789,#18999,#12779,.T.);
#24987=EDGE_CURVE('',#18998,#18790,#12780,.T.);
#24988=EDGE_CURVE('',#19000,#18788,#12781,.T.);
#24989=EDGE_CURVE('',#18785,#19003,#12782,.T.);
#24990=EDGE_CURVE('',#19002,#18786,#12783,.T.);
#24991=EDGE_CURVE('',#19004,#18784,#12784,.T.);
#24992=EDGE_CURVE('',#18783,#19005,#12785,.T.);
#24993=EDGE_CURVE('',#18777,#19011,#12786,.T.);
#24994=EDGE_CURVE('',#19010,#18778,#12787,.T.);
#24995=EDGE_CURVE('',#18779,#19009,#12788,.T.);
#24996=EDGE_CURVE('',#19008,#18780,#12789,.T.);
#24997=EDGE_CURVE('',#18703,#18727,#9358,.T.);
#24998=EDGE_CURVE('',#18726,#18704,#9359,.T.);
#24999=EDGE_CURVE('',#18730,#18700,#9360,.T.);
#25000=EDGE_CURVE('',#18721,#18678,#9361,.T.);
#25001=EDGE_CURVE('',#18677,#18722,#9362,.T.);
#25002=EDGE_CURVE('',#18773,#19015,#12790,.T.);
#25003=EDGE_CURVE('',#19014,#18774,#12791,.T.);
#25004=EDGE_CURVE('',#18775,#19013,#12792,.T.);
#25005=EDGE_CURVE('',#18771,#19017,#12793,.T.);
#25006=EDGE_CURVE('',#19016,#18772,#12794,.T.);
#25007=EDGE_CURVE('',#19018,#18770,#12795,.T.);
#25008=EDGE_CURVE('',#18699,#18731,#9363,.T.);
#25009=EDGE_CURVE('',#18732,#18698,#9364,.T.);
#25010=EDGE_CURVE('',#18668,#18708,#9365,.T.);
#25011=EDGE_CURVE('',#18709,#18667,#9366,.T.);
#25012=EDGE_CURVE('',#18747,#18674,#9367,.T.);
#25013=EDGE_CURVE('',#18674,#18707,#9368,.T.);
#25014=EDGE_CURVE('',#18707,#18748,#9369,.T.);
#25015=EDGE_CURVE('',#18745,#18723,#9370,.T.);
#25016=EDGE_CURVE('',#18723,#18676,#9371,.T.);
#25017=EDGE_CURVE('',#18676,#18746,#9372,.T.);
#25018=EDGE_CURVE('',#18743,#18705,#9373,.T.);
#25019=EDGE_CURVE('',#18705,#18725,#9374,.T.);
#25020=EDGE_CURVE('',#18725,#18744,#9375,.T.);
#25021=EDGE_CURVE('',#18767,#19021,#12796,.T.);
#25022=EDGE_CURVE('',#19020,#18768,#12797,.T.);
#25023=EDGE_CURVE('',#19022,#18766,#12798,.T.);
#25024=EDGE_CURVE('',#18765,#19023,#12799,.T.);
#25025=EDGE_CURVE('',#18759,#19029,#12800,.T.);
#25026=EDGE_CURVE('',#19028,#18760,#12801,.T.);
#25027=EDGE_CURVE('',#19030,#18758,#12802,.T.);
#25028=EDGE_CURVE('',#18761,#19027,#12803,.T.);
#25029=EDGE_CURVE('',#19026,#18762,#12804,.T.);
#25030=EDGE_CURVE('',#18763,#19025,#12805,.T.);
#25031=EDGE_CURVE('',#18667,#18896,#9376,.T.);
#25032=EDGE_CURVE('',#18895,#18709,#9377,.T.);
#25033=EDGE_CURVE('',#18716,#18898,#9378,.T.);
#25034=EDGE_CURVE('',#18897,#18683,#9379,.T.);
#25035=EDGE_CURVE('',#18698,#18894,#9380,.T.);
#25036=EDGE_CURVE('',#18893,#18732,#9381,.T.);
#25037=EDGE_CURVE('',#18755,#19033,#12806,.T.);
#25038=EDGE_CURVE('',#19032,#18756,#12807,.T.);
#25039=EDGE_CURVE('',#19034,#18754,#12808,.T.);
#25040=EDGE_CURVE('',#18753,#19035,#12809,.T.);
#25041=EDGE_CURVE('',#19036,#18752,#12810,.T.);
#25042=EDGE_CURVE('',#18757,#19031,#12811,.T.);
#25043=EDGE_CURVE('',#19024,#18764,#12812,.T.);
#25044=EDGE_CURVE('',#18769,#19019,#12813,.T.);
#25045=EDGE_CURVE('',#19012,#18776,#12814,.T.);
#25046=EDGE_CURVE('',#18781,#19007,#12815,.T.);
#25047=EDGE_CURVE('',#19006,#18782,#12816,.T.);
#25048=EDGE_CURVE('',#18787,#19001,#12817,.T.);
#25049=EDGE_CURVE('',#18994,#18794,#12818,.T.);
#25050=EDGE_CURVE('',#18799,#18989,#12819,.T.);
#25051=EDGE_CURVE('',#18988,#18800,#12820,.T.);
#25052=EDGE_CURVE('',#18805,#18983,#12821,.T.);
#25053=EDGE_CURVE('',#18976,#18812,#12822,.T.);
#25054=EDGE_CURVE('',#18817,#18971,#12823,.T.);
#25055=EDGE_CURVE('',#18970,#18818,#12824,.T.);
#25056=EDGE_CURVE('',#18823,#18965,#12825,.T.);
#25057=EDGE_CURVE('',#18958,#18830,#12826,.T.);
#25058=EDGE_CURVE('',#18835,#18953,#12827,.T.);
#25059=EDGE_CURVE('',#18952,#18836,#12828,.T.);
#25060=EDGE_CURVE('',#18841,#18947,#12829,.T.);
#25061=EDGE_CURVE('',#18940,#18848,#12830,.T.);
#25062=EDGE_CURVE('',#18853,#18935,#12831,.T.);
#25063=EDGE_CURVE('',#18934,#18854,#12832,.T.);
#25064=EDGE_CURVE('',#18859,#18929,#12833,.T.);
#25065=EDGE_CURVE('',#18922,#18866,#12834,.T.);
#25066=EDGE_CURVE('',#18871,#18917,#12835,.T.);
#25067=EDGE_CURVE('',#18916,#18872,#12836,.T.);
#25068=EDGE_CURVE('',#18877,#18911,#12837,.T.);
#25069=EDGE_CURVE('',#18904,#18884,#12838,.T.);
#25070=EDGE_CURVE('',#18889,#18899,#12839,.T.);
#35975=ORIENTED_EDGE('',*,*,#24499,.T.);
#35976=ORIENTED_EDGE('',*,*,#24500,.T.);
#35977=ORIENTED_EDGE('',*,*,#24501,.T.);
#35978=ORIENTED_EDGE('',*,*,#24502,.T.);
#35979=ORIENTED_EDGE('',*,*,#24500,.F.);
#35980=ORIENTED_EDGE('',*,*,#24502,.F.);
#35981=ORIENTED_EDGE('',*,*,#24503,.T.);
#35982=ORIENTED_EDGE('',*,*,#24504,.F.);
#35983=ORIENTED_EDGE('',*,*,#24505,.F.);
#35984=ORIENTED_EDGE('',*,*,#24506,.F.);
#35985=ORIENTED_EDGE('',*,*,#24507,.F.);
#35986=ORIENTED_EDGE('',*,*,#24508,.F.);
#35987=ORIENTED_EDGE('',*,*,#24509,.F.);
#35988=ORIENTED_EDGE('',*,*,#24510,.F.);
#35989=ORIENTED_EDGE('',*,*,#24511,.F.);
#35990=ORIENTED_EDGE('',*,*,#24512,.F.);
#35991=ORIENTED_EDGE('',*,*,#24513,.F.);
#35992=ORIENTED_EDGE('',*,*,#24514,.F.);
#35993=ORIENTED_EDGE('',*,*,#24515,.F.);
#35994=ORIENTED_EDGE('',*,*,#24516,.F.);
#35995=ORIENTED_EDGE('',*,*,#24517,.F.);
#35996=ORIENTED_EDGE('',*,*,#24518,.F.);
#35997=ORIENTED_EDGE('',*,*,#24519,.F.);
#35998=ORIENTED_EDGE('',*,*,#24520,.F.);
#35999=ORIENTED_EDGE('',*,*,#24521,.F.);
#36000=ORIENTED_EDGE('',*,*,#24503,.F.);
#36001=ORIENTED_EDGE('',*,*,#24501,.F.);
#36002=ORIENTED_EDGE('',*,*,#24499,.F.);
#36003=ORIENTED_EDGE('',*,*,#24522,.T.);
#36004=ORIENTED_EDGE('',*,*,#24523,.T.);
#36005=ORIENTED_EDGE('',*,*,#24524,.T.);
#36006=ORIENTED_EDGE('',*,*,#24508,.T.);
#36007=ORIENTED_EDGE('',*,*,#24523,.F.);
#36008=ORIENTED_EDGE('',*,*,#24525,.F.);
#36009=ORIENTED_EDGE('',*,*,#24526,.T.);
#36010=ORIENTED_EDGE('',*,*,#24527,.T.);
#36011=ORIENTED_EDGE('',*,*,#24528,.T.);
#36012=ORIENTED_EDGE('',*,*,#24517,.T.);
#36013=ORIENTED_EDGE('',*,*,#24527,.F.);
#36014=ORIENTED_EDGE('',*,*,#24529,.F.);
#36015=ORIENTED_EDGE('',*,*,#24510,.T.);
#36016=ORIENTED_EDGE('',*,*,#24530,.T.);
#36017=ORIENTED_EDGE('',*,*,#24531,.T.);
#36018=ORIENTED_EDGE('',*,*,#24532,.T.);
#36019=ORIENTED_EDGE('',*,*,#24530,.F.);
#36020=ORIENTED_EDGE('',*,*,#24509,.T.);
#36021=ORIENTED_EDGE('',*,*,#24524,.F.);
#36022=ORIENTED_EDGE('',*,*,#24525,.T.);
#36023=ORIENTED_EDGE('',*,*,#24522,.F.);
#36024=ORIENTED_EDGE('',*,*,#24507,.T.);
#36025=ORIENTED_EDGE('',*,*,#24533,.F.);
#36026=ORIENTED_EDGE('',*,*,#24534,.T.);
#36027=ORIENTED_EDGE('',*,*,#24535,.F.);
#36028=ORIENTED_EDGE('',*,*,#24536,.T.);
#36029=ORIENTED_EDGE('',*,*,#24537,.F.);
#36030=ORIENTED_EDGE('',*,*,#24538,.T.);
#36031=ORIENTED_EDGE('',*,*,#24539,.T.);
#36032=ORIENTED_EDGE('',*,*,#24540,.T.);
#36033=ORIENTED_EDGE('',*,*,#24541,.T.);
#36034=ORIENTED_EDGE('',*,*,#24540,.F.);
#36035=ORIENTED_EDGE('',*,*,#24541,.F.);
#36036=ORIENTED_EDGE('',*,*,#24542,.T.);
#36037=ORIENTED_EDGE('',*,*,#24543,.F.);
#36038=ORIENTED_EDGE('',*,*,#24544,.F.);
#36039=ORIENTED_EDGE('',*,*,#24545,.F.);
#36040=ORIENTED_EDGE('',*,*,#24546,.F.);
#36041=ORIENTED_EDGE('',*,*,#24547,.F.);
#36042=ORIENTED_EDGE('',*,*,#24548,.F.);
#36043=ORIENTED_EDGE('',*,*,#24549,.F.);
#36044=ORIENTED_EDGE('',*,*,#24550,.F.);
#36045=ORIENTED_EDGE('',*,*,#24551,.F.);
#36046=ORIENTED_EDGE('',*,*,#24552,.F.);
#36047=ORIENTED_EDGE('',*,*,#24553,.F.);
#36048=ORIENTED_EDGE('',*,*,#24531,.F.);
#36049=ORIENTED_EDGE('',*,*,#24538,.F.);
#36050=ORIENTED_EDGE('',*,*,#24554,.F.);
#36051=ORIENTED_EDGE('',*,*,#24534,.F.);
#36052=ORIENTED_EDGE('',*,*,#24555,.F.);
#36053=ORIENTED_EDGE('',*,*,#24556,.F.);
#36054=ORIENTED_EDGE('',*,*,#24557,.F.);
#36055=ORIENTED_EDGE('',*,*,#24542,.F.);
#36056=ORIENTED_EDGE('',*,*,#24539,.F.);
#36057=ORIENTED_EDGE('',*,*,#24537,.T.);
#36058=ORIENTED_EDGE('',*,*,#24558,.T.);
#36059=ORIENTED_EDGE('',*,*,#24535,.T.);
#36060=ORIENTED_EDGE('',*,*,#24554,.T.);
#36061=ORIENTED_EDGE('',*,*,#24558,.F.);
#36062=ORIENTED_EDGE('',*,*,#24536,.F.);
#36063=ORIENTED_EDGE('',*,*,#24559,.T.);
#36064=ORIENTED_EDGE('',*,*,#24560,.T.);
#36065=ORIENTED_EDGE('',*,*,#24561,.T.);
#36066=ORIENTED_EDGE('',*,*,#24547,.T.);
#36067=ORIENTED_EDGE('',*,*,#24560,.F.);
#36068=ORIENTED_EDGE('',*,*,#24562,.F.);
#36069=ORIENTED_EDGE('',*,*,#24563,.T.);
#36070=ORIENTED_EDGE('',*,*,#24564,.T.);
#36071=ORIENTED_EDGE('',*,*,#24565,.T.);
#36072=ORIENTED_EDGE('',*,*,#24566,.T.);
#36073=ORIENTED_EDGE('',*,*,#24564,.F.);
#36074=ORIENTED_EDGE('',*,*,#24566,.F.);
#36075=ORIENTED_EDGE('',*,*,#24567,.T.);
#36076=ORIENTED_EDGE('',*,*,#24568,.F.);
#36077=ORIENTED_EDGE('',*,*,#24569,.F.);
#36078=ORIENTED_EDGE('',*,*,#24570,.F.);
#36079=ORIENTED_EDGE('',*,*,#24571,.F.);
#36080=ORIENTED_EDGE('',*,*,#24572,.F.);
#36081=ORIENTED_EDGE('',*,*,#24573,.F.);
#36082=ORIENTED_EDGE('',*,*,#24574,.F.);
#36083=ORIENTED_EDGE('',*,*,#24575,.F.);
#36084=ORIENTED_EDGE('',*,*,#24576,.F.);
#36085=ORIENTED_EDGE('',*,*,#24577,.F.);
#36086=ORIENTED_EDGE('',*,*,#24578,.F.);
#36087=ORIENTED_EDGE('',*,*,#24579,.F.);
#36088=ORIENTED_EDGE('',*,*,#24580,.F.);
#36089=ORIENTED_EDGE('',*,*,#24581,.F.);
#36090=ORIENTED_EDGE('',*,*,#24582,.F.);
#36091=ORIENTED_EDGE('',*,*,#24583,.F.);
#36092=ORIENTED_EDGE('',*,*,#24584,.F.);
#36093=ORIENTED_EDGE('',*,*,#24585,.F.);
#36094=ORIENTED_EDGE('',*,*,#24567,.F.);
#36095=ORIENTED_EDGE('',*,*,#24565,.F.);
#36096=ORIENTED_EDGE('',*,*,#24563,.F.);
#36097=ORIENTED_EDGE('',*,*,#24586,.T.);
#36098=ORIENTED_EDGE('',*,*,#24587,.T.);
#36099=ORIENTED_EDGE('',*,*,#24588,.T.);
#36100=ORIENTED_EDGE('',*,*,#24572,.T.);
#36101=ORIENTED_EDGE('',*,*,#24587,.F.);
#36102=ORIENTED_EDGE('',*,*,#24589,.F.);
#36103=ORIENTED_EDGE('',*,*,#24590,.T.);
#36104=ORIENTED_EDGE('',*,*,#24591,.T.);
#36105=ORIENTED_EDGE('',*,*,#24592,.T.);
#36106=ORIENTED_EDGE('',*,*,#24581,.T.);
#36107=ORIENTED_EDGE('',*,*,#24591,.F.);
#36108=ORIENTED_EDGE('',*,*,#24593,.F.);
#36109=ORIENTED_EDGE('',*,*,#24594,.T.);
#36110=ORIENTED_EDGE('',*,*,#24595,.T.);
#36111=ORIENTED_EDGE('',*,*,#24596,.T.);
#36112=ORIENTED_EDGE('',*,*,#24597,.T.);
#36113=ORIENTED_EDGE('',*,*,#24595,.F.);
#36114=ORIENTED_EDGE('',*,*,#24598,.F.);
#36115=ORIENTED_EDGE('',*,*,#24599,.F.);
#36116=ORIENTED_EDGE('',*,*,#24600,.T.);
#36117=ORIENTED_EDGE('',*,*,#24601,.F.);
#36118=ORIENTED_EDGE('',*,*,#24602,.F.);
#36119=ORIENTED_EDGE('',*,*,#24603,.F.);
#36120=ORIENTED_EDGE('',*,*,#24604,.F.);
#36121=ORIENTED_EDGE('',*,*,#24605,.F.);
#36122=ORIENTED_EDGE('',*,*,#24606,.F.);
#36123=ORIENTED_EDGE('',*,*,#24607,.F.);
#36124=ORIENTED_EDGE('',*,*,#24608,.F.);
#36125=ORIENTED_EDGE('',*,*,#24609,.F.);
#36126=ORIENTED_EDGE('',*,*,#24594,.F.);
#36127=ORIENTED_EDGE('',*,*,#24610,.T.);
#36128=ORIENTED_EDGE('',*,*,#24611,.F.);
#36129=ORIENTED_EDGE('',*,*,#24612,.T.);
#36130=ORIENTED_EDGE('',*,*,#24613,.F.);
#36131=ORIENTED_EDGE('',*,*,#24614,.T.);
#36132=ORIENTED_EDGE('',*,*,#24615,.F.);
#36133=ORIENTED_EDGE('',*,*,#24616,.T.);
#36134=ORIENTED_EDGE('',*,*,#24617,.F.);
#36135=ORIENTED_EDGE('',*,*,#24618,.T.);
#36136=ORIENTED_EDGE('',*,*,#24619,.F.);
#36137=ORIENTED_EDGE('',*,*,#24620,.T.);
#36138=ORIENTED_EDGE('',*,*,#24621,.F.);
#36139=ORIENTED_EDGE('',*,*,#24622,.T.);
#36140=ORIENTED_EDGE('',*,*,#24623,.F.);
#36141=ORIENTED_EDGE('',*,*,#24624,.T.);
#36142=ORIENTED_EDGE('',*,*,#24625,.F.);
#36143=ORIENTED_EDGE('',*,*,#24626,.T.);
#36144=ORIENTED_EDGE('',*,*,#24627,.F.);
#36145=ORIENTED_EDGE('',*,*,#24628,.T.);
#36146=ORIENTED_EDGE('',*,*,#24629,.F.);
#36147=ORIENTED_EDGE('',*,*,#24630,.T.);
#36148=ORIENTED_EDGE('',*,*,#24631,.F.);
#36149=ORIENTED_EDGE('',*,*,#24632,.T.);
#36150=ORIENTED_EDGE('',*,*,#24633,.F.);
#36151=ORIENTED_EDGE('',*,*,#24634,.T.);
#36152=ORIENTED_EDGE('',*,*,#24635,.F.);
#36153=ORIENTED_EDGE('',*,*,#24636,.T.);
#36154=ORIENTED_EDGE('',*,*,#24637,.F.);
#36155=ORIENTED_EDGE('',*,*,#24638,.T.);
#36156=ORIENTED_EDGE('',*,*,#24639,.F.);
#36157=ORIENTED_EDGE('',*,*,#24640,.T.);
#36158=ORIENTED_EDGE('',*,*,#24641,.F.);
#36159=ORIENTED_EDGE('',*,*,#24642,.T.);
#36160=ORIENTED_EDGE('',*,*,#24643,.F.);
#36161=ORIENTED_EDGE('',*,*,#24644,.T.);
#36162=ORIENTED_EDGE('',*,*,#24645,.F.);
#36163=ORIENTED_EDGE('',*,*,#24646,.T.);
#36164=ORIENTED_EDGE('',*,*,#24647,.F.);
#36165=ORIENTED_EDGE('',*,*,#24648,.T.);
#36166=ORIENTED_EDGE('',*,*,#24649,.F.);
#36167=ORIENTED_EDGE('',*,*,#24650,.T.);
#36168=ORIENTED_EDGE('',*,*,#24651,.F.);
#36169=ORIENTED_EDGE('',*,*,#24652,.T.);
#36170=ORIENTED_EDGE('',*,*,#24653,.F.);
#36171=ORIENTED_EDGE('',*,*,#24654,.T.);
#36172=ORIENTED_EDGE('',*,*,#24655,.F.);
#36173=ORIENTED_EDGE('',*,*,#24656,.T.);
#36174=ORIENTED_EDGE('',*,*,#24657,.F.);
#36175=ORIENTED_EDGE('',*,*,#24658,.T.);
#36176=ORIENTED_EDGE('',*,*,#24659,.F.);
#36177=ORIENTED_EDGE('',*,*,#24660,.T.);
#36178=ORIENTED_EDGE('',*,*,#24661,.F.);
#36179=ORIENTED_EDGE('',*,*,#24662,.T.);
#36180=ORIENTED_EDGE('',*,*,#24663,.F.);
#36181=ORIENTED_EDGE('',*,*,#24664,.T.);
#36182=ORIENTED_EDGE('',*,*,#24665,.F.);
#36183=ORIENTED_EDGE('',*,*,#24666,.T.);
#36184=ORIENTED_EDGE('',*,*,#24667,.F.);
#36185=ORIENTED_EDGE('',*,*,#24668,.T.);
#36186=ORIENTED_EDGE('',*,*,#24669,.F.);
#36187=ORIENTED_EDGE('',*,*,#24670,.T.);
#36188=ORIENTED_EDGE('',*,*,#24671,.F.);
#36189=ORIENTED_EDGE('',*,*,#24672,.T.);
#36190=ORIENTED_EDGE('',*,*,#24673,.F.);
#36191=ORIENTED_EDGE('',*,*,#24674,.T.);
#36192=ORIENTED_EDGE('',*,*,#24675,.F.);
#36193=ORIENTED_EDGE('',*,*,#24676,.T.);
#36194=ORIENTED_EDGE('',*,*,#24677,.F.);
#36195=ORIENTED_EDGE('',*,*,#24678,.T.);
#36196=ORIENTED_EDGE('',*,*,#24679,.F.);
#36197=ORIENTED_EDGE('',*,*,#24680,.T.);
#36198=ORIENTED_EDGE('',*,*,#24681,.F.);
#36199=ORIENTED_EDGE('',*,*,#24682,.T.);
#36200=ORIENTED_EDGE('',*,*,#24683,.F.);
#36201=ORIENTED_EDGE('',*,*,#24684,.T.);
#36202=ORIENTED_EDGE('',*,*,#24685,.F.);
#36203=ORIENTED_EDGE('',*,*,#24686,.T.);
#36204=ORIENTED_EDGE('',*,*,#24687,.F.);
#36205=ORIENTED_EDGE('',*,*,#24688,.T.);
#36206=ORIENTED_EDGE('',*,*,#24689,.F.);
#36207=ORIENTED_EDGE('',*,*,#24690,.T.);
#36208=ORIENTED_EDGE('',*,*,#24691,.F.);
#36209=ORIENTED_EDGE('',*,*,#24692,.T.);
#36210=ORIENTED_EDGE('',*,*,#24693,.F.);
#36211=ORIENTED_EDGE('',*,*,#24694,.T.);
#36212=ORIENTED_EDGE('',*,*,#24695,.F.);
#36213=ORIENTED_EDGE('',*,*,#24696,.T.);
#36214=ORIENTED_EDGE('',*,*,#24697,.F.);
#36215=ORIENTED_EDGE('',*,*,#24698,.T.);
#36216=ORIENTED_EDGE('',*,*,#24699,.F.);
#36217=ORIENTED_EDGE('',*,*,#24700,.T.);
#36218=ORIENTED_EDGE('',*,*,#24701,.F.);
#36219=ORIENTED_EDGE('',*,*,#24702,.T.);
#36220=ORIENTED_EDGE('',*,*,#24703,.F.);
#36221=ORIENTED_EDGE('',*,*,#24704,.T.);
#36222=ORIENTED_EDGE('',*,*,#24705,.F.);
#36223=ORIENTED_EDGE('',*,*,#24706,.T.);
#36224=ORIENTED_EDGE('',*,*,#24707,.F.);
#36225=ORIENTED_EDGE('',*,*,#24708,.T.);
#36226=ORIENTED_EDGE('',*,*,#24709,.F.);
#36227=ORIENTED_EDGE('',*,*,#24710,.T.);
#36228=ORIENTED_EDGE('',*,*,#24711,.F.);
#36229=ORIENTED_EDGE('',*,*,#24712,.T.);
#36230=ORIENTED_EDGE('',*,*,#24713,.F.);
#36231=ORIENTED_EDGE('',*,*,#24714,.T.);
#36232=ORIENTED_EDGE('',*,*,#24715,.F.);
#36233=ORIENTED_EDGE('',*,*,#24716,.T.);
#36234=ORIENTED_EDGE('',*,*,#24717,.F.);
#36235=ORIENTED_EDGE('',*,*,#24718,.T.);
#36236=ORIENTED_EDGE('',*,*,#24719,.F.);
#36237=ORIENTED_EDGE('',*,*,#24720,.T.);
#36238=ORIENTED_EDGE('',*,*,#24721,.F.);
#36239=ORIENTED_EDGE('',*,*,#24722,.T.);
#36240=ORIENTED_EDGE('',*,*,#24723,.F.);
#36241=ORIENTED_EDGE('',*,*,#24724,.T.);
#36242=ORIENTED_EDGE('',*,*,#24725,.F.);
#36243=ORIENTED_EDGE('',*,*,#24726,.T.);
#36244=ORIENTED_EDGE('',*,*,#24727,.F.);
#36245=ORIENTED_EDGE('',*,*,#24728,.T.);
#36246=ORIENTED_EDGE('',*,*,#24729,.F.);
#36247=ORIENTED_EDGE('',*,*,#24730,.T.);
#36248=ORIENTED_EDGE('',*,*,#24731,.F.);
#36249=ORIENTED_EDGE('',*,*,#24732,.T.);
#36250=ORIENTED_EDGE('',*,*,#24733,.F.);
#36251=ORIENTED_EDGE('',*,*,#24734,.T.);
#36252=ORIENTED_EDGE('',*,*,#24735,.F.);
#36253=ORIENTED_EDGE('',*,*,#24736,.T.);
#36254=ORIENTED_EDGE('',*,*,#24737,.F.);
#36255=ORIENTED_EDGE('',*,*,#24738,.T.);
#36256=ORIENTED_EDGE('',*,*,#24739,.F.);
#36257=ORIENTED_EDGE('',*,*,#24740,.T.);
#36258=ORIENTED_EDGE('',*,*,#24741,.F.);
#36259=ORIENTED_EDGE('',*,*,#24742,.T.);
#36260=ORIENTED_EDGE('',*,*,#24743,.F.);
#36261=ORIENTED_EDGE('',*,*,#24744,.T.);
#36262=ORIENTED_EDGE('',*,*,#24745,.F.);
#36263=ORIENTED_EDGE('',*,*,#24746,.T.);
#36264=ORIENTED_EDGE('',*,*,#24747,.F.);
#36265=ORIENTED_EDGE('',*,*,#24748,.T.);
#36266=ORIENTED_EDGE('',*,*,#24749,.F.);
#36267=ORIENTED_EDGE('',*,*,#24750,.T.);
#36268=ORIENTED_EDGE('',*,*,#24751,.F.);
#36269=ORIENTED_EDGE('',*,*,#24598,.T.);
#36270=ORIENTED_EDGE('',*,*,#24611,.T.);
#36271=ORIENTED_EDGE('',*,*,#24752,.T.);
#36272=ORIENTED_EDGE('',*,*,#24753,.T.);
#36273=ORIENTED_EDGE('',*,*,#24754,.T.);
#36274=ORIENTED_EDGE('',*,*,#24754,.F.);
#36275=ORIENTED_EDGE('',*,*,#24755,.T.);
#36276=ORIENTED_EDGE('',*,*,#24756,.F.);
#36277=ORIENTED_EDGE('',*,*,#24612,.F.);
#36278=ORIENTED_EDGE('',*,*,#24757,.F.);
#36279=ORIENTED_EDGE('',*,*,#24758,.F.);
#36280=ORIENTED_EDGE('',*,*,#24759,.F.);
#36281=ORIENTED_EDGE('',*,*,#24760,.F.);
#36282=ORIENTED_EDGE('',*,*,#24761,.F.);
#36283=ORIENTED_EDGE('',*,*,#24762,.F.);
#36284=ORIENTED_EDGE('',*,*,#24763,.F.);
#36285=ORIENTED_EDGE('',*,*,#24764,.F.);
#36286=ORIENTED_EDGE('',*,*,#24765,.F.);
#36287=ORIENTED_EDGE('',*,*,#24596,.F.);
#36288=ORIENTED_EDGE('',*,*,#24600,.F.);
#36289=ORIENTED_EDGE('',*,*,#24766,.T.);
#36290=ORIENTED_EDGE('',*,*,#24767,.F.);
#36291=ORIENTED_EDGE('',*,*,#24768,.F.);
#36292=ORIENTED_EDGE('',*,*,#24769,.F.);
#36293=ORIENTED_EDGE('',*,*,#24770,.F.);
#36294=ORIENTED_EDGE('',*,*,#24771,.F.);
#36295=ORIENTED_EDGE('',*,*,#24772,.T.);
#36296=ORIENTED_EDGE('',*,*,#24773,.F.);
#36297=ORIENTED_EDGE('',*,*,#24774,.F.);
#36298=ORIENTED_EDGE('',*,*,#24775,.F.);
#36299=ORIENTED_EDGE('',*,*,#24776,.F.);
#36300=ORIENTED_EDGE('',*,*,#24777,.F.);
#36301=ORIENTED_EDGE('',*,*,#24778,.T.);
#36302=ORIENTED_EDGE('',*,*,#24779,.F.);
#36303=ORIENTED_EDGE('',*,*,#24780,.F.);
#36304=ORIENTED_EDGE('',*,*,#24781,.F.);
#36305=ORIENTED_EDGE('',*,*,#24782,.F.);
#36306=ORIENTED_EDGE('',*,*,#24783,.F.);
#36307=ORIENTED_EDGE('',*,*,#24784,.T.);
#36308=ORIENTED_EDGE('',*,*,#24785,.F.);
#36309=ORIENTED_EDGE('',*,*,#24786,.F.);
#36310=ORIENTED_EDGE('',*,*,#24787,.F.);
#36311=ORIENTED_EDGE('',*,*,#24788,.F.);
#36312=ORIENTED_EDGE('',*,*,#24789,.F.);
#36313=ORIENTED_EDGE('',*,*,#24790,.T.);
#36314=ORIENTED_EDGE('',*,*,#24791,.F.);
#36315=ORIENTED_EDGE('',*,*,#24792,.F.);
#36316=ORIENTED_EDGE('',*,*,#24793,.F.);
#36317=ORIENTED_EDGE('',*,*,#24794,.F.);
#36318=ORIENTED_EDGE('',*,*,#24795,.F.);
#36319=ORIENTED_EDGE('',*,*,#24796,.T.);
#36320=ORIENTED_EDGE('',*,*,#24797,.F.);
#36321=ORIENTED_EDGE('',*,*,#24798,.F.);
#36322=ORIENTED_EDGE('',*,*,#24799,.F.);
#36323=ORIENTED_EDGE('',*,*,#24800,.F.);
#36324=ORIENTED_EDGE('',*,*,#24801,.F.);
#36325=ORIENTED_EDGE('',*,*,#24802,.T.);
#36326=ORIENTED_EDGE('',*,*,#24803,.F.);
#36327=ORIENTED_EDGE('',*,*,#24804,.F.);
#36328=ORIENTED_EDGE('',*,*,#24805,.F.);
#36329=ORIENTED_EDGE('',*,*,#24806,.F.);
#36330=ORIENTED_EDGE('',*,*,#24807,.F.);
#36331=ORIENTED_EDGE('',*,*,#24808,.T.);
#36332=ORIENTED_EDGE('',*,*,#24809,.F.);
#36333=ORIENTED_EDGE('',*,*,#24810,.F.);
#36334=ORIENTED_EDGE('',*,*,#24811,.F.);
#36335=ORIENTED_EDGE('',*,*,#24812,.F.);
#36336=ORIENTED_EDGE('',*,*,#24813,.F.);
#36337=ORIENTED_EDGE('',*,*,#24814,.T.);
#36338=ORIENTED_EDGE('',*,*,#24815,.F.);
#36339=ORIENTED_EDGE('',*,*,#24816,.F.);
#36340=ORIENTED_EDGE('',*,*,#24817,.F.);
#36341=ORIENTED_EDGE('',*,*,#24818,.F.);
#36342=ORIENTED_EDGE('',*,*,#24819,.F.);
#36343=ORIENTED_EDGE('',*,*,#24820,.T.);
#36344=ORIENTED_EDGE('',*,*,#24821,.F.);
#36345=ORIENTED_EDGE('',*,*,#24822,.F.);
#36346=ORIENTED_EDGE('',*,*,#24823,.F.);
#36347=ORIENTED_EDGE('',*,*,#24824,.F.);
#36348=ORIENTED_EDGE('',*,*,#24825,.F.);
#36349=ORIENTED_EDGE('',*,*,#24826,.T.);
#36350=ORIENTED_EDGE('',*,*,#24827,.F.);
#36351=ORIENTED_EDGE('',*,*,#24828,.F.);
#36352=ORIENTED_EDGE('',*,*,#24829,.F.);
#36353=ORIENTED_EDGE('',*,*,#24830,.F.);
#36354=ORIENTED_EDGE('',*,*,#24831,.F.);
#36355=ORIENTED_EDGE('',*,*,#24832,.T.);
#36356=ORIENTED_EDGE('',*,*,#24833,.F.);
#36357=ORIENTED_EDGE('',*,*,#24834,.F.);
#36358=ORIENTED_EDGE('',*,*,#24835,.F.);
#36359=ORIENTED_EDGE('',*,*,#24836,.F.);
#36360=ORIENTED_EDGE('',*,*,#24837,.F.);
#36361=ORIENTED_EDGE('',*,*,#24838,.T.);
#36362=ORIENTED_EDGE('',*,*,#24839,.F.);
#36363=ORIENTED_EDGE('',*,*,#24840,.F.);
#36364=ORIENTED_EDGE('',*,*,#24841,.F.);
#36365=ORIENTED_EDGE('',*,*,#24842,.F.);
#36366=ORIENTED_EDGE('',*,*,#24843,.F.);
#36367=ORIENTED_EDGE('',*,*,#24844,.T.);
#36368=ORIENTED_EDGE('',*,*,#24845,.F.);
#36369=ORIENTED_EDGE('',*,*,#24846,.F.);
#36370=ORIENTED_EDGE('',*,*,#24847,.F.);
#36371=ORIENTED_EDGE('',*,*,#24848,.F.);
#36372=ORIENTED_EDGE('',*,*,#24849,.F.);
#36373=ORIENTED_EDGE('',*,*,#24850,.T.);
#36374=ORIENTED_EDGE('',*,*,#24851,.F.);
#36375=ORIENTED_EDGE('',*,*,#24852,.F.);
#36376=ORIENTED_EDGE('',*,*,#24853,.F.);
#36377=ORIENTED_EDGE('',*,*,#24854,.F.);
#36378=ORIENTED_EDGE('',*,*,#24855,.F.);
#36379=ORIENTED_EDGE('',*,*,#24856,.T.);
#36380=ORIENTED_EDGE('',*,*,#24857,.F.);
#36381=ORIENTED_EDGE('',*,*,#24858,.F.);
#36382=ORIENTED_EDGE('',*,*,#24859,.F.);
#36383=ORIENTED_EDGE('',*,*,#24860,.F.);
#36384=ORIENTED_EDGE('',*,*,#24861,.F.);
#36385=ORIENTED_EDGE('',*,*,#24862,.T.);
#36386=ORIENTED_EDGE('',*,*,#24863,.F.);
#36387=ORIENTED_EDGE('',*,*,#24864,.F.);
#36388=ORIENTED_EDGE('',*,*,#24865,.F.);
#36389=ORIENTED_EDGE('',*,*,#24866,.F.);
#36390=ORIENTED_EDGE('',*,*,#24867,.F.);
#36391=ORIENTED_EDGE('',*,*,#24868,.T.);
#36392=ORIENTED_EDGE('',*,*,#24869,.F.);
#36393=ORIENTED_EDGE('',*,*,#24870,.F.);
#36394=ORIENTED_EDGE('',*,*,#24871,.F.);
#36395=ORIENTED_EDGE('',*,*,#24872,.F.);
#36396=ORIENTED_EDGE('',*,*,#24873,.F.);
#36397=ORIENTED_EDGE('',*,*,#24874,.T.);
#36398=ORIENTED_EDGE('',*,*,#24875,.F.);
#36399=ORIENTED_EDGE('',*,*,#24876,.F.);
#36400=ORIENTED_EDGE('',*,*,#24877,.F.);
#36401=ORIENTED_EDGE('',*,*,#24878,.F.);
#36402=ORIENTED_EDGE('',*,*,#24879,.F.);
#36403=ORIENTED_EDGE('',*,*,#24880,.T.);
#36404=ORIENTED_EDGE('',*,*,#24881,.F.);
#36405=ORIENTED_EDGE('',*,*,#24882,.F.);
#36406=ORIENTED_EDGE('',*,*,#24883,.F.);
#36407=ORIENTED_EDGE('',*,*,#24884,.F.);
#36408=ORIENTED_EDGE('',*,*,#24885,.F.);
#36409=ORIENTED_EDGE('',*,*,#24886,.T.);
#36410=ORIENTED_EDGE('',*,*,#24887,.F.);
#36411=ORIENTED_EDGE('',*,*,#24888,.F.);
#36412=ORIENTED_EDGE('',*,*,#24889,.F.);
#36413=ORIENTED_EDGE('',*,*,#24890,.F.);
#36414=ORIENTED_EDGE('',*,*,#24891,.F.);
#36415=ORIENTED_EDGE('',*,*,#24892,.T.);
#36416=ORIENTED_EDGE('',*,*,#24893,.F.);
#36417=ORIENTED_EDGE('',*,*,#24894,.F.);
#36418=ORIENTED_EDGE('',*,*,#24895,.F.);
#36419=ORIENTED_EDGE('',*,*,#24896,.F.);
#36420=ORIENTED_EDGE('',*,*,#24897,.F.);
#36421=ORIENTED_EDGE('',*,*,#24898,.T.);
#36422=ORIENTED_EDGE('',*,*,#24899,.F.);
#36423=ORIENTED_EDGE('',*,*,#24900,.F.);
#36424=ORIENTED_EDGE('',*,*,#24901,.F.);
#36425=ORIENTED_EDGE('',*,*,#24902,.F.);
#36426=ORIENTED_EDGE('',*,*,#24903,.F.);
#36427=ORIENTED_EDGE('',*,*,#24904,.T.);
#36428=ORIENTED_EDGE('',*,*,#24755,.F.);
#36429=ORIENTED_EDGE('',*,*,#24753,.F.);
#36430=ORIENTED_EDGE('',*,*,#24905,.F.);
#36431=ORIENTED_EDGE('',*,*,#24747,.T.);
#36432=ORIENTED_EDGE('',*,*,#24906,.T.);
#36433=ORIENTED_EDGE('',*,*,#24770,.T.);
#36434=ORIENTED_EDGE('',*,*,#24907,.T.);
#36435=ORIENTED_EDGE('',*,*,#24907,.F.);
#36436=ORIENTED_EDGE('',*,*,#24769,.T.);
#36437=ORIENTED_EDGE('',*,*,#24908,.F.);
#36438=ORIENTED_EDGE('',*,*,#24748,.F.);
#36439=ORIENTED_EDGE('',*,*,#24749,.T.);
#36440=ORIENTED_EDGE('',*,*,#24908,.T.);
#36441=ORIENTED_EDGE('',*,*,#24768,.T.);
#36442=ORIENTED_EDGE('',*,*,#24909,.T.);
#36443=ORIENTED_EDGE('',*,*,#24743,.T.);
#36444=ORIENTED_EDGE('',*,*,#24910,.T.);
#36445=ORIENTED_EDGE('',*,*,#24774,.T.);
#36446=ORIENTED_EDGE('',*,*,#24911,.T.);
#36447=ORIENTED_EDGE('',*,*,#24911,.F.);
#36448=ORIENTED_EDGE('',*,*,#24773,.T.);
#36449=ORIENTED_EDGE('',*,*,#24912,.F.);
#36450=ORIENTED_EDGE('',*,*,#24744,.F.);
#36451=ORIENTED_EDGE('',*,*,#24741,.T.);
#36452=ORIENTED_EDGE('',*,*,#24913,.T.);
#36453=ORIENTED_EDGE('',*,*,#24776,.T.);
#36454=ORIENTED_EDGE('',*,*,#24914,.T.);
#36455=ORIENTED_EDGE('',*,*,#24913,.F.);
#36456=ORIENTED_EDGE('',*,*,#24740,.F.);
#36457=ORIENTED_EDGE('',*,*,#24915,.F.);
#36458=ORIENTED_EDGE('',*,*,#24777,.T.);
#36459=ORIENTED_EDGE('',*,*,#24737,.T.);
#36460=ORIENTED_EDGE('',*,*,#24916,.T.);
#36461=ORIENTED_EDGE('',*,*,#24780,.T.);
#36462=ORIENTED_EDGE('',*,*,#24917,.T.);
#36463=ORIENTED_EDGE('',*,*,#24916,.F.);
#36464=ORIENTED_EDGE('',*,*,#24736,.F.);
#36465=ORIENTED_EDGE('',*,*,#24918,.F.);
#36466=ORIENTED_EDGE('',*,*,#24781,.T.);
#36467=ORIENTED_EDGE('',*,*,#24735,.T.);
#36468=ORIENTED_EDGE('',*,*,#24919,.T.);
#36469=ORIENTED_EDGE('',*,*,#24782,.T.);
#36470=ORIENTED_EDGE('',*,*,#24918,.T.);
#36471=ORIENTED_EDGE('',*,*,#24729,.T.);
#36472=ORIENTED_EDGE('',*,*,#24920,.T.);
#36473=ORIENTED_EDGE('',*,*,#24788,.T.);
#36474=ORIENTED_EDGE('',*,*,#24921,.T.);
#36475=ORIENTED_EDGE('',*,*,#24921,.F.);
#36476=ORIENTED_EDGE('',*,*,#24787,.T.);
#36477=ORIENTED_EDGE('',*,*,#24922,.F.);
#36478=ORIENTED_EDGE('',*,*,#24730,.F.);
#36479=ORIENTED_EDGE('',*,*,#24731,.T.);
#36480=ORIENTED_EDGE('',*,*,#24922,.T.);
#36481=ORIENTED_EDGE('',*,*,#24786,.T.);
#36482=ORIENTED_EDGE('',*,*,#24923,.T.);
#36483=ORIENTED_EDGE('',*,*,#24725,.T.);
#36484=ORIENTED_EDGE('',*,*,#24924,.T.);
#36485=ORIENTED_EDGE('',*,*,#24792,.T.);
#36486=ORIENTED_EDGE('',*,*,#24925,.T.);
#36487=ORIENTED_EDGE('',*,*,#24925,.F.);
#36488=ORIENTED_EDGE('',*,*,#24791,.T.);
#36489=ORIENTED_EDGE('',*,*,#24926,.F.);
#36490=ORIENTED_EDGE('',*,*,#24726,.F.);
#36491=ORIENTED_EDGE('',*,*,#24723,.T.);
#36492=ORIENTED_EDGE('',*,*,#24927,.T.);
#36493=ORIENTED_EDGE('',*,*,#24794,.T.);
#36494=ORIENTED_EDGE('',*,*,#24928,.T.);
#36495=ORIENTED_EDGE('',*,*,#24927,.F.);
#36496=ORIENTED_EDGE('',*,*,#24722,.F.);
#36497=ORIENTED_EDGE('',*,*,#24929,.F.);
#36498=ORIENTED_EDGE('',*,*,#24795,.T.);
#36499=ORIENTED_EDGE('',*,*,#24719,.T.);
#36500=ORIENTED_EDGE('',*,*,#24930,.T.);
#36501=ORIENTED_EDGE('',*,*,#24798,.T.);
#36502=ORIENTED_EDGE('',*,*,#24931,.T.);
#36503=ORIENTED_EDGE('',*,*,#24930,.F.);
#36504=ORIENTED_EDGE('',*,*,#24718,.F.);
#36505=ORIENTED_EDGE('',*,*,#24932,.F.);
#36506=ORIENTED_EDGE('',*,*,#24799,.T.);
#36507=ORIENTED_EDGE('',*,*,#24717,.T.);
#36508=ORIENTED_EDGE('',*,*,#24933,.T.);
#36509=ORIENTED_EDGE('',*,*,#24800,.T.);
#36510=ORIENTED_EDGE('',*,*,#24932,.T.);
#36511=ORIENTED_EDGE('',*,*,#24711,.T.);
#36512=ORIENTED_EDGE('',*,*,#24934,.T.);
#36513=ORIENTED_EDGE('',*,*,#24806,.T.);
#36514=ORIENTED_EDGE('',*,*,#24935,.T.);
#36515=ORIENTED_EDGE('',*,*,#24935,.F.);
#36516=ORIENTED_EDGE('',*,*,#24805,.T.);
#36517=ORIENTED_EDGE('',*,*,#24936,.F.);
#36518=ORIENTED_EDGE('',*,*,#24712,.F.);
#36519=ORIENTED_EDGE('',*,*,#24713,.T.);
#36520=ORIENTED_EDGE('',*,*,#24936,.T.);
#36521=ORIENTED_EDGE('',*,*,#24804,.T.);
#36522=ORIENTED_EDGE('',*,*,#24937,.T.);
#36523=ORIENTED_EDGE('',*,*,#24707,.T.);
#36524=ORIENTED_EDGE('',*,*,#24938,.T.);
#36525=ORIENTED_EDGE('',*,*,#24810,.T.);
#36526=ORIENTED_EDGE('',*,*,#24939,.T.);
#36527=ORIENTED_EDGE('',*,*,#24939,.F.);
#36528=ORIENTED_EDGE('',*,*,#24809,.T.);
#36529=ORIENTED_EDGE('',*,*,#24940,.F.);
#36530=ORIENTED_EDGE('',*,*,#24708,.F.);
#36531=ORIENTED_EDGE('',*,*,#24705,.T.);
#36532=ORIENTED_EDGE('',*,*,#24941,.T.);
#36533=ORIENTED_EDGE('',*,*,#24812,.T.);
#36534=ORIENTED_EDGE('',*,*,#24942,.T.);
#36535=ORIENTED_EDGE('',*,*,#24941,.F.);
#36536=ORIENTED_EDGE('',*,*,#24704,.F.);
#36537=ORIENTED_EDGE('',*,*,#24943,.F.);
#36538=ORIENTED_EDGE('',*,*,#24813,.T.);
#36539=ORIENTED_EDGE('',*,*,#24701,.T.);
#36540=ORIENTED_EDGE('',*,*,#24944,.T.);
#36541=ORIENTED_EDGE('',*,*,#24816,.T.);
#36542=ORIENTED_EDGE('',*,*,#24945,.T.);
#36543=ORIENTED_EDGE('',*,*,#24944,.F.);
#36544=ORIENTED_EDGE('',*,*,#24700,.F.);
#36545=ORIENTED_EDGE('',*,*,#24946,.F.);
#36546=ORIENTED_EDGE('',*,*,#24817,.T.);
#36547=ORIENTED_EDGE('',*,*,#24699,.T.);
#36548=ORIENTED_EDGE('',*,*,#24947,.T.);
#36549=ORIENTED_EDGE('',*,*,#24818,.T.);
#36550=ORIENTED_EDGE('',*,*,#24946,.T.);
#36551=ORIENTED_EDGE('',*,*,#24693,.T.);
#36552=ORIENTED_EDGE('',*,*,#24948,.T.);
#36553=ORIENTED_EDGE('',*,*,#24824,.T.);
#36554=ORIENTED_EDGE('',*,*,#24949,.T.);
#36555=ORIENTED_EDGE('',*,*,#24949,.F.);
#36556=ORIENTED_EDGE('',*,*,#24823,.T.);
#36557=ORIENTED_EDGE('',*,*,#24950,.F.);
#36558=ORIENTED_EDGE('',*,*,#24694,.F.);
#36559=ORIENTED_EDGE('',*,*,#24695,.T.);
#36560=ORIENTED_EDGE('',*,*,#24950,.T.);
#36561=ORIENTED_EDGE('',*,*,#24822,.T.);
#36562=ORIENTED_EDGE('',*,*,#24951,.T.);
#36563=ORIENTED_EDGE('',*,*,#24689,.T.);
#36564=ORIENTED_EDGE('',*,*,#24952,.T.);
#36565=ORIENTED_EDGE('',*,*,#24828,.T.);
#36566=ORIENTED_EDGE('',*,*,#24953,.T.);
#36567=ORIENTED_EDGE('',*,*,#24953,.F.);
#36568=ORIENTED_EDGE('',*,*,#24827,.T.);
#36569=ORIENTED_EDGE('',*,*,#24954,.F.);
#36570=ORIENTED_EDGE('',*,*,#24690,.F.);
#36571=ORIENTED_EDGE('',*,*,#24687,.T.);
#36572=ORIENTED_EDGE('',*,*,#24955,.T.);
#36573=ORIENTED_EDGE('',*,*,#24830,.T.);
#36574=ORIENTED_EDGE('',*,*,#24956,.T.);
#36575=ORIENTED_EDGE('',*,*,#24955,.F.);
#36576=ORIENTED_EDGE('',*,*,#24686,.F.);
#36577=ORIENTED_EDGE('',*,*,#24957,.F.);
#36578=ORIENTED_EDGE('',*,*,#24831,.T.);
#36579=ORIENTED_EDGE('',*,*,#24683,.T.);
#36580=ORIENTED_EDGE('',*,*,#24958,.T.);
#36581=ORIENTED_EDGE('',*,*,#24834,.T.);
#36582=ORIENTED_EDGE('',*,*,#24959,.T.);
#36583=ORIENTED_EDGE('',*,*,#24958,.F.);
#36584=ORIENTED_EDGE('',*,*,#24682,.F.);
#36585=ORIENTED_EDGE('',*,*,#24960,.F.);
#36586=ORIENTED_EDGE('',*,*,#24835,.T.);
#36587=ORIENTED_EDGE('',*,*,#24681,.T.);
#36588=ORIENTED_EDGE('',*,*,#24961,.T.);
#36589=ORIENTED_EDGE('',*,*,#24836,.T.);
#36590=ORIENTED_EDGE('',*,*,#24960,.T.);
#36591=ORIENTED_EDGE('',*,*,#24675,.T.);
#36592=ORIENTED_EDGE('',*,*,#24962,.T.);
#36593=ORIENTED_EDGE('',*,*,#24842,.T.);
#36594=ORIENTED_EDGE('',*,*,#24963,.T.);
#36595=ORIENTED_EDGE('',*,*,#24963,.F.);
#36596=ORIENTED_EDGE('',*,*,#24841,.T.);
#36597=ORIENTED_EDGE('',*,*,#24964,.F.);
#36598=ORIENTED_EDGE('',*,*,#24676,.F.);
#36599=ORIENTED_EDGE('',*,*,#24677,.T.);
#36600=ORIENTED_EDGE('',*,*,#24964,.T.);
#36601=ORIENTED_EDGE('',*,*,#24840,.T.);
#36602=ORIENTED_EDGE('',*,*,#24965,.T.);
#36603=ORIENTED_EDGE('',*,*,#24671,.T.);
#36604=ORIENTED_EDGE('',*,*,#24966,.T.);
#36605=ORIENTED_EDGE('',*,*,#24846,.T.);
#36606=ORIENTED_EDGE('',*,*,#24967,.T.);
#36607=ORIENTED_EDGE('',*,*,#24967,.F.);
#36608=ORIENTED_EDGE('',*,*,#24845,.T.);
#36609=ORIENTED_EDGE('',*,*,#24968,.F.);
#36610=ORIENTED_EDGE('',*,*,#24672,.F.);
#36611=ORIENTED_EDGE('',*,*,#24669,.T.);
#36612=ORIENTED_EDGE('',*,*,#24969,.T.);
#36613=ORIENTED_EDGE('',*,*,#24848,.T.);
#36614=ORIENTED_EDGE('',*,*,#24970,.T.);
#36615=ORIENTED_EDGE('',*,*,#24969,.F.);
#36616=ORIENTED_EDGE('',*,*,#24668,.F.);
#36617=ORIENTED_EDGE('',*,*,#24971,.F.);
#36618=ORIENTED_EDGE('',*,*,#24849,.T.);
#36619=ORIENTED_EDGE('',*,*,#24665,.T.);
#36620=ORIENTED_EDGE('',*,*,#24972,.T.);
#36621=ORIENTED_EDGE('',*,*,#24852,.T.);
#36622=ORIENTED_EDGE('',*,*,#24973,.T.);
#36623=ORIENTED_EDGE('',*,*,#24972,.F.);
#36624=ORIENTED_EDGE('',*,*,#24664,.F.);
#36625=ORIENTED_EDGE('',*,*,#24974,.F.);
#36626=ORIENTED_EDGE('',*,*,#24853,.T.);
#36627=ORIENTED_EDGE('',*,*,#24663,.T.);
#36628=ORIENTED_EDGE('',*,*,#24975,.T.);
#36629=ORIENTED_EDGE('',*,*,#24854,.T.);
#36630=ORIENTED_EDGE('',*,*,#24974,.T.);
#36631=ORIENTED_EDGE('',*,*,#24657,.T.);
#36632=ORIENTED_EDGE('',*,*,#24976,.T.);
#36633=ORIENTED_EDGE('',*,*,#24860,.T.);
#36634=ORIENTED_EDGE('',*,*,#24977,.T.);
#36635=ORIENTED_EDGE('',*,*,#24977,.F.);
#36636=ORIENTED_EDGE('',*,*,#24859,.T.);
#36637=ORIENTED_EDGE('',*,*,#24978,.F.);
#36638=ORIENTED_EDGE('',*,*,#24658,.F.);
#36639=ORIENTED_EDGE('',*,*,#24659,.T.);
#36640=ORIENTED_EDGE('',*,*,#24978,.T.);
#36641=ORIENTED_EDGE('',*,*,#24858,.T.);
#36642=ORIENTED_EDGE('',*,*,#24979,.T.);
#36643=ORIENTED_EDGE('',*,*,#24570,.T.);
#36644=ORIENTED_EDGE('',*,*,#24980,.T.);
#36645=ORIENTED_EDGE('',*,*,#24519,.T.);
#36646=ORIENTED_EDGE('',*,*,#24981,.T.);
#36647=ORIENTED_EDGE('',*,*,#24980,.F.);
#36648=ORIENTED_EDGE('',*,*,#24569,.T.);
#36649=ORIENTED_EDGE('',*,*,#24982,.F.);
#36650=ORIENTED_EDGE('',*,*,#24520,.T.);
#36651=ORIENTED_EDGE('',*,*,#24653,.T.);
#36652=ORIENTED_EDGE('',*,*,#24983,.T.);
#36653=ORIENTED_EDGE('',*,*,#24864,.T.);
#36654=ORIENTED_EDGE('',*,*,#24984,.T.);
#36655=ORIENTED_EDGE('',*,*,#24984,.F.);
#36656=ORIENTED_EDGE('',*,*,#24863,.T.);
#36657=ORIENTED_EDGE('',*,*,#24985,.F.);
#36658=ORIENTED_EDGE('',*,*,#24654,.F.);
#36659=ORIENTED_EDGE('',*,*,#24651,.T.);
#36660=ORIENTED_EDGE('',*,*,#24986,.T.);
#36661=ORIENTED_EDGE('',*,*,#24866,.T.);
#36662=ORIENTED_EDGE('',*,*,#24987,.T.);
#36663=ORIENTED_EDGE('',*,*,#24986,.F.);
#36664=ORIENTED_EDGE('',*,*,#24650,.F.);
#36665=ORIENTED_EDGE('',*,*,#24988,.F.);
#36666=ORIENTED_EDGE('',*,*,#24867,.T.);
#36667=ORIENTED_EDGE('',*,*,#24647,.T.);
#36668=ORIENTED_EDGE('',*,*,#24989,.T.);
#36669=ORIENTED_EDGE('',*,*,#24870,.T.);
#36670=ORIENTED_EDGE('',*,*,#24990,.T.);
#36671=ORIENTED_EDGE('',*,*,#24989,.F.);
#36672=ORIENTED_EDGE('',*,*,#24646,.F.);
#36673=ORIENTED_EDGE('',*,*,#24991,.F.);
#36674=ORIENTED_EDGE('',*,*,#24871,.T.);
#36675=ORIENTED_EDGE('',*,*,#24645,.T.);
#36676=ORIENTED_EDGE('',*,*,#24992,.T.);
#36677=ORIENTED_EDGE('',*,*,#24872,.T.);
#36678=ORIENTED_EDGE('',*,*,#24991,.T.);
#36679=ORIENTED_EDGE('',*,*,#24639,.T.);
#36680=ORIENTED_EDGE('',*,*,#24993,.T.);
#36681=ORIENTED_EDGE('',*,*,#24878,.T.);
#36682=ORIENTED_EDGE('',*,*,#24994,.T.);
#36683=ORIENTED_EDGE('',*,*,#24994,.F.);
#36684=ORIENTED_EDGE('',*,*,#24877,.T.);
#36685=ORIENTED_EDGE('',*,*,#24995,.F.);
#36686=ORIENTED_EDGE('',*,*,#24640,.F.);
#36687=ORIENTED_EDGE('',*,*,#24641,.T.);
#36688=ORIENTED_EDGE('',*,*,#24995,.T.);
#36689=ORIENTED_EDGE('',*,*,#24876,.T.);
#36690=ORIENTED_EDGE('',*,*,#24996,.T.);
#36691=ORIENTED_EDGE('',*,*,#24549,.T.);
#36692=ORIENTED_EDGE('',*,*,#24997,.T.);
#36693=ORIENTED_EDGE('',*,*,#24579,.T.);
#36694=ORIENTED_EDGE('',*,*,#24998,.T.);
#36695=ORIENTED_EDGE('',*,*,#24997,.F.);
#36696=ORIENTED_EDGE('',*,*,#24548,.T.);
#36697=ORIENTED_EDGE('',*,*,#24561,.F.);
#36698=ORIENTED_EDGE('',*,*,#24562,.T.);
#36699=ORIENTED_EDGE('',*,*,#24559,.F.);
#36700=ORIENTED_EDGE('',*,*,#24546,.T.);
#36701=ORIENTED_EDGE('',*,*,#24999,.F.);
#36702=ORIENTED_EDGE('',*,*,#24582,.T.);
#36703=ORIENTED_EDGE('',*,*,#24592,.F.);
#36704=ORIENTED_EDGE('',*,*,#24593,.T.);
#36705=ORIENTED_EDGE('',*,*,#24590,.F.);
#36706=ORIENTED_EDGE('',*,*,#24580,.T.);
#36707=ORIENTED_EDGE('',*,*,#24574,.T.);
#36708=ORIENTED_EDGE('',*,*,#25000,.T.);
#36709=ORIENTED_EDGE('',*,*,#24515,.T.);
#36710=ORIENTED_EDGE('',*,*,#25001,.T.);
#36711=ORIENTED_EDGE('',*,*,#24981,.F.);
#36712=ORIENTED_EDGE('',*,*,#24518,.T.);
#36713=ORIENTED_EDGE('',*,*,#24528,.F.);
#36714=ORIENTED_EDGE('',*,*,#24529,.T.);
#36715=ORIENTED_EDGE('',*,*,#24526,.F.);
#36716=ORIENTED_EDGE('',*,*,#24516,.T.);
#36717=ORIENTED_EDGE('',*,*,#25000,.F.);
#36718=ORIENTED_EDGE('',*,*,#24573,.T.);
#36719=ORIENTED_EDGE('',*,*,#24588,.F.);
#36720=ORIENTED_EDGE('',*,*,#24589,.T.);
#36721=ORIENTED_EDGE('',*,*,#24586,.F.);
#36722=ORIENTED_EDGE('',*,*,#24571,.T.);
#36723=ORIENTED_EDGE('',*,*,#24635,.T.);
#36724=ORIENTED_EDGE('',*,*,#25002,.T.);
#36725=ORIENTED_EDGE('',*,*,#24882,.T.);
#36726=ORIENTED_EDGE('',*,*,#25003,.T.);
#36727=ORIENTED_EDGE('',*,*,#25003,.F.);
#36728=ORIENTED_EDGE('',*,*,#24881,.T.);
#36729=ORIENTED_EDGE('',*,*,#25004,.F.);
#36730=ORIENTED_EDGE('',*,*,#24636,.F.);
#36731=ORIENTED_EDGE('',*,*,#24633,.T.);
#36732=ORIENTED_EDGE('',*,*,#25005,.T.);
#36733=ORIENTED_EDGE('',*,*,#24884,.T.);
#36734=ORIENTED_EDGE('',*,*,#25006,.T.);
#36735=ORIENTED_EDGE('',*,*,#25005,.F.);
#36736=ORIENTED_EDGE('',*,*,#24632,.F.);
#36737=ORIENTED_EDGE('',*,*,#25007,.F.);
#36738=ORIENTED_EDGE('',*,*,#24885,.T.);
#36739=ORIENTED_EDGE('',*,*,#24545,.T.);
#36740=ORIENTED_EDGE('',*,*,#25008,.T.);
#36741=ORIENTED_EDGE('',*,*,#24583,.T.);
#36742=ORIENTED_EDGE('',*,*,#24999,.T.);
#36743=ORIENTED_EDGE('',*,*,#25008,.F.);
#36744=ORIENTED_EDGE('',*,*,#24544,.T.);
#36745=ORIENTED_EDGE('',*,*,#25009,.F.);
#36746=ORIENTED_EDGE('',*,*,#24584,.T.);
#36747=ORIENTED_EDGE('',*,*,#24506,.T.);
#36748=ORIENTED_EDGE('',*,*,#25010,.T.);
#36749=ORIENTED_EDGE('',*,*,#24555,.T.);
#36750=ORIENTED_EDGE('',*,*,#24533,.T.);
#36751=ORIENTED_EDGE('',*,*,#25010,.F.);
#36752=ORIENTED_EDGE('',*,*,#24505,.T.);
#36753=ORIENTED_EDGE('',*,*,#25011,.F.);
#36754=ORIENTED_EDGE('',*,*,#24556,.T.);
#36755=ORIENTED_EDGE('',*,*,#25012,.T.);
#36756=ORIENTED_EDGE('',*,*,#25013,.T.);
#36757=ORIENTED_EDGE('',*,*,#25014,.T.);
#36758=ORIENTED_EDGE('',*,*,#24608,.T.);
#36759=ORIENTED_EDGE('',*,*,#25012,.F.);
#36760=ORIENTED_EDGE('',*,*,#24607,.T.);
#36761=ORIENTED_EDGE('',*,*,#24512,.T.);
#36762=ORIENTED_EDGE('',*,*,#25014,.F.);
#36763=ORIENTED_EDGE('',*,*,#24552,.T.);
#36764=ORIENTED_EDGE('',*,*,#24609,.T.);
#36765=ORIENTED_EDGE('',*,*,#25015,.T.);
#36766=ORIENTED_EDGE('',*,*,#25016,.T.);
#36767=ORIENTED_EDGE('',*,*,#25017,.T.);
#36768=ORIENTED_EDGE('',*,*,#24605,.T.);
#36769=ORIENTED_EDGE('',*,*,#25015,.F.);
#36770=ORIENTED_EDGE('',*,*,#24604,.T.);
#36771=ORIENTED_EDGE('',*,*,#24576,.T.);
#36772=ORIENTED_EDGE('',*,*,#25017,.F.);
#36773=ORIENTED_EDGE('',*,*,#24513,.T.);
#36774=ORIENTED_EDGE('',*,*,#24606,.T.);
#36775=ORIENTED_EDGE('',*,*,#25018,.T.);
#36776=ORIENTED_EDGE('',*,*,#25019,.T.);
#36777=ORIENTED_EDGE('',*,*,#25020,.T.);
#36778=ORIENTED_EDGE('',*,*,#24602,.T.);
#36779=ORIENTED_EDGE('',*,*,#25018,.F.);
#36780=ORIENTED_EDGE('',*,*,#24601,.T.);
#36781=ORIENTED_EDGE('',*,*,#24551,.T.);
#36782=ORIENTED_EDGE('',*,*,#25020,.F.);
#36783=ORIENTED_EDGE('',*,*,#24577,.T.);
#36784=ORIENTED_EDGE('',*,*,#24603,.T.);
#36785=ORIENTED_EDGE('',*,*,#25001,.F.);
#36786=ORIENTED_EDGE('',*,*,#24514,.T.);
#36787=ORIENTED_EDGE('',*,*,#25016,.F.);
#36788=ORIENTED_EDGE('',*,*,#24575,.T.);
#36789=ORIENTED_EDGE('',*,*,#24998,.F.);
#36790=ORIENTED_EDGE('',*,*,#24578,.T.);
#36791=ORIENTED_EDGE('',*,*,#25019,.F.);
#36792=ORIENTED_EDGE('',*,*,#24550,.T.);
#36793=ORIENTED_EDGE('',*,*,#24629,.T.);
#36794=ORIENTED_EDGE('',*,*,#25021,.T.);
#36795=ORIENTED_EDGE('',*,*,#24888,.T.);
#36796=ORIENTED_EDGE('',*,*,#25022,.T.);
#36797=ORIENTED_EDGE('',*,*,#25021,.F.);
#36798=ORIENTED_EDGE('',*,*,#24628,.F.);
#36799=ORIENTED_EDGE('',*,*,#25023,.F.);
#36800=ORIENTED_EDGE('',*,*,#24889,.T.);
#36801=ORIENTED_EDGE('',*,*,#24627,.T.);
#36802=ORIENTED_EDGE('',*,*,#25024,.T.);
#36803=ORIENTED_EDGE('',*,*,#24890,.T.);
#36804=ORIENTED_EDGE('',*,*,#25023,.T.);
#36805=ORIENTED_EDGE('',*,*,#24621,.T.);
#36806=ORIENTED_EDGE('',*,*,#25025,.T.);
#36807=ORIENTED_EDGE('',*,*,#24896,.T.);
#36808=ORIENTED_EDGE('',*,*,#25026,.T.);
#36809=ORIENTED_EDGE('',*,*,#25025,.F.);
#36810=ORIENTED_EDGE('',*,*,#24620,.F.);
#36811=ORIENTED_EDGE('',*,*,#25027,.F.);
#36812=ORIENTED_EDGE('',*,*,#24897,.T.);
#36813=ORIENTED_EDGE('',*,*,#24623,.T.);
#36814=ORIENTED_EDGE('',*,*,#25028,.T.);
#36815=ORIENTED_EDGE('',*,*,#24894,.T.);
#36816=ORIENTED_EDGE('',*,*,#25029,.T.);
#36817=ORIENTED_EDGE('',*,*,#25029,.F.);
#36818=ORIENTED_EDGE('',*,*,#24893,.T.);
#36819=ORIENTED_EDGE('',*,*,#25030,.F.);
#36820=ORIENTED_EDGE('',*,*,#24624,.F.);
#36821=ORIENTED_EDGE('',*,*,#25031,.T.);
#36822=ORIENTED_EDGE('',*,*,#24761,.T.);
#36823=ORIENTED_EDGE('',*,*,#25032,.T.);
#36824=ORIENTED_EDGE('',*,*,#25011,.T.);
#36825=ORIENTED_EDGE('',*,*,#25031,.F.);
#36826=ORIENTED_EDGE('',*,*,#24504,.T.);
#36827=ORIENTED_EDGE('',*,*,#24762,.T.);
#36828=ORIENTED_EDGE('',*,*,#25032,.F.);
#36829=ORIENTED_EDGE('',*,*,#24760,.T.);
#36830=ORIENTED_EDGE('',*,*,#24557,.T.);
#36831=ORIENTED_EDGE('',*,*,#25033,.T.);
#36832=ORIENTED_EDGE('',*,*,#24764,.T.);
#36833=ORIENTED_EDGE('',*,*,#25034,.T.);
#36834=ORIENTED_EDGE('',*,*,#24982,.T.);
#36835=ORIENTED_EDGE('',*,*,#25033,.F.);
#36836=ORIENTED_EDGE('',*,*,#24568,.T.);
#36837=ORIENTED_EDGE('',*,*,#24765,.T.);
#36838=ORIENTED_EDGE('',*,*,#25034,.F.);
#36839=ORIENTED_EDGE('',*,*,#24763,.T.);
#36840=ORIENTED_EDGE('',*,*,#24521,.T.);
#36841=ORIENTED_EDGE('',*,*,#25035,.T.);
#36842=ORIENTED_EDGE('',*,*,#24758,.T.);
#36843=ORIENTED_EDGE('',*,*,#25036,.T.);
#36844=ORIENTED_EDGE('',*,*,#25009,.T.);
#36845=ORIENTED_EDGE('',*,*,#25035,.F.);
#36846=ORIENTED_EDGE('',*,*,#24543,.T.);
#36847=ORIENTED_EDGE('',*,*,#24759,.T.);
#36848=ORIENTED_EDGE('',*,*,#25036,.F.);
#36849=ORIENTED_EDGE('',*,*,#24757,.T.);
#36850=ORIENTED_EDGE('',*,*,#24585,.T.);
#36851=ORIENTED_EDGE('',*,*,#24617,.T.);
#36852=ORIENTED_EDGE('',*,*,#25037,.T.);
#36853=ORIENTED_EDGE('',*,*,#24900,.T.);
#36854=ORIENTED_EDGE('',*,*,#25038,.T.);
#36855=ORIENTED_EDGE('',*,*,#25037,.F.);
#36856=ORIENTED_EDGE('',*,*,#24616,.F.);
#36857=ORIENTED_EDGE('',*,*,#25039,.F.);
#36858=ORIENTED_EDGE('',*,*,#24901,.T.);
#36859=ORIENTED_EDGE('',*,*,#24615,.T.);
#36860=ORIENTED_EDGE('',*,*,#25040,.T.);
#36861=ORIENTED_EDGE('',*,*,#24902,.T.);
#36862=ORIENTED_EDGE('',*,*,#25039,.T.);
#36863=ORIENTED_EDGE('',*,*,#25040,.F.);
#36864=ORIENTED_EDGE('',*,*,#24614,.F.);
#36865=ORIENTED_EDGE('',*,*,#25041,.F.);
#36866=ORIENTED_EDGE('',*,*,#24903,.T.);
#36867=ORIENTED_EDGE('',*,*,#25038,.F.);
#36868=ORIENTED_EDGE('',*,*,#24899,.T.);
#36869=ORIENTED_EDGE('',*,*,#25042,.F.);
#36870=ORIENTED_EDGE('',*,*,#24618,.F.);
#36871=ORIENTED_EDGE('',*,*,#25041,.T.);
#36872=ORIENTED_EDGE('',*,*,#24613,.T.);
#36873=ORIENTED_EDGE('',*,*,#24756,.T.);
#36874=ORIENTED_EDGE('',*,*,#24904,.F.);
#36875=ORIENTED_EDGE('',*,*,#25042,.T.);
#36876=ORIENTED_EDGE('',*,*,#24898,.F.);
#36877=ORIENTED_EDGE('',*,*,#25027,.T.);
#36878=ORIENTED_EDGE('',*,*,#24619,.T.);
#36879=ORIENTED_EDGE('',*,*,#25026,.F.);
#36880=ORIENTED_EDGE('',*,*,#24895,.T.);
#36881=ORIENTED_EDGE('',*,*,#25028,.F.);
#36882=ORIENTED_EDGE('',*,*,#24622,.F.);
#36883=ORIENTED_EDGE('',*,*,#25024,.F.);
#36884=ORIENTED_EDGE('',*,*,#24626,.F.);
#36885=ORIENTED_EDGE('',*,*,#25043,.F.);
#36886=ORIENTED_EDGE('',*,*,#24891,.T.);
#36887=ORIENTED_EDGE('',*,*,#25022,.F.);
#36888=ORIENTED_EDGE('',*,*,#24887,.T.);
#36889=ORIENTED_EDGE('',*,*,#25044,.F.);
#36890=ORIENTED_EDGE('',*,*,#24630,.F.);
#36891=ORIENTED_EDGE('',*,*,#25044,.T.);
#36892=ORIENTED_EDGE('',*,*,#24886,.F.);
#36893=ORIENTED_EDGE('',*,*,#25007,.T.);
#36894=ORIENTED_EDGE('',*,*,#24631,.T.);
#36895=ORIENTED_EDGE('',*,*,#25002,.F.);
#36896=ORIENTED_EDGE('',*,*,#24634,.F.);
#36897=ORIENTED_EDGE('',*,*,#25006,.F.);
#36898=ORIENTED_EDGE('',*,*,#24883,.T.);
#36899=ORIENTED_EDGE('',*,*,#25030,.T.);
#36900=ORIENTED_EDGE('',*,*,#24892,.F.);
#36901=ORIENTED_EDGE('',*,*,#25043,.T.);
#36902=ORIENTED_EDGE('',*,*,#24625,.T.);
#36903=ORIENTED_EDGE('',*,*,#25004,.T.);
#36904=ORIENTED_EDGE('',*,*,#24880,.F.);
#36905=ORIENTED_EDGE('',*,*,#25045,.T.);
#36906=ORIENTED_EDGE('',*,*,#24637,.T.);
#36907=ORIENTED_EDGE('',*,*,#24996,.F.);
#36908=ORIENTED_EDGE('',*,*,#24875,.T.);
#36909=ORIENTED_EDGE('',*,*,#25046,.F.);
#36910=ORIENTED_EDGE('',*,*,#24642,.F.);
#36911=ORIENTED_EDGE('',*,*,#24993,.F.);
#36912=ORIENTED_EDGE('',*,*,#24638,.F.);
#36913=ORIENTED_EDGE('',*,*,#25045,.F.);
#36914=ORIENTED_EDGE('',*,*,#24879,.T.);
#36915=ORIENTED_EDGE('',*,*,#24992,.F.);
#36916=ORIENTED_EDGE('',*,*,#24644,.F.);
#36917=ORIENTED_EDGE('',*,*,#25047,.F.);
#36918=ORIENTED_EDGE('',*,*,#24873,.T.);
#36919=ORIENTED_EDGE('',*,*,#24990,.F.);
#36920=ORIENTED_EDGE('',*,*,#24869,.T.);
#36921=ORIENTED_EDGE('',*,*,#25048,.F.);
#36922=ORIENTED_EDGE('',*,*,#24648,.F.);
#36923=ORIENTED_EDGE('',*,*,#25048,.T.);
#36924=ORIENTED_EDGE('',*,*,#24868,.F.);
#36925=ORIENTED_EDGE('',*,*,#24988,.T.);
#36926=ORIENTED_EDGE('',*,*,#24649,.T.);
#36927=ORIENTED_EDGE('',*,*,#24983,.F.);
#36928=ORIENTED_EDGE('',*,*,#24652,.F.);
#36929=ORIENTED_EDGE('',*,*,#24987,.F.);
#36930=ORIENTED_EDGE('',*,*,#24865,.T.);
#36931=ORIENTED_EDGE('',*,*,#25046,.T.);
#36932=ORIENTED_EDGE('',*,*,#24874,.F.);
#36933=ORIENTED_EDGE('',*,*,#25047,.T.);
#36934=ORIENTED_EDGE('',*,*,#24643,.T.);
#36935=ORIENTED_EDGE('',*,*,#24985,.T.);
#36936=ORIENTED_EDGE('',*,*,#24862,.F.);
#36937=ORIENTED_EDGE('',*,*,#25049,.T.);
#36938=ORIENTED_EDGE('',*,*,#24655,.T.);
#36939=ORIENTED_EDGE('',*,*,#24979,.F.);
#36940=ORIENTED_EDGE('',*,*,#24857,.T.);
#36941=ORIENTED_EDGE('',*,*,#25050,.F.);
#36942=ORIENTED_EDGE('',*,*,#24660,.F.);
#36943=ORIENTED_EDGE('',*,*,#24976,.F.);
#36944=ORIENTED_EDGE('',*,*,#24656,.F.);
#36945=ORIENTED_EDGE('',*,*,#25049,.F.);
#36946=ORIENTED_EDGE('',*,*,#24861,.T.);
#36947=ORIENTED_EDGE('',*,*,#24975,.F.);
#36948=ORIENTED_EDGE('',*,*,#24662,.F.);
#36949=ORIENTED_EDGE('',*,*,#25051,.F.);
#36950=ORIENTED_EDGE('',*,*,#24855,.T.);
#36951=ORIENTED_EDGE('',*,*,#24973,.F.);
#36952=ORIENTED_EDGE('',*,*,#24851,.T.);
#36953=ORIENTED_EDGE('',*,*,#25052,.F.);
#36954=ORIENTED_EDGE('',*,*,#24666,.F.);
#36955=ORIENTED_EDGE('',*,*,#25052,.T.);
#36956=ORIENTED_EDGE('',*,*,#24850,.F.);
#36957=ORIENTED_EDGE('',*,*,#24971,.T.);
#36958=ORIENTED_EDGE('',*,*,#24667,.T.);
#36959=ORIENTED_EDGE('',*,*,#24966,.F.);
#36960=ORIENTED_EDGE('',*,*,#24670,.F.);
#36961=ORIENTED_EDGE('',*,*,#24970,.F.);
#36962=ORIENTED_EDGE('',*,*,#24847,.T.);
#36963=ORIENTED_EDGE('',*,*,#25050,.T.);
#36964=ORIENTED_EDGE('',*,*,#24856,.F.);
#36965=ORIENTED_EDGE('',*,*,#25051,.T.);
#36966=ORIENTED_EDGE('',*,*,#24661,.T.);
#36967=ORIENTED_EDGE('',*,*,#24968,.T.);
#36968=ORIENTED_EDGE('',*,*,#24844,.F.);
#36969=ORIENTED_EDGE('',*,*,#25053,.T.);
#36970=ORIENTED_EDGE('',*,*,#24673,.T.);
#36971=ORIENTED_EDGE('',*,*,#24965,.F.);
#36972=ORIENTED_EDGE('',*,*,#24839,.T.);
#36973=ORIENTED_EDGE('',*,*,#25054,.F.);
#36974=ORIENTED_EDGE('',*,*,#24678,.F.);
#36975=ORIENTED_EDGE('',*,*,#24962,.F.);
#36976=ORIENTED_EDGE('',*,*,#24674,.F.);
#36977=ORIENTED_EDGE('',*,*,#25053,.F.);
#36978=ORIENTED_EDGE('',*,*,#24843,.T.);
#36979=ORIENTED_EDGE('',*,*,#24961,.F.);
#36980=ORIENTED_EDGE('',*,*,#24680,.F.);
#36981=ORIENTED_EDGE('',*,*,#25055,.F.);
#36982=ORIENTED_EDGE('',*,*,#24837,.T.);
#36983=ORIENTED_EDGE('',*,*,#24959,.F.);
#36984=ORIENTED_EDGE('',*,*,#24833,.T.);
#36985=ORIENTED_EDGE('',*,*,#25056,.F.);
#36986=ORIENTED_EDGE('',*,*,#24684,.F.);
#36987=ORIENTED_EDGE('',*,*,#25056,.T.);
#36988=ORIENTED_EDGE('',*,*,#24832,.F.);
#36989=ORIENTED_EDGE('',*,*,#24957,.T.);
#36990=ORIENTED_EDGE('',*,*,#24685,.T.);
#36991=ORIENTED_EDGE('',*,*,#24952,.F.);
#36992=ORIENTED_EDGE('',*,*,#24688,.F.);
#36993=ORIENTED_EDGE('',*,*,#24956,.F.);
#36994=ORIENTED_EDGE('',*,*,#24829,.T.);
#36995=ORIENTED_EDGE('',*,*,#25054,.T.);
#36996=ORIENTED_EDGE('',*,*,#24838,.F.);
#36997=ORIENTED_EDGE('',*,*,#25055,.T.);
#36998=ORIENTED_EDGE('',*,*,#24679,.T.);
#36999=ORIENTED_EDGE('',*,*,#24954,.T.);
#37000=ORIENTED_EDGE('',*,*,#24826,.F.);
#37001=ORIENTED_EDGE('',*,*,#25057,.T.);
#37002=ORIENTED_EDGE('',*,*,#24691,.T.);
#37003=ORIENTED_EDGE('',*,*,#24951,.F.);
#37004=ORIENTED_EDGE('',*,*,#24821,.T.);
#37005=ORIENTED_EDGE('',*,*,#25058,.F.);
#37006=ORIENTED_EDGE('',*,*,#24696,.F.);
#37007=ORIENTED_EDGE('',*,*,#24948,.F.);
#37008=ORIENTED_EDGE('',*,*,#24692,.F.);
#37009=ORIENTED_EDGE('',*,*,#25057,.F.);
#37010=ORIENTED_EDGE('',*,*,#24825,.T.);
#37011=ORIENTED_EDGE('',*,*,#24947,.F.);
#37012=ORIENTED_EDGE('',*,*,#24698,.F.);
#37013=ORIENTED_EDGE('',*,*,#25059,.F.);
#37014=ORIENTED_EDGE('',*,*,#24819,.T.);
#37015=ORIENTED_EDGE('',*,*,#24945,.F.);
#37016=ORIENTED_EDGE('',*,*,#24815,.T.);
#37017=ORIENTED_EDGE('',*,*,#25060,.F.);
#37018=ORIENTED_EDGE('',*,*,#24702,.F.);
#37019=ORIENTED_EDGE('',*,*,#25060,.T.);
#37020=ORIENTED_EDGE('',*,*,#24814,.F.);
#37021=ORIENTED_EDGE('',*,*,#24943,.T.);
#37022=ORIENTED_EDGE('',*,*,#24703,.T.);
#37023=ORIENTED_EDGE('',*,*,#24938,.F.);
#37024=ORIENTED_EDGE('',*,*,#24706,.F.);
#37025=ORIENTED_EDGE('',*,*,#24942,.F.);
#37026=ORIENTED_EDGE('',*,*,#24811,.T.);
#37027=ORIENTED_EDGE('',*,*,#25058,.T.);
#37028=ORIENTED_EDGE('',*,*,#24820,.F.);
#37029=ORIENTED_EDGE('',*,*,#25059,.T.);
#37030=ORIENTED_EDGE('',*,*,#24697,.T.);
#37031=ORIENTED_EDGE('',*,*,#24940,.T.);
#37032=ORIENTED_EDGE('',*,*,#24808,.F.);
#37033=ORIENTED_EDGE('',*,*,#25061,.T.);
#37034=ORIENTED_EDGE('',*,*,#24709,.T.);
#37035=ORIENTED_EDGE('',*,*,#24937,.F.);
#37036=ORIENTED_EDGE('',*,*,#24803,.T.);
#37037=ORIENTED_EDGE('',*,*,#25062,.F.);
#37038=ORIENTED_EDGE('',*,*,#24714,.F.);
#37039=ORIENTED_EDGE('',*,*,#24934,.F.);
#37040=ORIENTED_EDGE('',*,*,#24710,.F.);
#37041=ORIENTED_EDGE('',*,*,#25061,.F.);
#37042=ORIENTED_EDGE('',*,*,#24807,.T.);
#37043=ORIENTED_EDGE('',*,*,#24933,.F.);
#37044=ORIENTED_EDGE('',*,*,#24716,.F.);
#37045=ORIENTED_EDGE('',*,*,#25063,.F.);
#37046=ORIENTED_EDGE('',*,*,#24801,.T.);
#37047=ORIENTED_EDGE('',*,*,#24931,.F.);
#37048=ORIENTED_EDGE('',*,*,#24797,.T.);
#37049=ORIENTED_EDGE('',*,*,#25064,.F.);
#37050=ORIENTED_EDGE('',*,*,#24720,.F.);
#37051=ORIENTED_EDGE('',*,*,#25064,.T.);
#37052=ORIENTED_EDGE('',*,*,#24796,.F.);
#37053=ORIENTED_EDGE('',*,*,#24929,.T.);
#37054=ORIENTED_EDGE('',*,*,#24721,.T.);
#37055=ORIENTED_EDGE('',*,*,#24924,.F.);
#37056=ORIENTED_EDGE('',*,*,#24724,.F.);
#37057=ORIENTED_EDGE('',*,*,#24928,.F.);
#37058=ORIENTED_EDGE('',*,*,#24793,.T.);
#37059=ORIENTED_EDGE('',*,*,#25062,.T.);
#37060=ORIENTED_EDGE('',*,*,#24802,.F.);
#37061=ORIENTED_EDGE('',*,*,#25063,.T.);
#37062=ORIENTED_EDGE('',*,*,#24715,.T.);
#37063=ORIENTED_EDGE('',*,*,#24926,.T.);
#37064=ORIENTED_EDGE('',*,*,#24790,.F.);
#37065=ORIENTED_EDGE('',*,*,#25065,.T.);
#37066=ORIENTED_EDGE('',*,*,#24727,.T.);
#37067=ORIENTED_EDGE('',*,*,#24923,.F.);
#37068=ORIENTED_EDGE('',*,*,#24785,.T.);
#37069=ORIENTED_EDGE('',*,*,#25066,.F.);
#37070=ORIENTED_EDGE('',*,*,#24732,.F.);
#37071=ORIENTED_EDGE('',*,*,#24920,.F.);
#37072=ORIENTED_EDGE('',*,*,#24728,.F.);
#37073=ORIENTED_EDGE('',*,*,#25065,.F.);
#37074=ORIENTED_EDGE('',*,*,#24789,.T.);
#37075=ORIENTED_EDGE('',*,*,#24919,.F.);
#37076=ORIENTED_EDGE('',*,*,#24734,.F.);
#37077=ORIENTED_EDGE('',*,*,#25067,.F.);
#37078=ORIENTED_EDGE('',*,*,#24783,.T.);
#37079=ORIENTED_EDGE('',*,*,#24917,.F.);
#37080=ORIENTED_EDGE('',*,*,#24779,.T.);
#37081=ORIENTED_EDGE('',*,*,#25068,.F.);
#37082=ORIENTED_EDGE('',*,*,#24738,.F.);
#37083=ORIENTED_EDGE('',*,*,#25068,.T.);
#37084=ORIENTED_EDGE('',*,*,#24778,.F.);
#37085=ORIENTED_EDGE('',*,*,#24915,.T.);
#37086=ORIENTED_EDGE('',*,*,#24739,.T.);
#37087=ORIENTED_EDGE('',*,*,#24910,.F.);
#37088=ORIENTED_EDGE('',*,*,#24742,.F.);
#37089=ORIENTED_EDGE('',*,*,#24914,.F.);
#37090=ORIENTED_EDGE('',*,*,#24775,.T.);
#37091=ORIENTED_EDGE('',*,*,#25066,.T.);
#37092=ORIENTED_EDGE('',*,*,#24784,.F.);
#37093=ORIENTED_EDGE('',*,*,#25067,.T.);
#37094=ORIENTED_EDGE('',*,*,#24733,.T.);
#37095=ORIENTED_EDGE('',*,*,#24912,.T.);
#37096=ORIENTED_EDGE('',*,*,#24772,.F.);
#37097=ORIENTED_EDGE('',*,*,#25069,.T.);
#37098=ORIENTED_EDGE('',*,*,#24745,.T.);
#37099=ORIENTED_EDGE('',*,*,#24909,.F.);
#37100=ORIENTED_EDGE('',*,*,#24767,.T.);
#37101=ORIENTED_EDGE('',*,*,#25070,.F.);
#37102=ORIENTED_EDGE('',*,*,#24750,.F.);
#37103=ORIENTED_EDGE('',*,*,#24906,.F.);
#37104=ORIENTED_EDGE('',*,*,#24746,.F.);
#37105=ORIENTED_EDGE('',*,*,#25069,.F.);
#37106=ORIENTED_EDGE('',*,*,#24771,.T.);
#37107=ORIENTED_EDGE('',*,*,#24597,.F.);
#37108=ORIENTED_EDGE('',*,*,#24905,.T.);
#37109=ORIENTED_EDGE('',*,*,#24752,.F.);
#37110=ORIENTED_EDGE('',*,*,#24610,.F.);
#37111=ORIENTED_EDGE('',*,*,#24532,.F.);
#37112=ORIENTED_EDGE('',*,*,#24553,.T.);
#37113=ORIENTED_EDGE('',*,*,#25013,.F.);
#37114=ORIENTED_EDGE('',*,*,#24511,.T.);
#37115=ORIENTED_EDGE('',*,*,#25070,.T.);
#37116=ORIENTED_EDGE('',*,*,#24766,.F.);
#37117=ORIENTED_EDGE('',*,*,#24599,.T.);
#37118=ORIENTED_EDGE('',*,*,#24751,.T.);
#37864=CYLINDRICAL_SURFACE('',#44815,8.99999999999999);
#37865=CYLINDRICAL_SURFACE('',#44828,15.);
#37866=CYLINDRICAL_SURFACE('',#44834,8.99999999999999);
#37867=CYLINDRICAL_SURFACE('',#44849,8.99999999999999);
#37868=CYLINDRICAL_SURFACE('',#44859,0.4);
#37869=CYLINDRICAL_SURFACE('',#44938,0.4);
#37870=CYLINDRICAL_SURFACE('',#45015,0.4);
#37871=CYLINDRICAL_SURFACE('',#45017,0.4);
#37872=CYLINDRICAL_SURFACE('',#45018,0.4);
#37873=CYLINDRICAL_SURFACE('',#45020,0.4);
#37874=CYLINDRICAL_SURFACE('',#45022,0.4);
#37875=CYLINDRICAL_SURFACE('',#45024,0.4);
#37876=CYLINDRICAL_SURFACE('',#45025,0.4);
#37877=CYLINDRICAL_SURFACE('',#45027,0.4);
#37878=CYLINDRICAL_SURFACE('',#45028,0.4);
#37879=CYLINDRICAL_SURFACE('',#45030,0.4);
#37880=CYLINDRICAL_SURFACE('',#45032,0.4);
#37881=CYLINDRICAL_SURFACE('',#45034,0.4);
#37882=CYLINDRICAL_SURFACE('',#45035,0.4);
#37883=CYLINDRICAL_SURFACE('',#45037,0.4);
#37884=CYLINDRICAL_SURFACE('',#45038,0.4);
#37885=CYLINDRICAL_SURFACE('',#45040,0.4);
#37886=CYLINDRICAL_SURFACE('',#45042,0.4);
#37887=CYLINDRICAL_SURFACE('',#45044,0.4);
#37888=CYLINDRICAL_SURFACE('',#45045,0.4);
#37889=CYLINDRICAL_SURFACE('',#45047,0.4);
#37890=CYLINDRICAL_SURFACE('',#45048,0.4);
#37891=CYLINDRICAL_SURFACE('',#45050,0.4);
#37892=CYLINDRICAL_SURFACE('',#45052,0.4);
#37893=CYLINDRICAL_SURFACE('',#45054,0.4);
#37894=CYLINDRICAL_SURFACE('',#45055,0.4);
#37895=CYLINDRICAL_SURFACE('',#45057,0.4);
#37896=CYLINDRICAL_SURFACE('',#45058,0.4);
#37897=CYLINDRICAL_SURFACE('',#45060,0.4);
#37898=CYLINDRICAL_SURFACE('',#45062,0.4);
#37899=CYLINDRICAL_SURFACE('',#45064,0.4);
#37900=CYLINDRICAL_SURFACE('',#45065,0.4);
#37901=CYLINDRICAL_SURFACE('',#45067,0.4);
#37902=CYLINDRICAL_SURFACE('',#45073,0.4);
#37903=CYLINDRICAL_SURFACE('',#45075,0.4);
#37904=CYLINDRICAL_SURFACE('',#45077,0.4);
#37905=CYLINDRICAL_SURFACE('',#45079,0.4);
#37906=CYLINDRICAL_SURFACE('',#45080,0.4);
#37907=CYLINDRICAL_SURFACE('',#45082,0.4);
#37908=CYLINDRICAL_SURFACE('',#45086,15.);
#37909=CYLINDRICAL_SURFACE('',#45091,15.);
#37910=CYLINDRICAL_SURFACE('',#45092,0.4);
#37911=CYLINDRICAL_SURFACE('',#45094,0.4);
#37912=CYLINDRICAL_SURFACE('',#45118,0.4);
#37913=CYLINDRICAL_SURFACE('',#45120,0.4);
#37914=CYLINDRICAL_SURFACE('',#45121,0.4);
#37915=CYLINDRICAL_SURFACE('',#45123,0.4);
#37916=CYLINDRICAL_SURFACE('',#45134,0.4);
#37917=CYLINDRICAL_SURFACE('',#45136,0.4);
#37918=CYLINDRICAL_SURFACE('',#45139,12.);
#37919=CYLINDRICAL_SURFACE('',#45140,12.);
#37920=CYLINDRICAL_SURFACE('',#45144,12.);
#37921=CYLINDRICAL_SURFACE('',#45146,12.);
#37922=CYLINDRICAL_SURFACE('',#45147,12.);
#37923=CYLINDRICAL_SURFACE('',#45152,12.);
#37924=CYLINDRICAL_SURFACE('',#45154,12.);
#37925=CYLINDRICAL_SURFACE('',#45155,12.);
#37926=CYLINDRICAL_SURFACE('',#45160,12.);
#37927=CYLINDRICAL_SURFACE('',#45162,12.);
#37928=CYLINDRICAL_SURFACE('',#45163,12.);
#37929=CYLINDRICAL_SURFACE('',#45168,12.);
#37930=CYLINDRICAL_SURFACE('',#45170,12.);
#37931=CYLINDRICAL_SURFACE('',#45171,12.);
#37932=CYLINDRICAL_SURFACE('',#45176,12.);
#37933=CYLINDRICAL_SURFACE('',#45178,12.);
#37934=CYLINDRICAL_SURFACE('',#45179,12.);
#37935=CYLINDRICAL_SURFACE('',#45184,12.);
#37936=CYLINDRICAL_SURFACE('',#45186,12.);
#37937=CYLINDRICAL_SURFACE('',#45187,12.);
#37938=CYLINDRICAL_SURFACE('',#45192,12.);
#37939=CYLINDRICAL_SURFACE('',#45194,12.);
#37940=CYLINDRICAL_SURFACE('',#45195,12.);
#37941=CYLINDRICAL_SURFACE('',#45200,12.);
#40120=ADVANCED_FACE('',(#4317),#1010,.T.);
#40121=ADVANCED_FACE('',(#4318),#37864,.T.);
#40122=ADVANCED_FACE('',(#4319),#1736,.T.);
#40123=ADVANCED_FACE('',(#4320),#1011,.T.);
#40124=ADVANCED_FACE('',(#4321),#1737,.F.);
#40125=ADVANCED_FACE('',(#4322),#1012,.T.);
#40126=ADVANCED_FACE('',(#4323),#1738,.F.);
#40127=ADVANCED_FACE('',(#4324),#1013,.T.);
#40128=ADVANCED_FACE('',(#4325),#37865,.T.);
#40129=ADVANCED_FACE('',(#4326),#1014,.T.);
#40130=ADVANCED_FACE('',(#4327),#37866,.T.);
#40131=ADVANCED_FACE('',(#4328),#1739,.T.);
#40132=ADVANCED_FACE('',(#4329),#1015,.T.);
#40133=ADVANCED_FACE('',(#4330),#1740,.F.);
#40134=ADVANCED_FACE('',(#4331),#1016,.T.);
#40135=ADVANCED_FACE('',(#4332),#1741,.F.);
#40136=ADVANCED_FACE('',(#4333),#1017,.T.);
#40137=ADVANCED_FACE('',(#4334),#37867,.T.);
#40138=ADVANCED_FACE('',(#4335),#1742,.T.);
#40139=ADVANCED_FACE('',(#4336),#1018,.T.);
#40140=ADVANCED_FACE('',(#4337),#1743,.F.);
#40141=ADVANCED_FACE('',(#4338),#1019,.T.);
#40142=ADVANCED_FACE('',(#4339),#1744,.F.);
#40143=ADVANCED_FACE('',(#4340),#37868,.T.);
#40144=ADVANCED_FACE('',(#4341),#1745,.T.);
#40145=ADVANCED_FACE('',(#4342,#1108),#1746,.T.);
#40146=ADVANCED_FACE('',(#4343),#37869,.T.);
#40147=ADVANCED_FACE('',(#4344),#1747,.T.);
#40148=ADVANCED_FACE('',(#4345,#1109),#1748,.T.);
#40149=ADVANCED_FACE('',(#4346),#37870,.T.);
#40150=ADVANCED_FACE('',(#4347),#1749,.T.);
#40151=ADVANCED_FACE('',(#4348),#37871,.T.);
#40152=ADVANCED_FACE('',(#4349),#37872,.T.);
#40153=ADVANCED_FACE('',(#4350),#1750,.T.);
#40154=ADVANCED_FACE('',(#4351),#37873,.T.);
#40155=ADVANCED_FACE('',(#4352),#1751,.T.);
#40156=ADVANCED_FACE('',(#4353),#37874,.T.);
#40157=ADVANCED_FACE('',(#4354),#1752,.T.);
#40158=ADVANCED_FACE('',(#4355),#37875,.T.);
#40159=ADVANCED_FACE('',(#4356),#37876,.T.);
#40160=ADVANCED_FACE('',(#4357),#1753,.T.);
#40161=ADVANCED_FACE('',(#4358),#37877,.T.);
#40162=ADVANCED_FACE('',(#4359),#37878,.T.);
#40163=ADVANCED_FACE('',(#4360),#1754,.T.);
#40164=ADVANCED_FACE('',(#4361),#37879,.T.);
#40165=ADVANCED_FACE('',(#4362),#1755,.T.);
#40166=ADVANCED_FACE('',(#4363),#37880,.T.);
#40167=ADVANCED_FACE('',(#4364),#1756,.T.);
#40168=ADVANCED_FACE('',(#4365),#37881,.T.);
#40169=ADVANCED_FACE('',(#4366),#37882,.T.);
#40170=ADVANCED_FACE('',(#4367),#1757,.T.);
#40171=ADVANCED_FACE('',(#4368),#37883,.T.);
#40172=ADVANCED_FACE('',(#4369),#37884,.T.);
#40173=ADVANCED_FACE('',(#4370),#1758,.T.);
#40174=ADVANCED_FACE('',(#4371),#37885,.T.);
#40175=ADVANCED_FACE('',(#4372),#1759,.T.);
#40176=ADVANCED_FACE('',(#4373),#37886,.T.);
#40177=ADVANCED_FACE('',(#4374),#1760,.T.);
#40178=ADVANCED_FACE('',(#4375),#37887,.T.);
#40179=ADVANCED_FACE('',(#4376),#37888,.T.);
#40180=ADVANCED_FACE('',(#4377),#1761,.T.);
#40181=ADVANCED_FACE('',(#4378),#37889,.T.);
#40182=ADVANCED_FACE('',(#4379),#37890,.T.);
#40183=ADVANCED_FACE('',(#4380),#1762,.T.);
#40184=ADVANCED_FACE('',(#4381),#37891,.T.);
#40185=ADVANCED_FACE('',(#4382),#1763,.T.);
#40186=ADVANCED_FACE('',(#4383),#37892,.T.);
#40187=ADVANCED_FACE('',(#4384),#1764,.T.);
#40188=ADVANCED_FACE('',(#4385),#37893,.T.);
#40189=ADVANCED_FACE('',(#4386),#37894,.T.);
#40190=ADVANCED_FACE('',(#4387),#1765,.T.);
#40191=ADVANCED_FACE('',(#4388),#37895,.T.);
#40192=ADVANCED_FACE('',(#4389),#37896,.T.);
#40193=ADVANCED_FACE('',(#4390),#1766,.T.);
#40194=ADVANCED_FACE('',(#4391),#37897,.T.);
#40195=ADVANCED_FACE('',(#4392),#1767,.T.);
#40196=ADVANCED_FACE('',(#4393),#37898,.T.);
#40197=ADVANCED_FACE('',(#4394),#1768,.T.);
#40198=ADVANCED_FACE('',(#4395),#37899,.T.);
#40199=ADVANCED_FACE('',(#4396),#37900,.T.);
#40200=ADVANCED_FACE('',(#4397),#1769,.T.);
#40201=ADVANCED_FACE('',(#4398),#37901,.T.);
#40202=ADVANCED_FACE('',(#4399),#1020,.T.);
#40203=ADVANCED_FACE('',(#4400),#775,.T.);
#40204=ADVANCED_FACE('',(#4401),#37902,.T.);
#40205=ADVANCED_FACE('',(#4402),#1770,.T.);
#40206=ADVANCED_FACE('',(#4403),#37903,.T.);
#40207=ADVANCED_FACE('',(#4404),#1771,.T.);
#40208=ADVANCED_FACE('',(#4405),#37904,.T.);
#40209=ADVANCED_FACE('',(#4406),#1772,.T.);
#40210=ADVANCED_FACE('',(#4407),#37905,.T.);
#40211=ADVANCED_FACE('',(#4408),#37906,.T.);
#40212=ADVANCED_FACE('',(#4409),#1773,.T.);
#40213=ADVANCED_FACE('',(#4410),#37907,.T.);
#40214=ADVANCED_FACE('',(#4411),#1021,.T.);
#40215=ADVANCED_FACE('',(#4412),#37908,.T.);
#40216=ADVANCED_FACE('',(#4413),#1022,.T.);
#40217=ADVANCED_FACE('',(#4414),#37909,.T.);
#40218=ADVANCED_FACE('',(#4415),#37910,.T.);
#40219=ADVANCED_FACE('',(#4416),#1774,.T.);
#40220=ADVANCED_FACE('',(#4417),#37911,.T.);
#40221=ADVANCED_FACE('',(#4418),#1775,.T.);
#40222=ADVANCED_FACE('',(#4419),#1023,.T.);
#40223=ADVANCED_FACE('',(#4420),#776,.T.);
#40224=ADVANCED_FACE('',(#4421),#1024,.T.);
#40225=ADVANCED_FACE('',(#4422),#777,.T.);
#40226=ADVANCED_FACE('',(#4423),#1025,.T.);
#40227=ADVANCED_FACE('',(#4424),#2133,.F.);
#40228=ADVANCED_FACE('',(#4425),#2134,.F.);
#40229=ADVANCED_FACE('',(#4426),#1026,.T.);
#40230=ADVANCED_FACE('',(#4427),#2135,.F.);
#40231=ADVANCED_FACE('',(#4428),#2136,.F.);
#40232=ADVANCED_FACE('',(#4429),#1027,.T.);
#40233=ADVANCED_FACE('',(#4430),#2137,.F.);
#40234=ADVANCED_FACE('',(#4431),#2138,.F.);
#40235=ADVANCED_FACE('',(#4432),#778,.T.);
#40236=ADVANCED_FACE('',(#4433),#779,.T.);
#40237=ADVANCED_FACE('',(#4434),#37912,.T.);
#40238=ADVANCED_FACE('',(#4435),#1776,.T.);
#40239=ADVANCED_FACE('',(#4436),#37913,.T.);
#40240=ADVANCED_FACE('',(#4437),#37914,.T.);
#40241=ADVANCED_FACE('',(#4438),#1777,.T.);
#40242=ADVANCED_FACE('',(#4439),#37915,.T.);
#40243=ADVANCED_FACE('',(#4440),#1778,.T.);
#40244=ADVANCED_FACE('',(#4441),#1028,.T.);
#40245=ADVANCED_FACE('',(#4442),#2139,.F.);
#40246=ADVANCED_FACE('',(#4443),#2140,.F.);
#40247=ADVANCED_FACE('',(#4444),#1029,.T.);
#40248=ADVANCED_FACE('',(#4445),#2141,.F.);
#40249=ADVANCED_FACE('',(#4446),#2142,.F.);
#40250=ADVANCED_FACE('',(#4447),#1030,.T.);
#40251=ADVANCED_FACE('',(#4448),#2143,.F.);
#40252=ADVANCED_FACE('',(#4449),#2144,.F.);
#40253=ADVANCED_FACE('',(#4450),#37916,.T.);
#40254=ADVANCED_FACE('',(#4451),#1779,.T.);
#40255=ADVANCED_FACE('',(#4452),#37917,.T.);
#40256=ADVANCED_FACE('',(#4453),#1780,.T.);
#40257=ADVANCED_FACE('',(#4454),#1781,.T.);
#40258=ADVANCED_FACE('',(#4455),#37918,.F.);
#40259=ADVANCED_FACE('',(#4456),#37919,.F.);
#40260=ADVANCED_FACE('',(#4457),#1782,.T.);
#40261=ADVANCED_FACE('',(#4458),#1783,.T.);
#40262=ADVANCED_FACE('',(#4459),#1784,.T.);
#40263=ADVANCED_FACE('',(#4460),#37920,.F.);
#40264=ADVANCED_FACE('',(#4461),#1785,.T.);
#40265=ADVANCED_FACE('',(#4462),#37921,.F.);
#40266=ADVANCED_FACE('',(#4463),#37922,.F.);
#40267=ADVANCED_FACE('',(#4464),#1786,.T.);
#40268=ADVANCED_FACE('',(#4465),#1787,.T.);
#40269=ADVANCED_FACE('',(#4466),#1788,.T.);
#40270=ADVANCED_FACE('',(#4467),#1789,.T.);
#40271=ADVANCED_FACE('',(#4468),#37923,.F.);
#40272=ADVANCED_FACE('',(#4469),#1790,.T.);
#40273=ADVANCED_FACE('',(#4470),#37924,.F.);
#40274=ADVANCED_FACE('',(#4471),#37925,.F.);
#40275=ADVANCED_FACE('',(#4472),#1791,.T.);
#40276=ADVANCED_FACE('',(#4473),#1792,.T.);
#40277=ADVANCED_FACE('',(#4474),#1793,.T.);
#40278=ADVANCED_FACE('',(#4475),#1794,.T.);
#40279=ADVANCED_FACE('',(#4476),#37926,.F.);
#40280=ADVANCED_FACE('',(#4477),#1795,.T.);
#40281=ADVANCED_FACE('',(#4478),#37927,.F.);
#40282=ADVANCED_FACE('',(#4479),#37928,.F.);
#40283=ADVANCED_FACE('',(#4480),#1796,.T.);
#40284=ADVANCED_FACE('',(#4481),#1797,.T.);
#40285=ADVANCED_FACE('',(#4482),#1798,.T.);
#40286=ADVANCED_FACE('',(#4483),#1799,.T.);
#40287=ADVANCED_FACE('',(#4484),#37929,.F.);
#40288=ADVANCED_FACE('',(#4485),#1800,.T.);
#40289=ADVANCED_FACE('',(#4486),#37930,.F.);
#40290=ADVANCED_FACE('',(#4487),#37931,.F.);
#40291=ADVANCED_FACE('',(#4488),#1801,.T.);
#40292=ADVANCED_FACE('',(#4489),#1802,.T.);
#40293=ADVANCED_FACE('',(#4490),#1803,.T.);
#40294=ADVANCED_FACE('',(#4491),#1804,.T.);
#40295=ADVANCED_FACE('',(#4492),#37932,.F.);
#40296=ADVANCED_FACE('',(#4493),#1805,.T.);
#40297=ADVANCED_FACE('',(#4494),#37933,.F.);
#40298=ADVANCED_FACE('',(#4495),#37934,.F.);
#40299=ADVANCED_FACE('',(#4496),#1806,.T.);
#40300=ADVANCED_FACE('',(#4497),#1807,.T.);
#40301=ADVANCED_FACE('',(#4498),#1808,.T.);
#40302=ADVANCED_FACE('',(#4499),#1809,.T.);
#40303=ADVANCED_FACE('',(#4500),#37935,.F.);
#40304=ADVANCED_FACE('',(#4501),#1810,.T.);
#40305=ADVANCED_FACE('',(#4502),#37936,.F.);
#40306=ADVANCED_FACE('',(#4503),#37937,.F.);
#40307=ADVANCED_FACE('',(#4504),#1811,.T.);
#40308=ADVANCED_FACE('',(#4505),#1812,.T.);
#40309=ADVANCED_FACE('',(#4506),#1813,.T.);
#40310=ADVANCED_FACE('',(#4507),#1814,.T.);
#40311=ADVANCED_FACE('',(#4508),#37938,.F.);
#40312=ADVANCED_FACE('',(#4509),#1815,.T.);
#40313=ADVANCED_FACE('',(#4510),#37939,.F.);
#40314=ADVANCED_FACE('',(#4511),#37940,.F.);
#40315=ADVANCED_FACE('',(#4512),#1816,.T.);
#40316=ADVANCED_FACE('',(#4513),#1817,.T.);
#40317=ADVANCED_FACE('',(#4514),#1818,.T.);
#40318=ADVANCED_FACE('',(#4515),#780,.T.);
#40319=ADVANCED_FACE('',(#4516),#37941,.F.);
#40358=CLOSED_SHELL('',(#40120,#40121,#40122,#40123,#40124,#40125,#40126,
#40127,#40128,#40129,#40130,#40131,#40132,#40133,#40134,#40135,#40136,#40137,
#40138,#40139,#40140,#40141,#40142,#40143,#40144,#40145,#40146,#40147,#40148,
#40149,#40150,#40151,#40152,#40153,#40154,#40155,#40156,#40157,#40158,#40159,
#40160,#40161,#40162,#40163,#40164,#40165,#40166,#40167,#40168,#40169,#40170,
#40171,#40172,#40173,#40174,#40175,#40176,#40177,#40178,#40179,#40180,#40181,
#40182,#40183,#40184,#40185,#40186,#40187,#40188,#40189,#40190,#40191,#40192,
#40193,#40194,#40195,#40196,#40197,#40198,#40199,#40200,#40201,#40202,#40203,
#40204,#40205,#40206,#40207,#40208,#40209,#40210,#40211,#40212,#40213,#40214,
#40215,#40216,#40217,#40218,#40219,#40220,#40221,#40222,#40223,#40224,#40225,
#40226,#40227,#40228,#40229,#40230,#40231,#40232,#40233,#40234,#40235,#40236,
#40237,#40238,#40239,#40240,#40241,#40242,#40243,#40244,#40245,#40246,#40247,
#40248,#40249,#40250,#40251,#40252,#40253,#40254,#40255,#40256,#40257,#40258,
#40259,#40260,#40261,#40262,#40263,#40264,#40265,#40266,#40267,#40268,#40269,
#40270,#40271,#40272,#40273,#40274,#40275,#40276,#40277,#40278,#40279,#40280,
#40281,#40282,#40283,#40284,#40285,#40286,#40287,#40288,#40289,#40290,#40291,
#40292,#40293,#40294,#40295,#40296,#40297,#40298,#40299,#40300,#40301,#40302,
#40303,#40304,#40305,#40306,#40307,#40308,#40309,#40310,#40311,#40312,#40313,
#40314,#40315,#40316,#40317,#40318,#40319));
#44809=AXIS2_PLACEMENT_3D('',#88374,#55999,#56000);
#44810=AXIS2_PLACEMENT_3D('',#88375,#56001,#56002);
#44811=AXIS2_PLACEMENT_3D('',#88377,#56003,#56004);
#44812=AXIS2_PLACEMENT_3D('',#88379,#56005,#56006);
#44813=AXIS2_PLACEMENT_3D('',#88381,#56007,#56008);
#44814=AXIS2_PLACEMENT_3D('',#88382,#56009,#56010);
#44815=AXIS2_PLACEMENT_3D('',#88383,#56011,#56012);
#44816=AXIS2_PLACEMENT_3D('',#88416,#56014,#56015);
#44817=AXIS2_PLACEMENT_3D('',#88474,#56016,#56017);
#44818=AXIS2_PLACEMENT_3D('',#88501,#56018,#56019);
#44819=AXIS2_PLACEMENT_3D('',#88502,#56020,#56021);
#44820=AXIS2_PLACEMENT_3D('',#88515,#56022,#56023);
#44821=AXIS2_PLACEMENT_3D('',#88524,#56024,#56025);
#44822=AXIS2_PLACEMENT_3D('',#88526,#56027,#56028);
#44823=AXIS2_PLACEMENT_3D('',#88539,#56029,#56030);
#44824=AXIS2_PLACEMENT_3D('',#88548,#56031,#56032);
#44825=AXIS2_PLACEMENT_3D('',#88550,#56034,#56035);
#44826=AXIS2_PLACEMENT_3D('',#88552,#56036,#56037);
#44827=AXIS2_PLACEMENT_3D('',#88560,#56038,#56039);
#44828=AXIS2_PLACEMENT_3D('',#88561,#56040,#56041);
#44829=AXIS2_PLACEMENT_3D('',#88563,#56042,#56043);
#44830=AXIS2_PLACEMENT_3D('',#88599,#56045,#56046);
#44831=AXIS2_PLACEMENT_3D('',#88601,#56047,#56048);
#44832=AXIS2_PLACEMENT_3D('',#88603,#56049,#56050);
#44833=AXIS2_PLACEMENT_3D('',#88604,#56051,#56052);
#44834=AXIS2_PLACEMENT_3D('',#88605,#56053,#56054);
#44835=AXIS2_PLACEMENT_3D('',#88638,#56056,#56057);
#44836=AXIS2_PLACEMENT_3D('',#88680,#56058,#56059);
#44837=AXIS2_PLACEMENT_3D('',#88700,#56060,#56061);
#44838=AXIS2_PLACEMENT_3D('',#88701,#56062,#56063);
#44839=AXIS2_PLACEMENT_3D('',#88702,#56064,#56065);
#44840=AXIS2_PLACEMENT_3D('',#88703,#56066,#56067);
#44841=AXIS2_PLACEMENT_3D('',#88704,#56068,#56069);
#44842=AXIS2_PLACEMENT_3D('',#88717,#56070,#56071);
#44843=AXIS2_PLACEMENT_3D('',#88726,#56072,#56073);
#44844=AXIS2_PLACEMENT_3D('',#88728,#56075,#56076);
#44845=AXIS2_PLACEMENT_3D('',#88730,#56077,#56078);
#44846=AXIS2_PLACEMENT_3D('',#88732,#56079,#56080);
#44847=AXIS2_PLACEMENT_3D('',#88734,#56081,#56082);
#44848=AXIS2_PLACEMENT_3D('',#88735,#56083,#56084);
#44849=AXIS2_PLACEMENT_3D('',#88736,#56085,#56086);
#44850=AXIS2_PLACEMENT_3D('',#88769,#56088,#56089);
#44851=AXIS2_PLACEMENT_3D('',#88827,#56090,#56091);
#44852=AXIS2_PLACEMENT_3D('',#88854,#56092,#56093);
#44853=AXIS2_PLACEMENT_3D('',#88855,#56094,#56095);
#44854=AXIS2_PLACEMENT_3D('',#88868,#56096,#56097);
#44855=AXIS2_PLACEMENT_3D('',#88877,#56098,#56099);
#44856=AXIS2_PLACEMENT_3D('',#88879,#56101,#56102);
#44857=AXIS2_PLACEMENT_3D('',#88892,#56103,#56104);
#44858=AXIS2_PLACEMENT_3D('',#88901,#56105,#56106);
#44859=AXIS2_PLACEMENT_3D('',#88903,#56108,#56109);
#44860=AXIS2_PLACEMENT_3D('',#88906,#56110,#56111);
#44861=AXIS2_PLACEMENT_3D('',#88910,#56113,#56114);
#44862=AXIS2_PLACEMENT_3D('',#88912,#56116,#56117);
#44863=AXIS2_PLACEMENT_3D('',#88918,#56121,#56122);
#44864=AXIS2_PLACEMENT_3D('',#88927,#56123,#56124);
#44865=AXIS2_PLACEMENT_3D('',#88942,#56125,#56126);
#44866=AXIS2_PLACEMENT_3D('',#88957,#56127,#56128);
#44867=AXIS2_PLACEMENT_3D('',#88967,#56130,#56131);
#44868=AXIS2_PLACEMENT_3D('',#88971,#56133,#56134);
#44869=AXIS2_PLACEMENT_3D('',#88975,#56136,#56137);
#44870=AXIS2_PLACEMENT_3D('',#88979,#56139,#56140);
#44871=AXIS2_PLACEMENT_3D('',#88983,#56142,#56143);
#44872=AXIS2_PLACEMENT_3D('',#88987,#56145,#56146);
#44873=AXIS2_PLACEMENT_3D('',#88991,#56148,#56149);
#44874=AXIS2_PLACEMENT_3D('',#88995,#56151,#56152);
#44875=AXIS2_PLACEMENT_3D('',#88999,#56154,#56155);
#44876=AXIS2_PLACEMENT_3D('',#89003,#56157,#56158);
#44877=AXIS2_PLACEMENT_3D('',#89007,#56160,#56161);
#44878=AXIS2_PLACEMENT_3D('',#89011,#56163,#56164);
#44879=AXIS2_PLACEMENT_3D('',#89015,#56166,#56167);
#44880=AXIS2_PLACEMENT_3D('',#89019,#56169,#56170);
#44881=AXIS2_PLACEMENT_3D('',#89023,#56172,#56173);
#44882=AXIS2_PLACEMENT_3D('',#89027,#56175,#56176);
#44883=AXIS2_PLACEMENT_3D('',#89031,#56178,#56179);
#44884=AXIS2_PLACEMENT_3D('',#89035,#56181,#56182);
#44885=AXIS2_PLACEMENT_3D('',#89039,#56184,#56185);
#44886=AXIS2_PLACEMENT_3D('',#89043,#56187,#56188);
#44887=AXIS2_PLACEMENT_3D('',#89047,#56190,#56191);
#44888=AXIS2_PLACEMENT_3D('',#89051,#56193,#56194);
#44889=AXIS2_PLACEMENT_3D('',#89055,#56196,#56197);
#44890=AXIS2_PLACEMENT_3D('',#89059,#56199,#56200);
#44891=AXIS2_PLACEMENT_3D('',#89063,#56202,#56203);
#44892=AXIS2_PLACEMENT_3D('',#89067,#56205,#56206);
#44893=AXIS2_PLACEMENT_3D('',#89071,#56208,#56209);
#44894=AXIS2_PLACEMENT_3D('',#89075,#56211,#56212);
#44895=AXIS2_PLACEMENT_3D('',#89079,#56214,#56215);
#44896=AXIS2_PLACEMENT_3D('',#89083,#56217,#56218);
#44897=AXIS2_PLACEMENT_3D('',#89087,#56220,#56221);
#44898=AXIS2_PLACEMENT_3D('',#89091,#56223,#56224);
#44899=AXIS2_PLACEMENT_3D('',#89095,#56226,#56227);
#44900=AXIS2_PLACEMENT_3D('',#89099,#56229,#56230);
#44901=AXIS2_PLACEMENT_3D('',#89103,#56232,#56233);
#44902=AXIS2_PLACEMENT_3D('',#89107,#56235,#56236);
#44903=AXIS2_PLACEMENT_3D('',#89111,#56238,#56239);
#44904=AXIS2_PLACEMENT_3D('',#89115,#56241,#56242);
#44905=AXIS2_PLACEMENT_3D('',#89119,#56244,#56245);
#44906=AXIS2_PLACEMENT_3D('',#89123,#56247,#56248);
#44907=AXIS2_PLACEMENT_3D('',#89127,#56250,#56251);
#44908=AXIS2_PLACEMENT_3D('',#89131,#56253,#56254);
#44909=AXIS2_PLACEMENT_3D('',#89135,#56256,#56257);
#44910=AXIS2_PLACEMENT_3D('',#89139,#56259,#56260);
#44911=AXIS2_PLACEMENT_3D('',#89143,#56262,#56263);
#44912=AXIS2_PLACEMENT_3D('',#89147,#56265,#56266);
#44913=AXIS2_PLACEMENT_3D('',#89151,#56268,#56269);
#44914=AXIS2_PLACEMENT_3D('',#89155,#56271,#56272);
#44915=AXIS2_PLACEMENT_3D('',#89159,#56274,#56275);
#44916=AXIS2_PLACEMENT_3D('',#89163,#56277,#56278);
#44917=AXIS2_PLACEMENT_3D('',#89167,#56280,#56281);
#44918=AXIS2_PLACEMENT_3D('',#89171,#56283,#56284);
#44919=AXIS2_PLACEMENT_3D('',#89175,#56286,#56287);
#44920=AXIS2_PLACEMENT_3D('',#89179,#56289,#56290);
#44921=AXIS2_PLACEMENT_3D('',#89183,#56292,#56293);
#44922=AXIS2_PLACEMENT_3D('',#89187,#56295,#56296);
#44923=AXIS2_PLACEMENT_3D('',#89191,#56298,#56299);
#44924=AXIS2_PLACEMENT_3D('',#89195,#56301,#56302);
#44925=AXIS2_PLACEMENT_3D('',#89199,#56304,#56305);
#44926=AXIS2_PLACEMENT_3D('',#89203,#56307,#56308);
#44927=AXIS2_PLACEMENT_3D('',#89207,#56310,#56311);
#44928=AXIS2_PLACEMENT_3D('',#89211,#56313,#56314);
#44929=AXIS2_PLACEMENT_3D('',#89215,#56316,#56317);
#44930=AXIS2_PLACEMENT_3D('',#89219,#56319,#56320);
#44931=AXIS2_PLACEMENT_3D('',#89223,#56322,#56323);
#44932=AXIS2_PLACEMENT_3D('',#89227,#56325,#56326);
#44933=AXIS2_PLACEMENT_3D('',#89231,#56328,#56329);
#44934=AXIS2_PLACEMENT_3D('',#89235,#56331,#56332);
#44935=AXIS2_PLACEMENT_3D('',#89239,#56334,#56335);
#44936=AXIS2_PLACEMENT_3D('',#89243,#56337,#56338);
#44937=AXIS2_PLACEMENT_3D('',#89246,#56340,#56341);
#44938=AXIS2_PLACEMENT_3D('',#89247,#56342,#56343);
#44939=AXIS2_PLACEMENT_3D('',#89251,#56345,#56346);
#44940=AXIS2_PLACEMENT_3D('',#89253,#56348,#56349);
#44941=AXIS2_PLACEMENT_3D('',#89257,#56352,#56353);
#44942=AXIS2_PLACEMENT_3D('',#89266,#56354,#56355);
#44943=AXIS2_PLACEMENT_3D('',#89281,#56356,#56357);
#44944=AXIS2_PLACEMENT_3D('',#89296,#56358,#56359);
#44945=AXIS2_PLACEMENT_3D('',#89304,#56360,#56361);
#44946=AXIS2_PLACEMENT_3D('',#89308,#56363,#56364);
#44947=AXIS2_PLACEMENT_3D('',#89312,#56366,#56367);
#44948=AXIS2_PLACEMENT_3D('',#89316,#56369,#56370);
#44949=AXIS2_PLACEMENT_3D('',#89320,#56372,#56373);
#44950=AXIS2_PLACEMENT_3D('',#89324,#56375,#56376);
#44951=AXIS2_PLACEMENT_3D('',#89328,#56378,#56379);
#44952=AXIS2_PLACEMENT_3D('',#89332,#56381,#56382);
#44953=AXIS2_PLACEMENT_3D('',#89336,#56384,#56385);
#44954=AXIS2_PLACEMENT_3D('',#89340,#56387,#56388);
#44955=AXIS2_PLACEMENT_3D('',#89344,#56390,#56391);
#44956=AXIS2_PLACEMENT_3D('',#89348,#56393,#56394);
#44957=AXIS2_PLACEMENT_3D('',#89352,#56396,#56397);
#44958=AXIS2_PLACEMENT_3D('',#89356,#56399,#56400);
#44959=AXIS2_PLACEMENT_3D('',#89360,#56402,#56403);
#44960=AXIS2_PLACEMENT_3D('',#89364,#56405,#56406);
#44961=AXIS2_PLACEMENT_3D('',#89368,#56408,#56409);
#44962=AXIS2_PLACEMENT_3D('',#89372,#56411,#56412);
#44963=AXIS2_PLACEMENT_3D('',#89376,#56414,#56415);
#44964=AXIS2_PLACEMENT_3D('',#89380,#56417,#56418);
#44965=AXIS2_PLACEMENT_3D('',#89384,#56420,#56421);
#44966=AXIS2_PLACEMENT_3D('',#89388,#56423,#56424);
#44967=AXIS2_PLACEMENT_3D('',#89392,#56426,#56427);
#44968=AXIS2_PLACEMENT_3D('',#89396,#56429,#56430);
#44969=AXIS2_PLACEMENT_3D('',#89400,#56432,#56433);
#44970=AXIS2_PLACEMENT_3D('',#89404,#56435,#56436);
#44971=AXIS2_PLACEMENT_3D('',#89408,#56438,#56439);
#44972=AXIS2_PLACEMENT_3D('',#89412,#56441,#56442);
#44973=AXIS2_PLACEMENT_3D('',#89416,#56444,#56445);
#44974=AXIS2_PLACEMENT_3D('',#89420,#56447,#56448);
#44975=AXIS2_PLACEMENT_3D('',#89424,#56450,#56451);
#44976=AXIS2_PLACEMENT_3D('',#89428,#56453,#56454);
#44977=AXIS2_PLACEMENT_3D('',#89432,#56456,#56457);
#44978=AXIS2_PLACEMENT_3D('',#89436,#56459,#56460);
#44979=AXIS2_PLACEMENT_3D('',#89440,#56462,#56463);
#44980=AXIS2_PLACEMENT_3D('',#89444,#56465,#56466);
#44981=AXIS2_PLACEMENT_3D('',#89448,#56468,#56469);
#44982=AXIS2_PLACEMENT_3D('',#89452,#56471,#56472);
#44983=AXIS2_PLACEMENT_3D('',#89456,#56474,#56475);
#44984=AXIS2_PLACEMENT_3D('',#89460,#56477,#56478);
#44985=AXIS2_PLACEMENT_3D('',#89464,#56480,#56481);
#44986=AXIS2_PLACEMENT_3D('',#89468,#56483,#56484);
#44987=AXIS2_PLACEMENT_3D('',#89472,#56486,#56487);
#44988=AXIS2_PLACEMENT_3D('',#89476,#56489,#56490);
#44989=AXIS2_PLACEMENT_3D('',#89480,#56492,#56493);
#44990=AXIS2_PLACEMENT_3D('',#89484,#56495,#56496);
#44991=AXIS2_PLACEMENT_3D('',#89488,#56498,#56499);
#44992=AXIS2_PLACEMENT_3D('',#89492,#56501,#56502);
#44993=AXIS2_PLACEMENT_3D('',#89496,#56504,#56505);
#44994=AXIS2_PLACEMENT_3D('',#89500,#56507,#56508);
#44995=AXIS2_PLACEMENT_3D('',#89504,#56510,#56511);
#44996=AXIS2_PLACEMENT_3D('',#89508,#56513,#56514);
#44997=AXIS2_PLACEMENT_3D('',#89512,#56516,#56517);
#44998=AXIS2_PLACEMENT_3D('',#89516,#56519,#56520);
#44999=AXIS2_PLACEMENT_3D('',#89520,#56522,#56523);
#45000=AXIS2_PLACEMENT_3D('',#89524,#56525,#56526);
#45001=AXIS2_PLACEMENT_3D('',#89528,#56528,#56529);
#45002=AXIS2_PLACEMENT_3D('',#89532,#56531,#56532);
#45003=AXIS2_PLACEMENT_3D('',#89536,#56534,#56535);
#45004=AXIS2_PLACEMENT_3D('',#89540,#56537,#56538);
#45005=AXIS2_PLACEMENT_3D('',#89544,#56540,#56541);
#45006=AXIS2_PLACEMENT_3D('',#89548,#56543,#56544);
#45007=AXIS2_PLACEMENT_3D('',#89552,#56546,#56547);
#45008=AXIS2_PLACEMENT_3D('',#89556,#56549,#56550);
#45009=AXIS2_PLACEMENT_3D('',#89560,#56552,#56553);
#45010=AXIS2_PLACEMENT_3D('',#89564,#56555,#56556);
#45011=AXIS2_PLACEMENT_3D('',#89568,#56558,#56559);
#45012=AXIS2_PLACEMENT_3D('',#89572,#56561,#56562);
#45013=AXIS2_PLACEMENT_3D('',#89576,#56564,#56565);
#45014=AXIS2_PLACEMENT_3D('',#89579,#56567,#56568);
#45015=AXIS2_PLACEMENT_3D('',#89581,#56570,#56571);
#45016=AXIS2_PLACEMENT_3D('',#89584,#56574,#56575);
#45017=AXIS2_PLACEMENT_3D('',#89586,#56577,#56578);
#45018=AXIS2_PLACEMENT_3D('',#89588,#56580,#56581);
#45019=AXIS2_PLACEMENT_3D('',#89591,#56584,#56585);
#45020=AXIS2_PLACEMENT_3D('',#89593,#56587,#56588);
#45021=AXIS2_PLACEMENT_3D('',#89596,#56591,#56592);
#45022=AXIS2_PLACEMENT_3D('',#89598,#56594,#56595);
#45023=AXIS2_PLACEMENT_3D('',#89601,#56598,#56599);
#45024=AXIS2_PLACEMENT_3D('',#89603,#56601,#56602);
#45025=AXIS2_PLACEMENT_3D('',#89605,#56604,#56605);
#45026=AXIS2_PLACEMENT_3D('',#89608,#56608,#56609);
#45027=AXIS2_PLACEMENT_3D('',#89610,#56611,#56612);
#45028=AXIS2_PLACEMENT_3D('',#89612,#56614,#56615);
#45029=AXIS2_PLACEMENT_3D('',#89615,#56618,#56619);
#45030=AXIS2_PLACEMENT_3D('',#89617,#56621,#56622);
#45031=AXIS2_PLACEMENT_3D('',#89620,#56625,#56626);
#45032=AXIS2_PLACEMENT_3D('',#89622,#56628,#56629);
#45033=AXIS2_PLACEMENT_3D('',#89625,#56632,#56633);
#45034=AXIS2_PLACEMENT_3D('',#89627,#56635,#56636);
#45035=AXIS2_PLACEMENT_3D('',#89629,#56638,#56639);
#45036=AXIS2_PLACEMENT_3D('',#89632,#56642,#56643);
#45037=AXIS2_PLACEMENT_3D('',#89634,#56645,#56646);
#45038=AXIS2_PLACEMENT_3D('',#89636,#56648,#56649);
#45039=AXIS2_PLACEMENT_3D('',#89639,#56652,#56653);
#45040=AXIS2_PLACEMENT_3D('',#89641,#56655,#56656);
#45041=AXIS2_PLACEMENT_3D('',#89644,#56659,#56660);
#45042=AXIS2_PLACEMENT_3D('',#89646,#56662,#56663);
#45043=AXIS2_PLACEMENT_3D('',#89649,#56666,#56667);
#45044=AXIS2_PLACEMENT_3D('',#89651,#56669,#56670);
#45045=AXIS2_PLACEMENT_3D('',#89653,#56672,#56673);
#45046=AXIS2_PLACEMENT_3D('',#89656,#56676,#56677);
#45047=AXIS2_PLACEMENT_3D('',#89658,#56679,#56680);
#45048=AXIS2_PLACEMENT_3D('',#89660,#56682,#56683);
#45049=AXIS2_PLACEMENT_3D('',#89663,#56686,#56687);
#45050=AXIS2_PLACEMENT_3D('',#89665,#56689,#56690);
#45051=AXIS2_PLACEMENT_3D('',#89668,#56693,#56694);
#45052=AXIS2_PLACEMENT_3D('',#89670,#56696,#56697);
#45053=AXIS2_PLACEMENT_3D('',#89673,#56700,#56701);
#45054=AXIS2_PLACEMENT_3D('',#89675,#56703,#56704);
#45055=AXIS2_PLACEMENT_3D('',#89677,#56706,#56707);
#45056=AXIS2_PLACEMENT_3D('',#89680,#56710,#56711);
#45057=AXIS2_PLACEMENT_3D('',#89682,#56713,#56714);
#45058=AXIS2_PLACEMENT_3D('',#89684,#56716,#56717);
#45059=AXIS2_PLACEMENT_3D('',#89687,#56720,#56721);
#45060=AXIS2_PLACEMENT_3D('',#89689,#56723,#56724);
#45061=AXIS2_PLACEMENT_3D('',#89692,#56727,#56728);
#45062=AXIS2_PLACEMENT_3D('',#89694,#56730,#56731);
#45063=AXIS2_PLACEMENT_3D('',#89697,#56734,#56735);
#45064=AXIS2_PLACEMENT_3D('',#89699,#56737,#56738);
#45065=AXIS2_PLACEMENT_3D('',#89701,#56740,#56741);
#45066=AXIS2_PLACEMENT_3D('',#89704,#56744,#56745);
#45067=AXIS2_PLACEMENT_3D('',#89706,#56747,#56748);
#45068=AXIS2_PLACEMENT_3D('',#89708,#56750,#56751);
#45069=AXIS2_PLACEMENT_3D('',#89709,#56752,#56753);
#45070=AXIS2_PLACEMENT_3D('',#89710,#56754,#56755);
#45071=AXIS2_PLACEMENT_3D('',#89711,#56756,#56757);
#45072=AXIS2_PLACEMENT_3D('',#89712,#56758,#56759);
#45073=AXIS2_PLACEMENT_3D('',#89713,#56760,#56761);
#45074=AXIS2_PLACEMENT_3D('',#89716,#56764,#56765);
#45075=AXIS2_PLACEMENT_3D('',#89718,#56767,#56768);
#45076=AXIS2_PLACEMENT_3D('',#89721,#56771,#56772);
#45077=AXIS2_PLACEMENT_3D('',#89723,#56774,#56775);
#45078=AXIS2_PLACEMENT_3D('',#89726,#56778,#56779);
#45079=AXIS2_PLACEMENT_3D('',#89728,#56781,#56782);
#45080=AXIS2_PLACEMENT_3D('',#89730,#56784,#56785);
#45081=AXIS2_PLACEMENT_3D('',#89733,#56788,#56789);
#45082=AXIS2_PLACEMENT_3D('',#89735,#56791,#56792);
#45083=AXIS2_PLACEMENT_3D('',#89737,#56794,#56795);
#45084=AXIS2_PLACEMENT_3D('',#89738,#56796,#56797);
#45085=AXIS2_PLACEMENT_3D('',#89739,#56798,#56799);
#45086=AXIS2_PLACEMENT_3D('',#89740,#56800,#56801);
#45087=AXIS2_PLACEMENT_3D('',#89741,#56802,#56803);
#45088=AXIS2_PLACEMENT_3D('',#89742,#56804,#56805);
#45089=AXIS2_PLACEMENT_3D('',#89743,#56806,#56807);
#45090=AXIS2_PLACEMENT_3D('',#89744,#56808,#56809);
#45091=AXIS2_PLACEMENT_3D('',#89745,#56810,#56811);
#45092=AXIS2_PLACEMENT_3D('',#89746,#56812,#56813);
#45093=AXIS2_PLACEMENT_3D('',#89749,#56816,#56817);
#45094=AXIS2_PLACEMENT_3D('',#89751,#56819,#56820);
#45095=AXIS2_PLACEMENT_3D('',#89754,#56823,#56824);
#45096=AXIS2_PLACEMENT_3D('',#89756,#56826,#56827);
#45097=AXIS2_PLACEMENT_3D('',#89757,#56828,#56829);
#45098=AXIS2_PLACEMENT_3D('',#89758,#56830,#56831);
#45099=AXIS2_PLACEMENT_3D('',#89759,#56832,#56833);
#45100=AXIS2_PLACEMENT_3D('',#89760,#56834,#56835);
#45101=AXIS2_PLACEMENT_3D('',#89761,#56836,#56837);
#45102=AXIS2_PLACEMENT_3D('',#89762,#56838,#56839);
#45103=AXIS2_PLACEMENT_3D('',#89763,#56840,#56841);
#45104=AXIS2_PLACEMENT_3D('',#89764,#56842,#56843);
#45105=AXIS2_PLACEMENT_3D('',#89765,#56844,#56845);
#45106=AXIS2_PLACEMENT_3D('',#89766,#56846,#56847);
#45107=AXIS2_PLACEMENT_3D('',#89767,#56848,#56849);
#45108=AXIS2_PLACEMENT_3D('',#89816,#56850,#56851);
#45109=AXIS2_PLACEMENT_3D('',#89817,#56852,#56853);
#45110=AXIS2_PLACEMENT_3D('',#89818,#56854,#56855);
#45111=AXIS2_PLACEMENT_3D('',#89819,#56856,#56857);
#45112=AXIS2_PLACEMENT_3D('',#89868,#56858,#56859);
#45113=AXIS2_PLACEMENT_3D('',#89869,#56860,#56861);
#45114=AXIS2_PLACEMENT_3D('',#89870,#56862,#56863);
#45115=AXIS2_PLACEMENT_3D('',#89871,#56864,#56865);
#45116=AXIS2_PLACEMENT_3D('',#89920,#56866,#56867);
#45117=AXIS2_PLACEMENT_3D('',#89921,#56868,#56869);
#45118=AXIS2_PLACEMENT_3D('',#89922,#56870,#56871);
#45119=AXIS2_PLACEMENT_3D('',#89925,#56874,#56875);
#45120=AXIS2_PLACEMENT_3D('',#89927,#56877,#56878);
#45121=AXIS2_PLACEMENT_3D('',#89929,#56880,#56881);
#45122=AXIS2_PLACEMENT_3D('',#89932,#56884,#56885);
#45123=AXIS2_PLACEMENT_3D('',#89934,#56887,#56888);
#45124=AXIS2_PLACEMENT_3D('',#89937,#56891,#56892);
#45125=AXIS2_PLACEMENT_3D('',#89939,#56894,#56895);
#45126=AXIS2_PLACEMENT_3D('',#89940,#56896,#56897);
#45127=AXIS2_PLACEMENT_3D('',#89941,#56898,#56899);
#45128=AXIS2_PLACEMENT_3D('',#89990,#56900,#56901);
#45129=AXIS2_PLACEMENT_3D('',#89991,#56902,#56903);
#45130=AXIS2_PLACEMENT_3D('',#89992,#56904,#56905);
#45131=AXIS2_PLACEMENT_3D('',#90041,#56906,#56907);
#45132=AXIS2_PLACEMENT_3D('',#90042,#56908,#56909);
#45133=AXIS2_PLACEMENT_3D('',#90043,#56910,#56911);
#45134=AXIS2_PLACEMENT_3D('',#90092,#56912,#56913);
#45135=AXIS2_PLACEMENT_3D('',#90095,#56916,#56917);
#45136=AXIS2_PLACEMENT_3D('',#90097,#56919,#56920);
#45137=AXIS2_PLACEMENT_3D('',#90099,#56922,#56923);
#45138=AXIS2_PLACEMENT_3D('',#90101,#56925,#56926);
#45139=AXIS2_PLACEMENT_3D('',#90103,#56928,#56929);
#45140=AXIS2_PLACEMENT_3D('',#90104,#56930,#56931);
#45141=AXIS2_PLACEMENT_3D('',#90105,#56932,#56933);
#45142=AXIS2_PLACEMENT_3D('',#90106,#56934,#56935);
#45143=AXIS2_PLACEMENT_3D('',#90108,#56937,#56938);
#45144=AXIS2_PLACEMENT_3D('',#90110,#56940,#56941);
#45145=AXIS2_PLACEMENT_3D('',#90111,#56942,#56943);
#45146=AXIS2_PLACEMENT_3D('',#90112,#56944,#56945);
#45147=AXIS2_PLACEMENT_3D('',#90113,#56946,#56947);
#45148=AXIS2_PLACEMENT_3D('',#90115,#56949,#56950);
#45149=AXIS2_PLACEMENT_3D('',#90117,#56952,#56953);
#45150=AXIS2_PLACEMENT_3D('',#90118,#56954,#56955);
#45151=AXIS2_PLACEMENT_3D('',#90120,#56957,#56958);
#45152=AXIS2_PLACEMENT_3D('',#90122,#56960,#56961);
#45153=AXIS2_PLACEMENT_3D('',#90123,#56962,#56963);
#45154=AXIS2_PLACEMENT_3D('',#90124,#56964,#56965);
#45155=AXIS2_PLACEMENT_3D('',#90125,#56966,#56967);
#45156=AXIS2_PLACEMENT_3D('',#90127,#56969,#56970);
#45157=AXIS2_PLACEMENT_3D('',#90129,#56972,#56973);
#45158=AXIS2_PLACEMENT_3D('',#90130,#56974,#56975);
#45159=AXIS2_PLACEMENT_3D('',#90132,#56977,#56978);
#45160=AXIS2_PLACEMENT_3D('',#90134,#56980,#56981);
#45161=AXIS2_PLACEMENT_3D('',#90135,#56982,#56983);
#45162=AXIS2_PLACEMENT_3D('',#90136,#56984,#56985);
#45163=AXIS2_PLACEMENT_3D('',#90137,#56986,#56987);
#45164=AXIS2_PLACEMENT_3D('',#90139,#56989,#56990);
#45165=AXIS2_PLACEMENT_3D('',#90141,#56992,#56993);
#45166=AXIS2_PLACEMENT_3D('',#90142,#56994,#56995);
#45167=AXIS2_PLACEMENT_3D('',#90144,#56997,#56998);
#45168=AXIS2_PLACEMENT_3D('',#90146,#57000,#57001);
#45169=AXIS2_PLACEMENT_3D('',#90147,#57002,#57003);
#45170=AXIS2_PLACEMENT_3D('',#90148,#57004,#57005);
#45171=AXIS2_PLACEMENT_3D('',#90149,#57006,#57007);
#45172=AXIS2_PLACEMENT_3D('',#90151,#57009,#57010);
#45173=AXIS2_PLACEMENT_3D('',#90153,#57012,#57013);
#45174=AXIS2_PLACEMENT_3D('',#90154,#57014,#57015);
#45175=AXIS2_PLACEMENT_3D('',#90156,#57017,#57018);
#45176=AXIS2_PLACEMENT_3D('',#90158,#57020,#57021);
#45177=AXIS2_PLACEMENT_3D('',#90159,#57022,#57023);
#45178=AXIS2_PLACEMENT_3D('',#90160,#57024,#57025);
#45179=AXIS2_PLACEMENT_3D('',#90161,#57026,#57027);
#45180=AXIS2_PLACEMENT_3D('',#90163,#57029,#57030);
#45181=AXIS2_PLACEMENT_3D('',#90165,#57032,#57033);
#45182=AXIS2_PLACEMENT_3D('',#90166,#57034,#57035);
#45183=AXIS2_PLACEMENT_3D('',#90168,#57037,#57038);
#45184=AXIS2_PLACEMENT_3D('',#90170,#57040,#57041);
#45185=AXIS2_PLACEMENT_3D('',#90171,#57042,#57043);
#45186=AXIS2_PLACEMENT_3D('',#90172,#57044,#57045);
#45187=AXIS2_PLACEMENT_3D('',#90173,#57046,#57047);
#45188=AXIS2_PLACEMENT_3D('',#90175,#57049,#57050);
#45189=AXIS2_PLACEMENT_3D('',#90177,#57052,#57053);
#45190=AXIS2_PLACEMENT_3D('',#90178,#57054,#57055);
#45191=AXIS2_PLACEMENT_3D('',#90180,#57057,#57058);
#45192=AXIS2_PLACEMENT_3D('',#90182,#57060,#57061);
#45193=AXIS2_PLACEMENT_3D('',#90183,#57062,#57063);
#45194=AXIS2_PLACEMENT_3D('',#90184,#57064,#57065);
#45195=AXIS2_PLACEMENT_3D('',#90185,#57066,#57067);
#45196=AXIS2_PLACEMENT_3D('',#90187,#57069,#57070);
#45197=AXIS2_PLACEMENT_3D('',#90189,#57072,#57073);
#45198=AXIS2_PLACEMENT_3D('',#90190,#57074,#57075);
#45199=AXIS2_PLACEMENT_3D('',#90191,#57076,#57077);
#45200=AXIS2_PLACEMENT_3D('',#90192,#57078,#57079);
#55999=DIRECTION('axis',(0.,0.,1.));
#56000=DIRECTION('refdir',(1.,0.,0.));
#56001=DIRECTION('center_axis',(0.,1.,0.));
#56002=DIRECTION('ref_axis',(0.,0.,1.));
#56003=DIRECTION('center_axis',(0.,-1.,0.));
#56004=DIRECTION('ref_axis',(1.,0.,0.));
#56005=DIRECTION('center_axis',(-1.,0.,0.));
#56006=DIRECTION('ref_axis',(0.,0.,-1.));
#56007=DIRECTION('center_axis',(0.,1.,0.));
#56008=DIRECTION('ref_axis',(1.,0.,0.));
#56009=DIRECTION('center_axis',(0.,1.,0.));
#56010=DIRECTION('ref_axis',(1.,0.,0.));
#56011=DIRECTION('center_axis',(0.,1.,0.));
#56012=DIRECTION('ref_axis',(1.,0.,0.));
#56013=DIRECTION('',(0.,-1.,0.));
#56014=DIRECTION('center_axis',(0.,-1.,0.));
#56015=DIRECTION('ref_axis',(0.,0.,1.));
#56016=DIRECTION('center_axis',(0.,-1.,0.));
#56017=DIRECTION('ref_axis',(0.,0.,-1.));
#56018=DIRECTION('center_axis',(0.,1.,0.));
#56019=DIRECTION('ref_axis',(1.,0.,0.));
#56020=DIRECTION('center_axis',(0.,1.,0.));
#56021=DIRECTION('ref_axis',(0.,0.,1.));
#56022=DIRECTION('center_axis',(0.,1.,0.));
#56023=DIRECTION('ref_axis',(0.,0.,1.));
#56024=DIRECTION('center_axis',(0.,1.,0.));
#56025=DIRECTION('ref_axis',(1.,0.,0.));
#56026=DIRECTION('',(-1.,0.,0.));
#56027=DIRECTION('center_axis',(0.,1.,0.));
#56028=DIRECTION('ref_axis',(0.,0.,-1.));
#56029=DIRECTION('center_axis',(0.,1.,0.));
#56030=DIRECTION('ref_axis',(0.,0.,-1.));
#56031=DIRECTION('center_axis',(0.,1.,0.));
#56032=DIRECTION('ref_axis',(1.,0.,0.));
#56033=DIRECTION('',(1.,0.,0.));
#56034=DIRECTION('center_axis',(1.,0.,0.));
#56035=DIRECTION('ref_axis',(0.,0.499999999999999,0.866025403784439));
#56036=DIRECTION('center_axis',(1.,0.,0.));
#56037=DIRECTION('ref_axis',(0.,0.5,0.866025403784438));
#56038=DIRECTION('center_axis',(-1.,0.,0.));
#56039=DIRECTION('ref_axis',(0.,0.5,0.866025403784438));
#56040=DIRECTION('center_axis',(1.,0.,0.));
#56041=DIRECTION('ref_axis',(0.,1.,0.));
#56042=DIRECTION('center_axis',(-1.,0.,0.));
#56043=DIRECTION('ref_axis',(0.,0.5,0.866025403784438));
#56044=DIRECTION('',(1.,0.,0.));
#56045=DIRECTION('center_axis',(0.,-0.5,0.866025403784439));
#56046=DIRECTION('ref_axis',(1.,0.,0.));
#56047=DIRECTION('center_axis',(0.,0.5,-0.866025403784439));
#56048=DIRECTION('ref_axis',(1.,5.62747233509627E-17,3.249022667525E-17));
#56049=DIRECTION('center_axis',(0.,-0.866025403784439,-0.5));
#56050=DIRECTION('ref_axis',(-1.,0.,0.));
#56051=DIRECTION('center_axis',(0.,-0.5,0.866025403784439));
#56052=DIRECTION('ref_axis',(1.,6.16790569236199E-17,2.31296463463575E-17));
#56053=DIRECTION('center_axis',(0.,-0.5,0.866025403784439));
#56054=DIRECTION('ref_axis',(1.,0.,0.));
#56055=DIRECTION('',(0.,0.5,-0.866025403784439));
#56056=DIRECTION('center_axis',(0.,0.5,-0.866025403784439));
#56057=DIRECTION('ref_axis',(0.,-0.866025403784439,-0.5));
#56058=DIRECTION('center_axis',(0.,0.5,-0.866025403784439));
#56059=DIRECTION('ref_axis',(0.,0.866025403784439,0.5));
#56060=DIRECTION('center_axis',(0.,-0.5,0.866025403784439));
#56061=DIRECTION('ref_axis',(1.,0.,0.));
#56062=DIRECTION('center_axis',(0.,-0.5,0.866025403784439));
#56063=DIRECTION('ref_axis',(1.,0.,0.));
#56064=DIRECTION('center_axis',(0.,-0.5,0.866025403784439));
#56065=DIRECTION('ref_axis',(0.,0.866025403784439,0.5));
#56066=DIRECTION('center_axis',(0.,-0.5,0.866025403784439));
#56067=DIRECTION('ref_axis',(1.,0.,0.));
#56068=DIRECTION('center_axis',(0.,-0.5,0.866025403784439));
#56069=DIRECTION('ref_axis',(1.,0.,0.));
#56070=DIRECTION('center_axis',(0.,-0.5,0.866025403784439));
#56071=DIRECTION('ref_axis',(0.,-0.866025403784439,-0.5));
#56072=DIRECTION('center_axis',(0.,-0.5,0.866025403784439));
#56073=DIRECTION('ref_axis',(1.,0.,0.));
#56074=DIRECTION('',(-1.,0.,0.));
#56075=DIRECTION('center_axis',(0.,-0.5,-0.866025403784438));
#56076=DIRECTION('ref_axis',(-1.,0.,0.));
#56077=DIRECTION('center_axis',(0.,0.5,0.866025403784438));
#56078=DIRECTION('ref_axis',(1.,8.36373887689785E-17,-4.82880689200872E-17));
#56079=DIRECTION('center_axis',(0.,-0.866025403784438,0.5));
#56080=DIRECTION('ref_axis',(1.,0.,0.));
#56081=DIRECTION('center_axis',(0.,-0.5,-0.866025403784438));
#56082=DIRECTION('ref_axis',(1.,8.48087032699774E-17,-4.62592926927149E-17));
#56083=DIRECTION('center_axis',(0.,-0.5,-0.866025403784438));
#56084=DIRECTION('ref_axis',(1.,8.48087032699774E-17,-4.62592926927149E-17));
#56085=DIRECTION('center_axis',(0.,-0.5,-0.866025403784438));
#56086=DIRECTION('ref_axis',(1.,0.,0.));
#56087=DIRECTION('',(0.,0.5,0.866025403784438));
#56088=DIRECTION('center_axis',(0.,0.5,0.866025403784438));
#56089=DIRECTION('ref_axis',(0.,0.866025403784438,-0.5));
#56090=DIRECTION('center_axis',(0.,0.5,0.866025403784438));
#56091=DIRECTION('ref_axis',(0.,-0.866025403784438,0.5));
#56092=DIRECTION('center_axis',(0.,-0.5,-0.866025403784438));
#56093=DIRECTION('ref_axis',(1.,0.,0.));
#56094=DIRECTION('center_axis',(0.,-0.5,-0.866025403784438));
#56095=DIRECTION('ref_axis',(-1.,0.,0.));
#56096=DIRECTION('center_axis',(0.,-0.5,-0.866025403784438));
#56097=DIRECTION('ref_axis',(0.,0.866025403784438,-0.500000000000001));
#56098=DIRECTION('center_axis',(0.,-0.5,-0.866025403784438));
#56099=DIRECTION('ref_axis',(1.,0.,0.));
#56100=DIRECTION('',(-1.,0.,0.));
#56101=DIRECTION('center_axis',(0.,-0.5,-0.866025403784438));
#56102=DIRECTION('ref_axis',(-1.,0.,0.));
#56103=DIRECTION('center_axis',(0.,-0.5,-0.866025403784438));
#56104=DIRECTION('ref_axis',(0.,-0.866025403784438,0.500000000000001));
#56105=DIRECTION('center_axis',(0.,-0.5,-0.866025403784438));
#56106=DIRECTION('ref_axis',(1.,0.,0.));
#56107=DIRECTION('',(1.,0.,0.));
#56108=DIRECTION('center_axis',(1.,0.,0.));
#56109=DIRECTION('ref_axis',(0.,-0.707106781186548,0.707106781186547));
#56110=DIRECTION('center_axis',(-1.,0.,0.));
#56111=DIRECTION('ref_axis',(0.,-0.707106781186548,0.707106781186547));
#56112=DIRECTION('',(-1.,0.,0.));
#56113=DIRECTION('center_axis',(1.,0.,0.));
#56114=DIRECTION('ref_axis',(0.,-0.707106781186548,0.707106781186547));
#56115=DIRECTION('',(1.,0.,0.));
#56116=DIRECTION('center_axis',(0.,0.,1.));
#56117=DIRECTION('ref_axis',(0.,-1.,0.));
#56118=DIRECTION('',(0.,-1.,0.));
#56119=DIRECTION('',(1.,0.,0.));
#56120=DIRECTION('',(0.,-1.,0.));
#56121=DIRECTION('center_axis',(1.,0.,0.));
#56122=DIRECTION('ref_axis',(0.,0.,-1.));
#56123=DIRECTION('center_axis',(-1.,0.,0.));
#56124=DIRECTION('ref_axis',(0.,-1.,-1.06397713344143E-13));
#56125=DIRECTION('center_axis',(-1.,0.,0.));
#56126=DIRECTION('ref_axis',(0.,0.500000000000038,-0.866025403784417));
#56127=DIRECTION('center_axis',(-1.,0.,0.));
#56128=DIRECTION('ref_axis',(0.,0.499999999999946,0.86602540378447));
#56129=DIRECTION('',(0.,0.,-1.));
#56130=DIRECTION('center_axis',(-1.,0.,0.));
#56131=DIRECTION('ref_axis',(0.,-0.707106781186548,-0.707106781186547));
#56132=DIRECTION('',(0.,1.,0.));
#56133=DIRECTION('center_axis',(1.,0.,0.));
#56134=DIRECTION('ref_axis',(0.,0.,-1.));
#56135=DIRECTION('',(0.,-0.965925826289068,0.258819045102522));
#56136=DIRECTION('center_axis',(-1.,0.,0.));
#56137=DIRECTION('ref_axis',(0.,-0.499999999999996,0.866025403784441));
#56138=DIRECTION('',(0.,-0.258819045102522,-0.965925826289068));
#56139=DIRECTION('center_axis',(-1.,0.,0.));
#56140=DIRECTION('ref_axis',(0.,-0.866025403784437,-0.500000000000003));
#56141=DIRECTION('',(0.,0.965925826289068,-0.258819045102522));
#56142=DIRECTION('center_axis',(1.,0.,0.));
#56143=DIRECTION('ref_axis',(0.,0.,-1.));
#56144=DIRECTION('',(0.,-0.866025403784438,0.5));
#56145=DIRECTION('center_axis',(-1.,0.,0.));
#56146=DIRECTION('ref_axis',(0.,-0.258819045102516,0.965925826289069));
#56147=DIRECTION('',(0.,-0.5,-0.866025403784438));
#56148=DIRECTION('center_axis',(-1.,0.,0.));
#56149=DIRECTION('ref_axis',(0.,-0.965925826289069,-0.25881904510252));
#56150=DIRECTION('',(0.,0.866025403784438,-0.5));
#56151=DIRECTION('center_axis',(1.,0.,0.));
#56152=DIRECTION('ref_axis',(0.,0.,-1.));
#56153=DIRECTION('',(0.,-0.707106781186547,0.707106781186548));
#56154=DIRECTION('center_axis',(-1.,0.,0.));
#56155=DIRECTION('ref_axis',(0.,0.,1.));
#56156=DIRECTION('',(0.,-0.707106781186548,-0.707106781186547));
#56157=DIRECTION('center_axis',(-1.,0.,0.));
#56158=DIRECTION('ref_axis',(0.,-1.,0.));
#56159=DIRECTION('',(0.,0.707106781186547,-0.707106781186548));
#56160=DIRECTION('center_axis',(1.,0.,0.));
#56161=DIRECTION('ref_axis',(0.,0.,-1.));
#56162=DIRECTION('',(0.,-0.499999999999999,0.866025403784439));
#56163=DIRECTION('center_axis',(-1.,0.,0.));
#56164=DIRECTION('ref_axis',(0.,0.258819045102522,0.965925826289068));
#56165=DIRECTION('',(0.,-0.866025403784439,-0.499999999999999));
#56166=DIRECTION('center_axis',(-1.,0.,0.));
#56167=DIRECTION('ref_axis',(0.,-0.965925826289068,0.258819045102523));
#56168=DIRECTION('',(0.,0.499999999999999,-0.866025403784439));
#56169=DIRECTION('center_axis',(1.,0.,0.));
#56170=DIRECTION('ref_axis',(0.,0.,-1.));
#56171=DIRECTION('',(0.,-0.25881904510252,0.965925826289068));
#56172=DIRECTION('center_axis',(-1.,0.,0.));
#56173=DIRECTION('ref_axis',(0.,0.499999999999998,0.86602540378444));
#56174=DIRECTION('',(0.,-0.965925826289068,-0.25881904510252));
#56175=DIRECTION('center_axis',(-1.,0.,0.));
#56176=DIRECTION('ref_axis',(0.,-0.866025403784438,0.500000000000001));
#56177=DIRECTION('',(0.,0.25881904510252,-0.965925826289068));
#56178=DIRECTION('center_axis',(1.,0.,0.));
#56179=DIRECTION('ref_axis',(0.,0.,-1.));
#56180=DIRECTION('',(0.,1.83697019872103E-16,1.));
#56181=DIRECTION('center_axis',(-1.,0.,0.));
#56182=DIRECTION('ref_axis',(0.,0.707106781186547,0.707106781186548));
#56183=DIRECTION('',(0.,-1.,1.83697019872103E-16));
#56184=DIRECTION('center_axis',(-1.,0.,0.));
#56185=DIRECTION('ref_axis',(0.,-0.707106781186547,0.707106781186548));
#56186=DIRECTION('',(0.,-1.83697019872103E-16,-1.));
#56187=DIRECTION('center_axis',(1.,0.,0.));
#56188=DIRECTION('ref_axis',(0.,0.,-1.));
#56189=DIRECTION('',(0.,0.258819045102522,0.965925826289068));
#56190=DIRECTION('center_axis',(-1.,0.,0.));
#56191=DIRECTION('ref_axis',(0.,0.866025403784441,0.499999999999996));
#56192=DIRECTION('',(0.,-0.965925826289068,0.258819045102522));
#56193=DIRECTION('center_axis',(-1.,0.,0.));
#56194=DIRECTION('ref_axis',(0.,-0.500000000000004,0.866025403784436));
#56195=DIRECTION('',(0.,-0.258819045102522,-0.965925826289068));
#56196=DIRECTION('center_axis',(1.,0.,0.));
#56197=DIRECTION('ref_axis',(0.,0.,-1.));
#56198=DIRECTION('',(0.,0.5,0.866025403784438));
#56199=DIRECTION('center_axis',(-1.,0.,0.));
#56200=DIRECTION('ref_axis',(0.,0.965925826289069,0.258819045102516));
#56201=DIRECTION('',(0.,-0.866025403784438,0.5));
#56202=DIRECTION('center_axis',(-1.,0.,0.));
#56203=DIRECTION('ref_axis',(0.,-0.25881904510252,0.965925826289069));
#56204=DIRECTION('',(0.,-0.5,-0.866025403784438));
#56205=DIRECTION('center_axis',(1.,0.,0.));
#56206=DIRECTION('ref_axis',(0.,0.,-1.));
#56207=DIRECTION('',(0.,0.707106781186548,0.707106781186547));
#56208=DIRECTION('center_axis',(-1.,0.,0.));
#56209=DIRECTION('ref_axis',(0.,1.,0.));
#56210=DIRECTION('',(0.,-0.707106781186547,0.707106781186548));
#56211=DIRECTION('center_axis',(-1.,0.,0.));
#56212=DIRECTION('ref_axis',(0.,0.,1.));
#56213=DIRECTION('',(0.,-0.707106781186548,-0.707106781186547));
#56214=DIRECTION('center_axis',(1.,0.,0.));
#56215=DIRECTION('ref_axis',(0.,0.,-1.));
#56216=DIRECTION('',(0.,0.866025403784439,0.5));
#56217=DIRECTION('center_axis',(-1.,0.,0.));
#56218=DIRECTION('ref_axis',(0.,0.965925826289069,-0.25881904510252));
#56219=DIRECTION('',(0.,-0.5,0.866025403784439));
#56220=DIRECTION('center_axis',(-1.,0.,0.));
#56221=DIRECTION('ref_axis',(0.,0.258819045102516,0.965925826289069));
#56222=DIRECTION('',(0.,-0.866025403784439,-0.5));
#56223=DIRECTION('center_axis',(1.,0.,0.));
#56224=DIRECTION('ref_axis',(0.,0.,-1.));
#56225=DIRECTION('',(0.,0.965925826289068,0.25881904510252));
#56226=DIRECTION('center_axis',(-1.,0.,0.));
#56227=DIRECTION('ref_axis',(0.,0.866025403784439,-0.499999999999999));
#56228=DIRECTION('',(0.,-0.25881904510252,0.965925826289068));
#56229=DIRECTION('center_axis',(-1.,0.,0.));
#56230=DIRECTION('ref_axis',(0.,0.500000000000002,0.866025403784438));
#56231=DIRECTION('',(0.,-0.965925826289068,-0.25881904510252));
#56232=DIRECTION('center_axis',(1.,0.,0.));
#56233=DIRECTION('ref_axis',(0.,0.,-1.));
#56234=DIRECTION('',(0.,1.,-1.22464679914735E-16));
#56235=DIRECTION('center_axis',(-1.,0.,0.));
#56236=DIRECTION('ref_axis',(0.,0.707106781186548,-0.707106781186547));
#56237=DIRECTION('',(0.,1.22464679914735E-16,1.));
#56238=DIRECTION('center_axis',(-1.,0.,0.));
#56239=DIRECTION('ref_axis',(0.,0.707106781186548,0.707106781186547));
#56240=DIRECTION('',(0.,-1.,1.22464679914735E-16));
#56241=DIRECTION('center_axis',(1.,0.,0.));
#56242=DIRECTION('ref_axis',(0.,0.,-1.));
#56243=DIRECTION('',(0.,0.965925826289068,-0.258819045102521));
#56244=DIRECTION('center_axis',(-1.,0.,0.));
#56245=DIRECTION('ref_axis',(0.,0.500000000000002,-0.866025403784438));
#56246=DIRECTION('',(0.,0.258819045102521,0.965925826289068));
#56247=DIRECTION('center_axis',(-1.,0.,0.));
#56248=DIRECTION('ref_axis',(0.,0.866025403784439,0.499999999999999));
#56249=DIRECTION('',(0.,-0.965925826289068,0.258819045102521));
#56250=DIRECTION('center_axis',(1.,0.,0.));
#56251=DIRECTION('ref_axis',(0.,0.,-1.));
#56252=DIRECTION('',(0.,0.866025403784438,-0.5));
#56253=DIRECTION('center_axis',(-1.,0.,0.));
#56254=DIRECTION('ref_axis',(0.,0.258819045102523,-0.965925826289068));
#56255=DIRECTION('',(0.,0.5,0.866025403784438));
#56256=DIRECTION('center_axis',(-1.,0.,0.));
#56257=DIRECTION('ref_axis',(0.,0.965925826289069,0.258819045102519));
#56258=DIRECTION('',(0.,-0.866025403784438,0.5));
#56259=DIRECTION('center_axis',(1.,0.,0.));
#56260=DIRECTION('ref_axis',(0.,0.,-1.));
#56261=DIRECTION('',(0.,0.707106781186547,-0.707106781186548));
#56262=DIRECTION('center_axis',(-1.,0.,0.));
#56263=DIRECTION('ref_axis',(0.,0.,-1.));
#56264=DIRECTION('',(0.,0.707106781186548,0.707106781186547));
#56265=DIRECTION('center_axis',(-1.,0.,0.));
#56266=DIRECTION('ref_axis',(0.,1.,0.));
#56267=DIRECTION('',(0.,-0.707106781186547,0.707106781186548));
#56268=DIRECTION('center_axis',(1.,0.,0.));
#56269=DIRECTION('ref_axis',(0.,0.,-1.));
#56270=DIRECTION('',(0.,0.5,-0.866025403784439));
#56271=DIRECTION('center_axis',(-1.,0.,0.));
#56272=DIRECTION('ref_axis',(0.,-0.25881904510252,-0.965925826289069));
#56273=DIRECTION('',(0.,0.866025403784439,0.5));
#56274=DIRECTION('center_axis',(-1.,0.,0.));
#56275=DIRECTION('ref_axis',(0.,0.965925826289068,-0.258819045102523));
#56276=DIRECTION('',(0.,-0.5,0.866025403784439));
#56277=DIRECTION('center_axis',(1.,0.,0.));
#56278=DIRECTION('ref_axis',(0.,0.,-1.));
#56279=DIRECTION('',(0.,0.258819045102521,-0.965925826289068));
#56280=DIRECTION('center_axis',(-1.,0.,0.));
#56281=DIRECTION('ref_axis',(0.,-0.500000000000001,-0.866025403784438));
#56282=DIRECTION('',(0.,0.965925826289068,0.258819045102521));
#56283=DIRECTION('center_axis',(-1.,0.,0.));
#56284=DIRECTION('ref_axis',(0.,0.866025403784438,-0.500000000000002));
#56285=DIRECTION('',(0.,-0.258819045102521,0.965925826289068));
#56286=DIRECTION('center_axis',(1.,0.,0.));
#56287=DIRECTION('ref_axis',(0.,0.,-1.));
#56288=DIRECTION('',(0.,-6.12323399573677E-17,-1.));
#56289=DIRECTION('center_axis',(-1.,0.,0.));
#56290=DIRECTION('ref_axis',(0.,-0.707106781186547,-0.707106781186548));
#56291=DIRECTION('',(0.,1.,-6.12323399573677E-17));
#56292=DIRECTION('center_axis',(-1.,0.,0.));
#56293=DIRECTION('ref_axis',(0.,0.707106781186547,-0.707106781186548));
#56294=DIRECTION('',(0.,6.12323399573677E-17,1.));
#56295=DIRECTION('center_axis',(1.,0.,0.));
#56296=DIRECTION('ref_axis',(0.,0.,-1.));
#56297=DIRECTION('',(0.,-0.258819045102521,-0.965925826289068));
#56298=DIRECTION('center_axis',(-1.,0.,0.));
#56299=DIRECTION('ref_axis',(0.,-0.866025403784438,-0.500000000000002));
#56300=DIRECTION('',(0.,0.965925826289068,-0.258819045102521));
#56301=DIRECTION('center_axis',(-1.,0.,0.));
#56302=DIRECTION('ref_axis',(0.,0.499999999999999,-0.866025403784439));
#56303=DIRECTION('',(0.,0.258819045102521,0.965925826289068));
#56304=DIRECTION('center_axis',(1.,0.,0.));
#56305=DIRECTION('ref_axis',(0.,0.,-1.));
#56306=DIRECTION('',(0.,-0.5,-0.866025403784439));
#56307=DIRECTION('center_axis',(-1.,0.,0.));
#56308=DIRECTION('ref_axis',(0.,-0.965925826289068,-0.258819045102523));
#56309=DIRECTION('',(0.,0.866025403784439,-0.5));
#56310=DIRECTION('center_axis',(-1.,0.,0.));
#56311=DIRECTION('ref_axis',(0.,0.25881904510252,-0.965925826289069));
#56312=DIRECTION('',(0.,0.5,0.866025403784439));
#56313=DIRECTION('center_axis',(1.,0.,0.));
#56314=DIRECTION('ref_axis',(0.,0.,-1.));
#56315=DIRECTION('',(0.,-0.707106781186548,-0.707106781186548));
#56316=DIRECTION('center_axis',(-1.,0.,0.));
#56317=DIRECTION('ref_axis',(0.,-1.,0.));
#56318=DIRECTION('',(0.,0.707106781186548,-0.707106781186548));
#56319=DIRECTION('center_axis',(-1.,0.,0.));
#56320=DIRECTION('ref_axis',(0.,0.,-1.));
#56321=DIRECTION('',(0.,0.707106781186548,0.707106781186548));
#56322=DIRECTION('center_axis',(1.,0.,0.));
#56323=DIRECTION('ref_axis',(0.,0.,-1.));
#56324=DIRECTION('',(0.,-0.866025403784439,-0.5));
#56325=DIRECTION('center_axis',(-1.,0.,0.));
#56326=DIRECTION('ref_axis',(0.,-0.965925826289069,0.258819045102519));
#56327=DIRECTION('',(0.,0.5,-0.866025403784439));
#56328=DIRECTION('center_axis',(-1.,0.,0.));
#56329=DIRECTION('ref_axis',(0.,-0.258819045102523,-0.965925826289068));
#56330=DIRECTION('',(0.,0.866025403784439,0.5));
#56331=DIRECTION('center_axis',(1.,0.,0.));
#56332=DIRECTION('ref_axis',(0.,0.,-1.));
#56333=DIRECTION('',(0.,-0.965925826289068,-0.258819045102521));
#56334=DIRECTION('center_axis',(-1.,0.,0.));
#56335=DIRECTION('ref_axis',(0.,-0.866025403784438,0.500000000000001));
#56336=DIRECTION('',(0.,0.258819045102521,-0.965925826289068));
#56337=DIRECTION('center_axis',(-1.,0.,0.));
#56338=DIRECTION('ref_axis',(0.,-0.500000000000001,-0.866025403784438));
#56339=DIRECTION('',(0.,0.965925826289068,0.258819045102521));
#56340=DIRECTION('center_axis',(1.,0.,0.));
#56341=DIRECTION('ref_axis',(0.,0.,-1.));
#56342=DIRECTION('center_axis',(1.,0.,0.));
#56343=DIRECTION('ref_axis',(0.,-0.707106781186548,-0.707106781186547));
#56344=DIRECTION('',(-1.,0.,0.));
#56345=DIRECTION('center_axis',(1.,0.,0.));
#56346=DIRECTION('ref_axis',(0.,-0.707106781186548,-0.707106781186547));
#56347=DIRECTION('',(1.,0.,0.));
#56348=DIRECTION('center_axis',(0.,0.,-1.));
#56349=DIRECTION('ref_axis',(0.,1.,0.));
#56350=DIRECTION('',(0.,1.,0.));
#56351=DIRECTION('',(-1.,0.,0.));
#56352=DIRECTION('center_axis',(-1.,0.,0.));
#56353=DIRECTION('ref_axis',(0.,0.,1.));
#56354=DIRECTION('center_axis',(1.,0.,0.));
#56355=DIRECTION('ref_axis',(0.,-1.,-1.06397713344143E-13));
#56356=DIRECTION('center_axis',(1.,0.,0.));
#56357=DIRECTION('ref_axis',(0.,0.499999999999946,0.86602540378447));
#56358=DIRECTION('center_axis',(1.,0.,0.));
#56359=DIRECTION('ref_axis',(0.,0.500000000000038,-0.866025403784417));
#56360=DIRECTION('center_axis',(1.,0.,0.));
#56361=DIRECTION('ref_axis',(0.,0.,-1.));
#56362=DIRECTION('',(0.,0.965925826289068,0.258819045102521));
#56363=DIRECTION('center_axis',(1.,0.,0.));
#56364=DIRECTION('ref_axis',(0.,-0.500000000000001,-0.866025403784438));
#56365=DIRECTION('',(0.,0.258819045102521,-0.965925826289068));
#56366=DIRECTION('center_axis',(1.,0.,0.));
#56367=DIRECTION('ref_axis',(0.,-0.866025403784438,0.500000000000001));
#56368=DIRECTION('',(0.,-0.965925826289068,-0.258819045102521));
#56369=DIRECTION('center_axis',(1.,0.,0.));
#56370=DIRECTION('ref_axis',(0.,0.,-1.));
#56371=DIRECTION('',(0.,0.866025403784439,0.5));
#56372=DIRECTION('center_axis',(1.,0.,0.));
#56373=DIRECTION('ref_axis',(0.,-0.258819045102523,-0.965925826289068));
#56374=DIRECTION('',(0.,0.5,-0.866025403784439));
#56375=DIRECTION('center_axis',(1.,0.,0.));
#56376=DIRECTION('ref_axis',(0.,-0.965925826289069,0.258819045102519));
#56377=DIRECTION('',(0.,-0.866025403784439,-0.5));
#56378=DIRECTION('center_axis',(1.,0.,0.));
#56379=DIRECTION('ref_axis',(0.,0.,-1.));
#56380=DIRECTION('',(0.,0.707106781186548,0.707106781186548));
#56381=DIRECTION('center_axis',(1.,0.,0.));
#56382=DIRECTION('ref_axis',(0.,0.,-1.));
#56383=DIRECTION('',(0.,0.707106781186548,-0.707106781186548));
#56384=DIRECTION('center_axis',(1.,0.,0.));
#56385=DIRECTION('ref_axis',(0.,-1.,0.));
#56386=DIRECTION('',(0.,-0.707106781186548,-0.707106781186548));
#56387=DIRECTION('center_axis',(1.,0.,0.));
#56388=DIRECTION('ref_axis',(0.,0.,-1.));
#56389=DIRECTION('',(0.,0.5,0.866025403784439));
#56390=DIRECTION('center_axis',(1.,0.,0.));
#56391=DIRECTION('ref_axis',(0.,0.25881904510252,-0.965925826289069));
#56392=DIRECTION('',(0.,0.866025403784439,-0.5));
#56393=DIRECTION('center_axis',(1.,0.,0.));
#56394=DIRECTION('ref_axis',(0.,-0.965925826289068,-0.258819045102523));
#56395=DIRECTION('',(0.,-0.5,-0.866025403784439));
#56396=DIRECTION('center_axis',(1.,0.,0.));
#56397=DIRECTION('ref_axis',(0.,0.,-1.));
#56398=DIRECTION('',(0.,0.258819045102521,0.965925826289068));
#56399=DIRECTION('center_axis',(1.,0.,0.));
#56400=DIRECTION('ref_axis',(0.,0.499999999999999,-0.866025403784439));
#56401=DIRECTION('',(0.,0.965925826289068,-0.258819045102521));
#56402=DIRECTION('center_axis',(1.,0.,0.));
#56403=DIRECTION('ref_axis',(0.,-0.866025403784438,-0.500000000000002));
#56404=DIRECTION('',(0.,-0.258819045102521,-0.965925826289068));
#56405=DIRECTION('center_axis',(1.,0.,0.));
#56406=DIRECTION('ref_axis',(0.,0.,-1.));
#56407=DIRECTION('',(0.,6.12323399573677E-17,1.));
#56408=DIRECTION('center_axis',(1.,0.,0.));
#56409=DIRECTION('ref_axis',(0.,0.707106781186547,-0.707106781186548));
#56410=DIRECTION('',(0.,1.,-6.12323399573677E-17));
#56411=DIRECTION('center_axis',(1.,0.,0.));
#56412=DIRECTION('ref_axis',(0.,-0.707106781186547,-0.707106781186548));
#56413=DIRECTION('',(0.,-6.12323399573677E-17,-1.));
#56414=DIRECTION('center_axis',(1.,0.,0.));
#56415=DIRECTION('ref_axis',(0.,0.,-1.));
#56416=DIRECTION('',(0.,-0.258819045102521,0.965925826289068));
#56417=DIRECTION('center_axis',(1.,0.,0.));
#56418=DIRECTION('ref_axis',(0.,0.866025403784438,-0.500000000000002));
#56419=DIRECTION('',(0.,0.965925826289068,0.258819045102521));
#56420=DIRECTION('center_axis',(1.,0.,0.));
#56421=DIRECTION('ref_axis',(0.,-0.500000000000001,-0.866025403784438));
#56422=DIRECTION('',(0.,0.258819045102521,-0.965925826289068));
#56423=DIRECTION('center_axis',(1.,0.,0.));
#56424=DIRECTION('ref_axis',(0.,0.,-1.));
#56425=DIRECTION('',(0.,-0.5,0.866025403784439));
#56426=DIRECTION('center_axis',(1.,0.,0.));
#56427=DIRECTION('ref_axis',(0.,0.965925826289068,-0.258819045102523));
#56428=DIRECTION('',(0.,0.866025403784439,0.5));
#56429=DIRECTION('center_axis',(1.,0.,0.));
#56430=DIRECTION('ref_axis',(0.,-0.25881904510252,-0.965925826289069));
#56431=DIRECTION('',(0.,0.5,-0.866025403784439));
#56432=DIRECTION('center_axis',(1.,0.,0.));
#56433=DIRECTION('ref_axis',(0.,0.,-1.));
#56434=DIRECTION('',(0.,-0.707106781186547,0.707106781186548));
#56435=DIRECTION('center_axis',(1.,0.,0.));
#56436=DIRECTION('ref_axis',(0.,1.,0.));
#56437=DIRECTION('',(0.,0.707106781186548,0.707106781186547));
#56438=DIRECTION('center_axis',(1.,0.,0.));
#56439=DIRECTION('ref_axis',(0.,0.,-1.));
#56440=DIRECTION('',(0.,0.707106781186547,-0.707106781186548));
#56441=DIRECTION('center_axis',(1.,0.,0.));
#56442=DIRECTION('ref_axis',(0.,0.,-1.));
#56443=DIRECTION('',(0.,-0.866025403784438,0.5));
#56444=DIRECTION('center_axis',(1.,0.,0.));
#56445=DIRECTION('ref_axis',(0.,0.965925826289069,0.258819045102519));
#56446=DIRECTION('',(0.,0.5,0.866025403784438));
#56447=DIRECTION('center_axis',(1.,0.,0.));
#56448=DIRECTION('ref_axis',(0.,0.258819045102523,-0.965925826289068));
#56449=DIRECTION('',(0.,0.866025403784438,-0.5));
#56450=DIRECTION('center_axis',(1.,0.,0.));
#56451=DIRECTION('ref_axis',(0.,0.,-1.));
#56452=DIRECTION('',(0.,-0.965925826289068,0.258819045102521));
#56453=DIRECTION('center_axis',(1.,0.,0.));
#56454=DIRECTION('ref_axis',(0.,0.866025403784439,0.499999999999999));
#56455=DIRECTION('',(0.,0.258819045102521,0.965925826289068));
#56456=DIRECTION('center_axis',(1.,0.,0.));
#56457=DIRECTION('ref_axis',(0.,0.500000000000002,-0.866025403784438));
#56458=DIRECTION('',(0.,0.965925826289068,-0.258819045102521));
#56459=DIRECTION('center_axis',(1.,0.,0.));
#56460=DIRECTION('ref_axis',(0.,0.,-1.));
#56461=DIRECTION('',(0.,-1.,1.22464679914735E-16));
#56462=DIRECTION('center_axis',(1.,0.,0.));
#56463=DIRECTION('ref_axis',(0.,0.707106781186548,0.707106781186547));
#56464=DIRECTION('',(0.,1.22464679914735E-16,1.));
#56465=DIRECTION('center_axis',(1.,0.,0.));
#56466=DIRECTION('ref_axis',(0.,0.707106781186548,-0.707106781186547));
#56467=DIRECTION('',(0.,1.,-1.22464679914735E-16));
#56468=DIRECTION('center_axis',(1.,0.,0.));
#56469=DIRECTION('ref_axis',(0.,0.,-1.));
#56470=DIRECTION('',(0.,-0.965925826289068,-0.25881904510252));
#56471=DIRECTION('center_axis',(1.,0.,0.));
#56472=DIRECTION('ref_axis',(0.,0.500000000000002,0.866025403784438));
#56473=DIRECTION('',(0.,-0.25881904510252,0.965925826289068));
#56474=DIRECTION('center_axis',(1.,0.,0.));
#56475=DIRECTION('ref_axis',(0.,0.866025403784439,-0.499999999999999));
#56476=DIRECTION('',(0.,0.965925826289068,0.25881904510252));
#56477=DIRECTION('center_axis',(1.,0.,0.));
#56478=DIRECTION('ref_axis',(0.,0.,-1.));
#56479=DIRECTION('',(0.,-0.866025403784439,-0.5));
#56480=DIRECTION('center_axis',(1.,0.,0.));
#56481=DIRECTION('ref_axis',(0.,0.258819045102516,0.965925826289069));
#56482=DIRECTION('',(0.,-0.5,0.866025403784439));
#56483=DIRECTION('center_axis',(1.,0.,0.));
#56484=DIRECTION('ref_axis',(0.,0.965925826289069,-0.25881904510252));
#56485=DIRECTION('',(0.,0.866025403784439,0.5));
#56486=DIRECTION('center_axis',(1.,0.,0.));
#56487=DIRECTION('ref_axis',(0.,0.,-1.));
#56488=DIRECTION('',(0.,-0.707106781186548,-0.707106781186547));
#56489=DIRECTION('center_axis',(1.,0.,0.));
#56490=DIRECTION('ref_axis',(0.,0.,1.));
#56491=DIRECTION('',(0.,-0.707106781186547,0.707106781186548));
#56492=DIRECTION('center_axis',(1.,0.,0.));
#56493=DIRECTION('ref_axis',(0.,1.,0.));
#56494=DIRECTION('',(0.,0.707106781186548,0.707106781186547));
#56495=DIRECTION('center_axis',(1.,0.,0.));
#56496=DIRECTION('ref_axis',(0.,0.,-1.));
#56497=DIRECTION('',(0.,-0.5,-0.866025403784438));
#56498=DIRECTION('center_axis',(1.,0.,0.));
#56499=DIRECTION('ref_axis',(0.,-0.25881904510252,0.965925826289069));
#56500=DIRECTION('',(0.,-0.866025403784438,0.5));
#56501=DIRECTION('center_axis',(1.,0.,0.));
#56502=DIRECTION('ref_axis',(0.,0.965925826289069,0.258819045102516));
#56503=DIRECTION('',(0.,0.5,0.866025403784438));
#56504=DIRECTION('center_axis',(1.,0.,0.));
#56505=DIRECTION('ref_axis',(0.,0.,-1.));
#56506=DIRECTION('',(0.,-0.258819045102522,-0.965925826289068));
#56507=DIRECTION('center_axis',(1.,0.,0.));
#56508=DIRECTION('ref_axis',(0.,-0.500000000000004,0.866025403784436));
#56509=DIRECTION('',(0.,-0.965925826289068,0.258819045102522));
#56510=DIRECTION('center_axis',(1.,0.,0.));
#56511=DIRECTION('ref_axis',(0.,0.866025403784441,0.499999999999996));
#56512=DIRECTION('',(0.,0.258819045102522,0.965925826289068));
#56513=DIRECTION('center_axis',(1.,0.,0.));
#56514=DIRECTION('ref_axis',(0.,0.,-1.));
#56515=DIRECTION('',(0.,-1.83697019872103E-16,-1.));
#56516=DIRECTION('center_axis',(1.,0.,0.));
#56517=DIRECTION('ref_axis',(0.,-0.707106781186547,0.707106781186548));
#56518=DIRECTION('',(0.,-1.,1.83697019872103E-16));
#56519=DIRECTION('center_axis',(1.,0.,0.));
#56520=DIRECTION('ref_axis',(0.,0.707106781186547,0.707106781186548));
#56521=DIRECTION('',(0.,1.83697019872103E-16,1.));
#56522=DIRECTION('center_axis',(1.,0.,0.));
#56523=DIRECTION('ref_axis',(0.,0.,-1.));
#56524=DIRECTION('',(0.,0.25881904510252,-0.965925826289068));
#56525=DIRECTION('center_axis',(1.,0.,0.));
#56526=DIRECTION('ref_axis',(0.,-0.866025403784438,0.500000000000001));
#56527=DIRECTION('',(0.,-0.965925826289068,-0.25881904510252));
#56528=DIRECTION('center_axis',(1.,0.,0.));
#56529=DIRECTION('ref_axis',(0.,0.499999999999998,0.86602540378444));
#56530=DIRECTION('',(0.,-0.25881904510252,0.965925826289068));
#56531=DIRECTION('center_axis',(1.,0.,0.));
#56532=DIRECTION('ref_axis',(0.,0.,-1.));
#56533=DIRECTION('',(0.,0.499999999999999,-0.866025403784439));
#56534=DIRECTION('center_axis',(1.,0.,0.));
#56535=DIRECTION('ref_axis',(0.,-0.965925826289068,0.258819045102523));
#56536=DIRECTION('',(0.,-0.866025403784439,-0.499999999999999));
#56537=DIRECTION('center_axis',(1.,0.,0.));
#56538=DIRECTION('ref_axis',(0.,0.258819045102522,0.965925826289068));
#56539=DIRECTION('',(0.,-0.499999999999999,0.866025403784439));
#56540=DIRECTION('center_axis',(1.,0.,0.));
#56541=DIRECTION('ref_axis',(0.,0.,-1.));
#56542=DIRECTION('',(0.,0.707106781186547,-0.707106781186548));
#56543=DIRECTION('center_axis',(1.,0.,0.));
#56544=DIRECTION('ref_axis',(0.,-1.,0.));
#56545=DIRECTION('',(0.,-0.707106781186548,-0.707106781186547));
#56546=DIRECTION('center_axis',(1.,0.,0.));
#56547=DIRECTION('ref_axis',(0.,0.,1.));
#56548=DIRECTION('',(0.,-0.707106781186547,0.707106781186548));
#56549=DIRECTION('center_axis',(1.,0.,0.));
#56550=DIRECTION('ref_axis',(0.,0.,-1.));
#56551=DIRECTION('',(0.,0.866025403784438,-0.5));
#56552=DIRECTION('center_axis',(1.,0.,0.));
#56553=DIRECTION('ref_axis',(0.,-0.965925826289069,-0.25881904510252));
#56554=DIRECTION('',(0.,-0.5,-0.866025403784438));
#56555=DIRECTION('center_axis',(1.,0.,0.));
#56556=DIRECTION('ref_axis',(0.,-0.258819045102516,0.965925826289069));
#56557=DIRECTION('',(0.,-0.866025403784438,0.5));
#56558=DIRECTION('center_axis',(1.,0.,0.));
#56559=DIRECTION('ref_axis',(0.,0.,-1.));
#56560=DIRECTION('',(0.,0.965925826289068,-0.258819045102522));
#56561=DIRECTION('center_axis',(1.,0.,0.));
#56562=DIRECTION('ref_axis',(0.,-0.866025403784437,-0.500000000000003));
#56563=DIRECTION('',(0.,-0.258819045102522,-0.965925826289068));
#56564=DIRECTION('center_axis',(1.,0.,0.));
#56565=DIRECTION('ref_axis',(0.,-0.499999999999996,0.866025403784441));
#56566=DIRECTION('',(0.,-0.965925826289068,0.258819045102522));
#56567=DIRECTION('center_axis',(1.,0.,0.));
#56568=DIRECTION('ref_axis',(0.,0.,-1.));
#56569=DIRECTION('',(0.,0.,-1.));
#56570=DIRECTION('center_axis',(1.,0.,0.));
#56571=DIRECTION('ref_axis',(0.,-0.866025403784438,0.500000000000001));
#56572=DIRECTION('',(-1.,0.,0.));
#56573=DIRECTION('',(1.,0.,0.));
#56574=DIRECTION('center_axis',(0.,-0.965925826289068,-0.258819045102521));
#56575=DIRECTION('ref_axis',(0.,0.258819045102521,-0.965925826289068));
#56576=DIRECTION('',(-1.,0.,0.));
#56577=DIRECTION('center_axis',(1.,0.,0.));
#56578=DIRECTION('ref_axis',(0.,-0.500000000000001,-0.866025403784438));
#56579=DIRECTION('',(1.,0.,0.));
#56580=DIRECTION('center_axis',(1.,0.,0.));
#56581=DIRECTION('ref_axis',(0.,-0.258819045102523,-0.965925826289068));
#56582=DIRECTION('',(-1.,0.,0.));
#56583=DIRECTION('',(1.,0.,0.));
#56584=DIRECTION('center_axis',(0.,0.5,-0.866025403784439));
#56585=DIRECTION('ref_axis',(0.,0.866025403784439,0.5));
#56586=DIRECTION('',(-1.,0.,0.));
#56587=DIRECTION('center_axis',(1.,0.,0.));
#56588=DIRECTION('ref_axis',(0.,-0.965925826289069,0.258819045102519));
#56589=DIRECTION('',(-1.,0.,0.));
#56590=DIRECTION('',(1.,0.,0.));
#56591=DIRECTION('center_axis',(0.,-0.5,0.866025403784439));
#56592=DIRECTION('ref_axis',(0.,-0.866025403784439,-0.5));
#56593=DIRECTION('',(1.,0.,0.));
#56594=DIRECTION('center_axis',(1.,0.,0.));
#56595=DIRECTION('ref_axis',(0.,0.,-1.));
#56596=DIRECTION('',(-1.,0.,0.));
#56597=DIRECTION('',(1.,0.,0.));
#56598=DIRECTION('center_axis',(0.,-0.707106781186548,-0.707106781186548));
#56599=DIRECTION('ref_axis',(0.,0.707106781186548,-0.707106781186548));
#56600=DIRECTION('',(1.,0.,0.));
#56601=DIRECTION('center_axis',(1.,0.,0.));
#56602=DIRECTION('ref_axis',(0.,-1.,0.));
#56603=DIRECTION('',(-1.,0.,0.));
#56604=DIRECTION('center_axis',(1.,0.,0.));
#56605=DIRECTION('ref_axis',(0.,-0.965925826289068,-0.258819045102523));
#56606=DIRECTION('',(-1.,0.,0.));
#56607=DIRECTION('',(1.,0.,0.));
#56608=DIRECTION('center_axis',(0.,-0.5,-0.866025403784439));
#56609=DIRECTION('ref_axis',(0.,0.866025403784439,-0.5));
#56610=DIRECTION('',(-1.,0.,0.));
#56611=DIRECTION('center_axis',(1.,0.,0.));
#56612=DIRECTION('ref_axis',(0.,0.25881904510252,-0.965925826289069));
#56613=DIRECTION('',(1.,0.,0.));
#56614=DIRECTION('center_axis',(1.,0.,0.));
#56615=DIRECTION('ref_axis',(0.,0.499999999999999,-0.866025403784439));
#56616=DIRECTION('',(-1.,0.,0.));
#56617=DIRECTION('',(1.,0.,0.));
#56618=DIRECTION('center_axis',(0.,0.965925826289068,-0.258819045102521));
#56619=DIRECTION('ref_axis',(0.,0.258819045102521,0.965925826289068));
#56620=DIRECTION('',(-1.,0.,0.));
#56621=DIRECTION('center_axis',(1.,0.,0.));
#56622=DIRECTION('ref_axis',(0.,-0.866025403784438,-0.500000000000002));
#56623=DIRECTION('',(-1.,0.,0.));
#56624=DIRECTION('',(1.,0.,0.));
#56625=DIRECTION('center_axis',(0.,-0.965925826289068,0.258819045102521));
#56626=DIRECTION('ref_axis',(0.,-0.258819045102521,-0.965925826289068));
#56627=DIRECTION('',(1.,0.,0.));
#56628=DIRECTION('center_axis',(1.,0.,0.));
#56629=DIRECTION('ref_axis',(0.,0.707106781186547,-0.707106781186548));
#56630=DIRECTION('',(-1.,0.,0.));
#56631=DIRECTION('',(1.,0.,0.));
#56632=DIRECTION('center_axis',(0.,-6.12323399573677E-17,-1.));
#56633=DIRECTION('ref_axis',(0.,1.,-6.12323399573677E-17));
#56634=DIRECTION('',(1.,0.,0.));
#56635=DIRECTION('center_axis',(1.,0.,0.));
#56636=DIRECTION('ref_axis',(0.,-0.707106781186547,-0.707106781186548));
#56637=DIRECTION('',(-1.,0.,0.));
#56638=DIRECTION('center_axis',(1.,0.,0.));
#56639=DIRECTION('ref_axis',(0.,-0.500000000000001,-0.866025403784438));
#56640=DIRECTION('',(-1.,0.,0.));
#56641=DIRECTION('',(1.,0.,0.));
#56642=DIRECTION('center_axis',(0.,0.258819045102521,-0.965925826289068));
#56643=DIRECTION('ref_axis',(0.,0.965925826289068,0.258819045102521));
#56644=DIRECTION('',(-1.,0.,0.));
#56645=DIRECTION('center_axis',(1.,0.,0.));
#56646=DIRECTION('ref_axis',(0.,0.866025403784438,-0.500000000000002));
#56647=DIRECTION('',(1.,0.,0.));
#56648=DIRECTION('center_axis',(1.,0.,0.));
#56649=DIRECTION('ref_axis',(0.,0.965925826289068,-0.258819045102523));
#56650=DIRECTION('',(-1.,0.,0.));
#56651=DIRECTION('',(1.,0.,0.));
#56652=DIRECTION('center_axis',(0.,0.866025403784439,0.5));
#56653=DIRECTION('ref_axis',(0.,-0.5,0.866025403784439));
#56654=DIRECTION('',(-1.,0.,0.));
#56655=DIRECTION('center_axis',(1.,0.,0.));
#56656=DIRECTION('ref_axis',(0.,-0.25881904510252,-0.965925826289069));
#56657=DIRECTION('',(-1.,0.,0.));
#56658=DIRECTION('',(1.,0.,0.));
#56659=DIRECTION('center_axis',(0.,-0.866025403784439,-0.5));
#56660=DIRECTION('ref_axis',(0.,0.5,-0.866025403784439));
#56661=DIRECTION('',(1.,0.,0.));
#56662=DIRECTION('center_axis',(1.,0.,0.));
#56663=DIRECTION('ref_axis',(0.,1.,0.));
#56664=DIRECTION('',(-1.,0.,0.));
#56665=DIRECTION('',(1.,0.,0.));
#56666=DIRECTION('center_axis',(0.,0.707106781186547,-0.707106781186548));
#56667=DIRECTION('ref_axis',(0.,0.707106781186548,0.707106781186547));
#56668=DIRECTION('',(1.,0.,0.));
#56669=DIRECTION('center_axis',(1.,0.,0.));
#56670=DIRECTION('ref_axis',(0.,0.,-1.));
#56671=DIRECTION('',(-1.,0.,0.));
#56672=DIRECTION('center_axis',(1.,0.,0.));
#56673=DIRECTION('ref_axis',(0.,0.258819045102523,-0.965925826289068));
#56674=DIRECTION('',(-1.,0.,0.));
#56675=DIRECTION('',(1.,0.,0.));
#56676=DIRECTION('center_axis',(0.,0.866025403784438,-0.5));
#56677=DIRECTION('ref_axis',(0.,0.5,0.866025403784438));
#56678=DIRECTION('',(-1.,0.,0.));
#56679=DIRECTION('center_axis',(1.,0.,0.));
#56680=DIRECTION('ref_axis',(0.,0.965925826289069,0.258819045102519));
#56681=DIRECTION('',(1.,0.,0.));
#56682=DIRECTION('center_axis',(1.,0.,0.));
#56683=DIRECTION('ref_axis',(0.,0.866025403784439,0.499999999999999));
#56684=DIRECTION('',(-1.,0.,0.));
#56685=DIRECTION('',(1.,0.,0.));
#56686=DIRECTION('center_axis',(0.,0.258819045102521,0.965925826289068));
#56687=DIRECTION('ref_axis',(0.,-0.965925826289068,0.258819045102521));
#56688=DIRECTION('',(-1.,0.,0.));
#56689=DIRECTION('center_axis',(1.,0.,0.));
#56690=DIRECTION('ref_axis',(0.,0.500000000000002,-0.866025403784438));
#56691=DIRECTION('',(-1.,0.,0.));
#56692=DIRECTION('',(1.,0.,0.));
#56693=DIRECTION('center_axis',(0.,-0.258819045102521,-0.965925826289068));
#56694=DIRECTION('ref_axis',(0.,0.965925826289068,-0.258819045102521));
#56695=DIRECTION('',(1.,0.,0.));
#56696=DIRECTION('center_axis',(1.,0.,0.));
#56697=DIRECTION('ref_axis',(0.,0.707106781186548,0.707106781186547));
#56698=DIRECTION('',(-1.,0.,0.));
#56699=DIRECTION('',(1.,0.,0.));
#56700=DIRECTION('center_axis',(0.,1.,-1.22464679914735E-16));
#56701=DIRECTION('ref_axis',(0.,1.22464679914735E-16,1.));
#56702=DIRECTION('',(1.,0.,0.));
#56703=DIRECTION('center_axis',(1.,0.,0.));
#56704=DIRECTION('ref_axis',(0.,0.707106781186548,-0.707106781186547));
#56705=DIRECTION('',(-1.,0.,0.));
#56706=DIRECTION('center_axis',(1.,0.,0.));
#56707=DIRECTION('ref_axis',(0.,0.866025403784439,-0.499999999999999));
#56708=DIRECTION('',(-1.,0.,0.));
#56709=DIRECTION('',(1.,0.,0.));
#56710=DIRECTION('center_axis',(0.,0.965925826289068,0.25881904510252));
#56711=DIRECTION('ref_axis',(0.,-0.25881904510252,0.965925826289068));
#56712=DIRECTION('',(-1.,0.,0.));
#56713=DIRECTION('center_axis',(1.,0.,0.));
#56714=DIRECTION('ref_axis',(0.,0.500000000000002,0.866025403784438));
#56715=DIRECTION('',(1.,0.,0.));
#56716=DIRECTION('center_axis',(1.,0.,0.));
#56717=DIRECTION('ref_axis',(0.,0.258819045102516,0.965925826289069));
#56718=DIRECTION('',(-1.,0.,0.));
#56719=DIRECTION('',(1.,0.,0.));
#56720=DIRECTION('center_axis',(0.,-0.5,0.866025403784439));
#56721=DIRECTION('ref_axis',(0.,-0.866025403784439,-0.5));
#56722=DIRECTION('',(-1.,0.,0.));
#56723=DIRECTION('center_axis',(1.,0.,0.));
#56724=DIRECTION('ref_axis',(0.,0.965925826289069,-0.25881904510252));
#56725=DIRECTION('',(-1.,0.,0.));
#56726=DIRECTION('',(1.,0.,0.));
#56727=DIRECTION('center_axis',(0.,0.5,-0.866025403784439));
#56728=DIRECTION('ref_axis',(0.,0.866025403784439,0.5));
#56729=DIRECTION('',(1.,0.,0.));
#56730=DIRECTION('center_axis',(1.,0.,0.));
#56731=DIRECTION('ref_axis',(0.,0.,1.));
#56732=DIRECTION('',(-1.,0.,0.));
#56733=DIRECTION('',(1.,0.,0.));
#56734=DIRECTION('center_axis',(0.,0.707106781186548,0.707106781186547));
#56735=DIRECTION('ref_axis',(0.,-0.707106781186547,0.707106781186548));
#56736=DIRECTION('',(1.,0.,0.));
#56737=DIRECTION('center_axis',(1.,0.,0.));
#56738=DIRECTION('ref_axis',(0.,1.,0.));
#56739=DIRECTION('',(-1.,0.,0.));
#56740=DIRECTION('center_axis',(1.,0.,0.));
#56741=DIRECTION('ref_axis',(0.,0.965925826289069,0.258819045102516));
#56742=DIRECTION('',(-1.,0.,0.));
#56743=DIRECTION('',(1.,0.,0.));
#56744=DIRECTION('center_axis',(0.,0.5,0.866025403784438));
#56745=DIRECTION('ref_axis',(0.,-0.866025403784438,0.5));
#56746=DIRECTION('',(-1.,0.,0.));
#56747=DIRECTION('center_axis',(1.,0.,0.));
#56748=DIRECTION('ref_axis',(0.,-0.25881904510252,0.965925826289069));
#56749=DIRECTION('',(1.,0.,0.));
#56750=DIRECTION('center_axis',(1.,0.,0.));
#56751=DIRECTION('ref_axis',(0.,0.,-1.));
#56752=DIRECTION('center_axis',(1.,0.,0.));
#56753=DIRECTION('ref_axis',(0.,0.499999999999999,-0.866025403784439));
#56754=DIRECTION('center_axis',(-1.,0.,0.));
#56755=DIRECTION('ref_axis',(0.,0.499999999999999,-0.866025403784439));
#56756=DIRECTION('center_axis',(1.,0.,0.));
#56757=DIRECTION('ref_axis',(0.,1.,0.));
#56758=DIRECTION('center_axis',(-1.,0.,0.));
#56759=DIRECTION('ref_axis',(0.,0.500000000000038,-0.866025403784417));
#56760=DIRECTION('center_axis',(1.,0.,0.));
#56761=DIRECTION('ref_axis',(0.,-0.500000000000004,0.866025403784436));
#56762=DIRECTION('',(-1.,0.,0.));
#56763=DIRECTION('',(1.,0.,0.));
#56764=DIRECTION('center_axis',(0.,-0.965925826289068,0.258819045102522));
#56765=DIRECTION('ref_axis',(0.,-0.258819045102522,-0.965925826289068));
#56766=DIRECTION('',(-1.,0.,0.));
#56767=DIRECTION('center_axis',(1.,0.,0.));
#56768=DIRECTION('ref_axis',(0.,0.866025403784441,0.499999999999996));
#56769=DIRECTION('',(-1.,0.,0.));
#56770=DIRECTION('',(1.,0.,0.));
#56771=DIRECTION('center_axis',(0.,0.965925826289068,-0.258819045102522));
#56772=DIRECTION('ref_axis',(0.,0.258819045102522,0.965925826289068));
#56773=DIRECTION('',(1.,0.,0.));
#56774=DIRECTION('center_axis',(1.,0.,0.));
#56775=DIRECTION('ref_axis',(0.,-0.707106781186547,0.707106781186548));
#56776=DIRECTION('',(-1.,0.,0.));
#56777=DIRECTION('',(1.,0.,0.));
#56778=DIRECTION('center_axis',(0.,1.83697019872103E-16,1.));
#56779=DIRECTION('ref_axis',(0.,-1.,1.83697019872103E-16));
#56780=DIRECTION('',(1.,0.,0.));
#56781=DIRECTION('center_axis',(1.,0.,0.));
#56782=DIRECTION('ref_axis',(0.,0.707106781186547,0.707106781186548));
#56783=DIRECTION('',(-1.,0.,0.));
#56784=DIRECTION('center_axis',(1.,0.,0.));
#56785=DIRECTION('ref_axis',(0.,0.499999999999998,0.86602540378444));
#56786=DIRECTION('',(-1.,0.,0.));
#56787=DIRECTION('',(1.,0.,0.));
#56788=DIRECTION('center_axis',(0.,-0.25881904510252,0.965925826289068));
#56789=DIRECTION('ref_axis',(0.,-0.965925826289068,-0.25881904510252));
#56790=DIRECTION('',(-1.,0.,0.));
#56791=DIRECTION('center_axis',(1.,0.,0.));
#56792=DIRECTION('ref_axis',(0.,-0.866025403784438,0.500000000000001));
#56793=DIRECTION('',(1.,0.,0.));
#56794=DIRECTION('center_axis',(1.,0.,0.));
#56795=DIRECTION('ref_axis',(0.,0.,-1.));
#56796=DIRECTION('center_axis',(1.,0.,0.));
#56797=DIRECTION('ref_axis',(0.,-1.,1.07187543957223E-15));
#56798=DIRECTION('center_axis',(-1.,0.,0.));
#56799=DIRECTION('ref_axis',(0.,-1.,9.18794589678809E-16));
#56800=DIRECTION('center_axis',(1.,0.,0.));
#56801=DIRECTION('ref_axis',(0.,-1.,1.22464679914735E-16));
#56802=DIRECTION('center_axis',(-1.,0.,0.));
#56803=DIRECTION('ref_axis',(0.,-1.,1.83697019872103E-16));
#56804=DIRECTION('center_axis',(1.,0.,0.));
#56805=DIRECTION('ref_axis',(0.,0.,-1.));
#56806=DIRECTION('center_axis',(1.,0.,0.));
#56807=DIRECTION('ref_axis',(0.,0.499999999999999,-0.866025403784439));
#56808=DIRECTION('center_axis',(-1.,0.,0.));
#56809=DIRECTION('ref_axis',(0.,0.499999999999999,-0.866025403784439));
#56810=DIRECTION('center_axis',(1.,0.,0.));
#56811=DIRECTION('ref_axis',(0.,1.,0.));
#56812=DIRECTION('center_axis',(1.,0.,0.));
#56813=DIRECTION('ref_axis',(0.,-0.965925826289068,0.258819045102523));
#56814=DIRECTION('',(-1.,0.,0.));
#56815=DIRECTION('',(1.,0.,0.));
#56816=DIRECTION('center_axis',(0.,-0.866025403784439,-0.499999999999999));
#56817=DIRECTION('ref_axis',(0.,0.499999999999999,-0.866025403784439));
#56818=DIRECTION('',(-1.,0.,0.));
#56819=DIRECTION('center_axis',(1.,0.,0.));
#56820=DIRECTION('ref_axis',(0.,0.258819045102522,0.965925826289068));
#56821=DIRECTION('',(-1.,0.,0.));
#56822=DIRECTION('',(1.,0.,0.));
#56823=DIRECTION('center_axis',(0.,0.866025403784439,0.499999999999999));
#56824=DIRECTION('ref_axis',(0.,-0.499999999999999,0.866025403784439));
#56825=DIRECTION('',(1.,0.,0.));
#56826=DIRECTION('center_axis',(1.,0.,0.));
#56827=DIRECTION('ref_axis',(0.,0.,-1.));
#56828=DIRECTION('center_axis',(1.,0.,0.));
#56829=DIRECTION('ref_axis',(0.,-1.,3.06161699786838E-17));
#56830=DIRECTION('center_axis',(1.,0.,0.));
#56831=DIRECTION('ref_axis',(0.,-1.,-6.09478425798614E-15));
#56832=DIRECTION('center_axis',(-1.,0.,0.));
#56833=DIRECTION('ref_axis',(0.,-1.,-1.06328749589111E-13));
#56834=DIRECTION('center_axis',(1.,0.,0.));
#56835=DIRECTION('ref_axis',(0.,0.499999999999999,0.866025403784439));
#56836=DIRECTION('center_axis',(1.,0.,0.));
#56837=DIRECTION('ref_axis',(0.,0.5,0.866025403784438));
#56838=DIRECTION('center_axis',(1.,0.,0.));
#56839=DIRECTION('ref_axis',(0.,1.,0.));
#56840=DIRECTION('center_axis',(-1.,0.,0.));
#56841=DIRECTION('ref_axis',(0.,0.499999999999946,0.86602540378447));
#56842=DIRECTION('center_axis',(1.,0.,0.));
#56843=DIRECTION('ref_axis',(0.,0.499999999999988,0.866025403784445));
#56844=DIRECTION('center_axis',(0.,-0.0997060130126144,0.995016940041288));
#56845=DIRECTION('ref_axis',(1.,0.,0.));
#56846=DIRECTION('center_axis',(1.,0.,0.));
#56847=DIRECTION('ref_axis',(0.,0.499999999999946,0.86602540378447));
#56848=DIRECTION('center_axis',(0.,0.9115629537779,0.411160529841704));
#56849=DIRECTION('ref_axis',(0.707106781098648,-0.290734398843463,0.644572346174919));
#56850=DIRECTION('center_axis',(1.,0.,0.));
#56851=DIRECTION('ref_axis',(0.,0.,-1.));
#56852=DIRECTION('center_axis',(0.,0.911562953777902,-0.411160529841698));
#56853=DIRECTION('ref_axis',(1.,0.,0.));
#56854=DIRECTION('center_axis',(1.,0.,0.));
#56855=DIRECTION('ref_axis',(0.,0.500000000000038,-0.866025403784417));
#56856=DIRECTION('center_axis',(0.,-0.099706013012563,-0.995016940041293));
#56857=DIRECTION('ref_axis',(0.707106781098668,0.703583225786129,-0.0705027979350196));
#56858=DIRECTION('center_axis',(1.,0.,0.));
#56859=DIRECTION('ref_axis',(0.,0.,-1.));
#56860=DIRECTION('center_axis',(0.,-0.811856940765334,-0.583856410199591));
#56861=DIRECTION('ref_axis',(1.,0.,0.));
#56862=DIRECTION('center_axis',(1.,0.,0.));
#56863=DIRECTION('ref_axis',(0.,-1.,-1.06328749589111E-13));
#56864=DIRECTION('center_axis',(0.,-0.811856940765331,0.583856410199595));
#56865=DIRECTION('ref_axis',(0.707106781098664,-0.41284882694268,-0.57406954823988));
#56866=DIRECTION('center_axis',(-1.,0.,0.));
#56867=DIRECTION('ref_axis',(0.,1.,0.));
#56868=DIRECTION('center_axis',(-1.,0.,0.));
#56869=DIRECTION('ref_axis',(0.,-1.,1.01064309961486E-15));
#56870=DIRECTION('center_axis',(1.,0.,0.));
#56871=DIRECTION('ref_axis',(0.,-1.,0.));
#56872=DIRECTION('',(-1.,0.,0.));
#56873=DIRECTION('',(1.,0.,0.));
#56874=DIRECTION('center_axis',(0.,-0.707106781186547,0.707106781186548));
#56875=DIRECTION('ref_axis',(0.,-0.707106781186548,-0.707106781186547));
#56876=DIRECTION('',(1.,0.,0.));
#56877=DIRECTION('center_axis',(1.,0.,0.));
#56878=DIRECTION('ref_axis',(0.,0.,1.));
#56879=DIRECTION('',(-1.,0.,0.));
#56880=DIRECTION('center_axis',(1.,0.,0.));
#56881=DIRECTION('ref_axis',(0.,-0.258819045102516,0.965925826289069));
#56882=DIRECTION('',(-1.,0.,0.));
#56883=DIRECTION('',(1.,0.,0.));
#56884=DIRECTION('center_axis',(0.,0.5,0.866025403784438));
#56885=DIRECTION('ref_axis',(0.,-0.866025403784438,0.5));
#56886=DIRECTION('',(1.,0.,0.));
#56887=DIRECTION('center_axis',(1.,0.,0.));
#56888=DIRECTION('ref_axis',(0.,-0.965925826289069,-0.25881904510252));
#56889=DIRECTION('',(-1.,0.,0.));
#56890=DIRECTION('',(1.,0.,0.));
#56891=DIRECTION('center_axis',(0.,-0.5,-0.866025403784438));
#56892=DIRECTION('ref_axis',(0.,0.866025403784438,-0.5));
#56893=DIRECTION('',(-1.,0.,0.));
#56894=DIRECTION('center_axis',(1.,0.,0.));
#56895=DIRECTION('ref_axis',(0.,0.500000000000006,0.866025403784435));
#56896=DIRECTION('center_axis',(0.,-0.0997060130125527,0.995016940041294));
#56897=DIRECTION('ref_axis',(-0.707106781098737,0.70358322578606,0.0705027979350053));
#56898=DIRECTION('center_axis',(0.,0.911562953777896,0.411160529841712));
#56899=DIRECTION('ref_axis',(-1.,0.,0.));
#56900=DIRECTION('center_axis',(1.,0.,0.));
#56901=DIRECTION('ref_axis',(0.,0.,-1.));
#56902=DIRECTION('center_axis',(0.,0.911562953777888,-0.41116052984173));
#56903=DIRECTION('ref_axis',(-0.707106781098756,-0.290734398843438,-0.644572346174811));
#56904=DIRECTION('center_axis',(0.,-0.099706013012563,-0.995016940041293));
#56905=DIRECTION('ref_axis',(-1.,0.,0.));
#56906=DIRECTION('center_axis',(1.,0.,0.));
#56907=DIRECTION('ref_axis',(0.,0.,-1.));
#56908=DIRECTION('center_axis',(0.,-0.811856940765334,-0.583856410199591));
#56909=DIRECTION('ref_axis',(-0.707106781098559,-0.412848826942738,0.574069548239967));
#56910=DIRECTION('center_axis',(0.,-0.811856940765337,0.583856410199587));
#56911=DIRECTION('ref_axis',(-1.,0.,0.));
#56912=DIRECTION('center_axis',(1.,0.,0.));
#56913=DIRECTION('ref_axis',(0.,-0.866025403784437,-0.500000000000003));
#56914=DIRECTION('',(-1.,0.,0.));
#56915=DIRECTION('',(1.,0.,0.));
#56916=DIRECTION('center_axis',(0.,-0.965925826289068,0.258819045102522));
#56917=DIRECTION('ref_axis',(0.,-0.258819045102522,-0.965925826289068));
#56918=DIRECTION('',(1.,0.,0.));
#56919=DIRECTION('center_axis',(1.,0.,0.));
#56920=DIRECTION('ref_axis',(0.,-0.499999999999996,0.866025403784441));
#56921=DIRECTION('',(-1.,0.,0.));
#56922=DIRECTION('center_axis',(0.,0.258819045102522,0.965925826289068));
#56923=DIRECTION('ref_axis',(0.,-0.965925826289068,0.258819045102522));
#56924=DIRECTION('',(1.,0.,0.));
#56925=DIRECTION('center_axis',(0.,-0.258819045102522,-0.965925826289068));
#56926=DIRECTION('ref_axis',(0.,0.965925826289068,-0.258819045102522));
#56927=DIRECTION('',(-1.,0.,0.));
#56928=DIRECTION('center_axis',(1.,0.,0.));
#56929=DIRECTION('ref_axis',(0.,1.,0.));
#56930=DIRECTION('center_axis',(1.,0.,0.));
#56931=DIRECTION('ref_axis',(0.,1.,0.));
#56932=DIRECTION('center_axis',(0.,-0.866025403784438,0.5));
#56933=DIRECTION('ref_axis',(0.,-0.5,-0.866025403784438));
#56934=DIRECTION('center_axis',(0.,0.707106781186548,0.707106781186547));
#56935=DIRECTION('ref_axis',(0.,-0.707106781186547,0.707106781186548));
#56936=DIRECTION('',(1.,0.,0.));
#56937=DIRECTION('center_axis',(0.,-0.707106781186548,-0.707106781186547));
#56938=DIRECTION('ref_axis',(0.,0.707106781186547,-0.707106781186548));
#56939=DIRECTION('',(-1.,0.,0.));
#56940=DIRECTION('center_axis',(1.,0.,0.));
#56941=DIRECTION('ref_axis',(0.,1.,0.));
#56942=DIRECTION('center_axis',(0.,-0.499999999999999,0.866025403784439));
#56943=DIRECTION('ref_axis',(0.,-0.866025403784439,-0.499999999999999));
#56944=DIRECTION('center_axis',(1.,0.,0.));
#56945=DIRECTION('ref_axis',(0.,1.,0.));
#56946=DIRECTION('center_axis',(1.,0.,0.));
#56947=DIRECTION('ref_axis',(0.,1.,0.));
#56948=DIRECTION('',(1.,0.,0.));
#56949=DIRECTION('center_axis',(0.,-0.965925826289068,-0.25881904510252));
#56950=DIRECTION('ref_axis',(0.,0.25881904510252,-0.965925826289068));
#56951=DIRECTION('',(-1.,0.,0.));
#56952=DIRECTION('center_axis',(0.,0.965925826289068,0.25881904510252));
#56953=DIRECTION('ref_axis',(0.,-0.25881904510252,0.965925826289068));
#56954=DIRECTION('center_axis',(0.,1.,-1.83697019872103E-16));
#56955=DIRECTION('ref_axis',(0.,1.83697019872103E-16,1.));
#56956=DIRECTION('',(1.,0.,0.));
#56957=DIRECTION('center_axis',(0.,-1.,1.83697019872103E-16));
#56958=DIRECTION('ref_axis',(0.,-1.83697019872103E-16,-1.));
#56959=DIRECTION('',(-1.,0.,0.));
#56960=DIRECTION('center_axis',(1.,0.,0.));
#56961=DIRECTION('ref_axis',(0.,1.,0.));
#56962=DIRECTION('center_axis',(0.,0.258819045102522,0.965925826289068));
#56963=DIRECTION('ref_axis',(0.,-0.965925826289068,0.258819045102522));
#56964=DIRECTION('center_axis',(1.,0.,0.));
#56965=DIRECTION('ref_axis',(0.,1.,0.));
#56966=DIRECTION('center_axis',(1.,0.,0.));
#56967=DIRECTION('ref_axis',(0.,1.,0.));
#56968=DIRECTION('',(1.,0.,0.));
#56969=DIRECTION('center_axis',(0.,-0.866025403784438,0.5));
#56970=DIRECTION('ref_axis',(0.,-0.5,-0.866025403784438));
#56971=DIRECTION('',(-1.,0.,0.));
#56972=DIRECTION('center_axis',(0.,0.866025403784438,-0.5));
#56973=DIRECTION('ref_axis',(0.,0.5,0.866025403784438));
#56974=DIRECTION('center_axis',(0.,0.707106781186547,-0.707106781186548));
#56975=DIRECTION('ref_axis',(0.,0.707106781186548,0.707106781186547));
#56976=DIRECTION('',(1.,0.,0.));
#56977=DIRECTION('center_axis',(0.,-0.707106781186547,0.707106781186548));
#56978=DIRECTION('ref_axis',(0.,-0.707106781186548,-0.707106781186547));
#56979=DIRECTION('',(-1.,0.,0.));
#56980=DIRECTION('center_axis',(1.,0.,0.));
#56981=DIRECTION('ref_axis',(0.,1.,0.));
#56982=DIRECTION('center_axis',(0.,0.866025403784439,0.5));
#56983=DIRECTION('ref_axis',(0.,-0.5,0.866025403784439));
#56984=DIRECTION('center_axis',(1.,0.,0.));
#56985=DIRECTION('ref_axis',(0.,1.,0.));
#56986=DIRECTION('center_axis',(1.,0.,0.));
#56987=DIRECTION('ref_axis',(0.,1.,0.));
#56988=DIRECTION('',(1.,0.,0.));
#56989=DIRECTION('center_axis',(0.,-0.25881904510252,0.965925826289068));
#56990=DIRECTION('ref_axis',(0.,-0.965925826289068,-0.25881904510252));
#56991=DIRECTION('',(-1.,0.,0.));
#56992=DIRECTION('center_axis',(0.,0.25881904510252,-0.965925826289068));
#56993=DIRECTION('ref_axis',(0.,0.965925826289068,0.25881904510252));
#56994=DIRECTION('center_axis',(0.,-1.22464679914735E-16,-1.));
#56995=DIRECTION('ref_axis',(0.,1.,-1.22464679914735E-16));
#56996=DIRECTION('',(1.,0.,0.));
#56997=DIRECTION('center_axis',(0.,1.22464679914735E-16,1.));
#56998=DIRECTION('ref_axis',(0.,-1.,1.22464679914735E-16));
#56999=DIRECTION('',(-1.,0.,0.));
#57000=DIRECTION('center_axis',(1.,0.,0.));
#57001=DIRECTION('ref_axis',(0.,1.,0.));
#57002=DIRECTION('center_axis',(0.,0.965925826289068,-0.258819045102521));
#57003=DIRECTION('ref_axis',(0.,0.258819045102521,0.965925826289068));
#57004=DIRECTION('center_axis',(1.,0.,0.));
#57005=DIRECTION('ref_axis',(0.,1.,0.));
#57006=DIRECTION('center_axis',(1.,0.,0.));
#57007=DIRECTION('ref_axis',(0.,1.,0.));
#57008=DIRECTION('',(1.,0.,0.));
#57009=DIRECTION('center_axis',(0.,0.5,0.866025403784438));
#57010=DIRECTION('ref_axis',(0.,-0.866025403784438,0.5));
#57011=DIRECTION('',(-1.,0.,0.));
#57012=DIRECTION('center_axis',(0.,-0.5,-0.866025403784438));
#57013=DIRECTION('ref_axis',(0.,0.866025403784438,-0.5));
#57014=DIRECTION('center_axis',(0.,-0.707106781186548,-0.707106781186547));
#57015=DIRECTION('ref_axis',(0.,0.707106781186547,-0.707106781186548));
#57016=DIRECTION('',(1.,0.,0.));
#57017=DIRECTION('center_axis',(0.,0.707106781186548,0.707106781186547));
#57018=DIRECTION('ref_axis',(0.,-0.707106781186547,0.707106781186548));
#57019=DIRECTION('',(-1.,0.,0.));
#57020=DIRECTION('center_axis',(1.,0.,0.));
#57021=DIRECTION('ref_axis',(0.,1.,0.));
#57022=DIRECTION('center_axis',(0.,0.5,-0.866025403784439));
#57023=DIRECTION('ref_axis',(0.,0.866025403784439,0.5));
#57024=DIRECTION('center_axis',(1.,0.,0.));
#57025=DIRECTION('ref_axis',(0.,1.,0.));
#57026=DIRECTION('center_axis',(1.,0.,0.));
#57027=DIRECTION('ref_axis',(0.,1.,0.));
#57028=DIRECTION('',(1.,0.,0.));
#57029=DIRECTION('center_axis',(0.,0.965925826289068,0.258819045102521));
#57030=DIRECTION('ref_axis',(0.,-0.258819045102521,0.965925826289068));
#57031=DIRECTION('',(-1.,0.,0.));
#57032=DIRECTION('center_axis',(0.,-0.965925826289068,-0.258819045102521));
#57033=DIRECTION('ref_axis',(0.,0.258819045102521,-0.965925826289068));
#57034=DIRECTION('center_axis',(0.,-1.,6.12323399573677E-17));
#57035=DIRECTION('ref_axis',(0.,-6.12323399573677E-17,-1.));
#57036=DIRECTION('',(1.,0.,0.));
#57037=DIRECTION('center_axis',(0.,1.,-6.12323399573677E-17));
#57038=DIRECTION('ref_axis',(0.,6.12323399573677E-17,1.));
#57039=DIRECTION('',(-1.,0.,0.));
#57040=DIRECTION('center_axis',(1.,0.,0.));
#57041=DIRECTION('ref_axis',(0.,1.,0.));
#57042=DIRECTION('center_axis',(0.,-0.258819045102521,-0.965925826289068));
#57043=DIRECTION('ref_axis',(0.,0.965925826289068,-0.258819045102521));
#57044=DIRECTION('center_axis',(1.,0.,0.));
#57045=DIRECTION('ref_axis',(0.,1.,0.));
#57046=DIRECTION('center_axis',(1.,0.,0.));
#57047=DIRECTION('ref_axis',(0.,1.,0.));
#57048=DIRECTION('',(1.,0.,0.));
#57049=DIRECTION('center_axis',(0.,0.866025403784439,-0.5));
#57050=DIRECTION('ref_axis',(0.,0.5,0.866025403784439));
#57051=DIRECTION('',(-1.,0.,0.));
#57052=DIRECTION('center_axis',(0.,-0.866025403784439,0.5));
#57053=DIRECTION('ref_axis',(0.,-0.5,-0.866025403784439));
#57054=DIRECTION('center_axis',(0.,-0.707106781186548,0.707106781186548));
#57055=DIRECTION('ref_axis',(0.,-0.707106781186548,-0.707106781186548));
#57056=DIRECTION('',(1.,0.,0.));
#57057=DIRECTION('center_axis',(0.,0.707106781186548,-0.707106781186548));
#57058=DIRECTION('ref_axis',(0.,0.707106781186548,0.707106781186548));
#57059=DIRECTION('',(-1.,0.,0.));
#57060=DIRECTION('center_axis',(1.,0.,0.));
#57061=DIRECTION('ref_axis',(0.,1.,0.));
#57062=DIRECTION('center_axis',(0.,-0.866025403784439,-0.5));
#57063=DIRECTION('ref_axis',(0.,0.5,-0.866025403784439));
#57064=DIRECTION('center_axis',(1.,0.,0.));
#57065=DIRECTION('ref_axis',(0.,1.,0.));
#57066=DIRECTION('center_axis',(1.,0.,0.));
#57067=DIRECTION('ref_axis',(0.,1.,0.));
#57068=DIRECTION('',(1.,0.,0.));
#57069=DIRECTION('center_axis',(0.,0.258819045102521,-0.965925826289068));
#57070=DIRECTION('ref_axis',(0.,0.965925826289068,0.258819045102521));
#57071=DIRECTION('',(-1.,0.,0.));
#57072=DIRECTION('center_axis',(0.,-0.258819045102521,0.965925826289068));
#57073=DIRECTION('ref_axis',(0.,-0.965925826289068,-0.258819045102521));
#57074=DIRECTION('center_axis',(0.,-1.,0.));
#57075=DIRECTION('ref_axis',(0.,0.,-1.));
#57076=DIRECTION('center_axis',(-1.,0.,0.));
#57077=DIRECTION('ref_axis',(0.,1.,0.));
#57078=DIRECTION('center_axis',(1.,0.,0.));
#57079=DIRECTION('ref_axis',(0.,1.,0.));
#88374=CARTESIAN_POINT('',(0.,0.,0.));
#88375=CARTESIAN_POINT('Origin',(527.,27.1,0.));
#88376=CARTESIAN_POINT('',(527.,27.5,-8.59999999999999));
#88377=CARTESIAN_POINT('Origin',(527.,27.5,0.));
#88378=CARTESIAN_POINT('',(527.,27.1,-8.99999999999999));
#88379=CARTESIAN_POINT('Origin',(527.,27.1,-8.59999999999999));
#88380=CARTESIAN_POINT('',(518.,27.1,1.10218211923262E-15));
#88381=CARTESIAN_POINT('Origin',(527.,27.1,0.));
#88382=CARTESIAN_POINT('Origin',(527.,27.1,0.));
#88383=CARTESIAN_POINT('Origin',(527.,13.,0.));
#88384=CARTESIAN_POINT('',(518.,14.4,0.));
#88385=CARTESIAN_POINT('',(518.,13.,1.10218211923262E-15));
#88386=CARTESIAN_POINT('',(518.117157287549,14.4448174223783,1.44744787341983));
#88387=CARTESIAN_POINT('Ctrl Pts',(518.11715728757,14.4448174223773,1.4474478734047));
#88388=CARTESIAN_POINT('Ctrl Pts',(518.041461163612,14.4152915542387,0.982908337704877));
#88389=CARTESIAN_POINT('Ctrl Pts',(518.000676801706,14.4002754503427,0.499523458887916));
#88390=CARTESIAN_POINT('Ctrl Pts',(518.000009683209,14.4000036894498,0.0132961349833423));
#88391=CARTESIAN_POINT('Ctrl Pts',(518.000003601837,14.4000012121102,0.00886374519088948));
#88392=CARTESIAN_POINT('Ctrl Pts',(518.,14.4000000000001,0.00443224585609541));
#88393=CARTESIAN_POINT('Ctrl Pts',(518.,14.4000000000001,3.05311331771918E-15));
#88394=CARTESIAN_POINT('',(518.482842712485,14.5959232481191,2.90826954389088));
#88395=CARTESIAN_POINT('Ctrl Pts',(518.482842712495,14.5959232481186,2.90826954388758));
#88396=CARTESIAN_POINT('Ctrl Pts',(518.444859936036,14.5793579098115,2.79703319648565));
#88397=CARTESIAN_POINT('Ctrl Pts',(518.408958670823,14.5639684796705,2.68475891749876));
#88398=CARTESIAN_POINT('Ctrl Pts',(518.2652421474,14.5032163043335,2.2027721309851));
#88399=CARTESIAN_POINT('Ctrl Pts',(518.178681115507,14.4688152750555,1.82501344703967));
#88400=CARTESIAN_POINT('Ctrl Pts',(518.117157287572,14.4448174223781,1.44744787341611));
#88401=CARTESIAN_POINT('',(518.765685425361,14.5534853731784,3.63263864053153));
#88402=CARTESIAN_POINT('Ctrl Pts',(518.482842712495,14.5959232481186,2.90826954388759));
#88403=CARTESIAN_POINT('Ctrl Pts',(518.484338637184,14.5965756622086,2.91265050846784));
#88404=CARTESIAN_POINT('Ctrl Pts',(518.485847944177,14.5972101270179,2.91705961064773));
#88405=CARTESIAN_POINT('Ctrl Pts',(518.556292080332,14.6257255154875,3.12231910261073));
#88406=CARTESIAN_POINT('Ctrl Pts',(518.653850216063,14.6167613702112,3.37913522636895));
#88407=CARTESIAN_POINT('Ctrl Pts',(518.765685424949,14.5534853736448,3.63263863866276));
#88408=CARTESIAN_POINT('',(521.036779393934,13.3999999999368,6.74091981879216));
#88409=CARTESIAN_POINT('Ctrl Pts',(521.036779393919,13.39999999988,6.7409198187796));
#88410=CARTESIAN_POINT('Ctrl Pts',(520.89804042185,13.4617411265306,6.61818714737095));
#88411=CARTESIAN_POINT('Ctrl Pts',(520.76436353255,13.5229549178595,6.49228559390815));
#88412=CARTESIAN_POINT('Ctrl Pts',(519.890508026718,13.932374822938,5.61843008807617));
#88413=CARTESIAN_POINT('Ctrl Pts',(519.227527232995,14.2921767844317,4.67952249017717));
#88414=CARTESIAN_POINT('Ctrl Pts',(518.76568542571,14.5534853732145,3.63263864038689));
#88415=CARTESIAN_POINT('',(532.963220606066,13.3999999999368,6.74091981879216));
#88416=CARTESIAN_POINT('Origin',(527.,13.4,0.));
#88417=CARTESIAN_POINT('',(535.234314574639,14.5534853731784,3.63263864053159));
#88418=CARTESIAN_POINT('Ctrl Pts',(535.23431457429,14.5534853732145,3.63263864038688));
#88419=CARTESIAN_POINT('Ctrl Pts',(534.772472767005,14.2921767844317,4.67952249017712));
#88420=CARTESIAN_POINT('Ctrl Pts',(534.109491973282,13.932374822938,5.61843008807619));
#88421=CARTESIAN_POINT('Ctrl Pts',(533.23563646745,13.5229549178595,6.49228559390812));
#88422=CARTESIAN_POINT('Ctrl Pts',(533.10195957815,13.4617411265306,6.61818714737088));
#88423=CARTESIAN_POINT('Ctrl Pts',(532.963220606081,13.3999999998801,6.74091981877953));
#88424=CARTESIAN_POINT('',(535.517157287515,14.595923248119,2.90826954389093));
#88425=CARTESIAN_POINT('Ctrl Pts',(535.234314575051,14.5534853736448,3.63263863866289));
#88426=CARTESIAN_POINT('Ctrl Pts',(535.347942428929,14.6177756429034,3.37507173306295));
#88427=CARTESIAN_POINT('Ctrl Pts',(535.447565241837,14.626274262105,3.11207678732332));
#88428=CARTESIAN_POINT('Ctrl Pts',(535.517157287505,14.5959232481186,2.90826954388767));
#88429=CARTESIAN_POINT('',(535.882842712451,14.4448174223783,1.44744787342066));
#88430=CARTESIAN_POINT('Ctrl Pts',(535.882842712428,14.444817422378,1.44744787341694));
#88431=CARTESIAN_POINT('Ctrl Pts',(535.821318884493,14.4688152750555,1.82501344704022));
#88432=CARTESIAN_POINT('Ctrl Pts',(535.7347578526,14.5032163043335,2.20277213098536));
#88433=CARTESIAN_POINT('Ctrl Pts',(535.591041329177,14.5639684796705,2.68475891749878));
#88434=CARTESIAN_POINT('Ctrl Pts',(535.555140063964,14.5793579098115,2.79703319648571));
#88435=CARTESIAN_POINT('Ctrl Pts',(535.517157287505,14.5959232481186,2.90826954388771));
#88436=CARTESIAN_POINT('',(536.,14.4,0.));
#88437=CARTESIAN_POINT('Ctrl Pts',(536.,14.4,-7.49400541621981E-15));
#88438=CARTESIAN_POINT('Ctrl Pts',(536.,14.4,0.0044321487043113));
#88439=CARTESIAN_POINT('Ctrl Pts',(535.999996398319,14.4000012120569,0.00886355094690782));
#88440=CARTESIAN_POINT('Ctrl Pts',(535.999990317216,14.4000036892881,0.0132958436075195));
#88441=CARTESIAN_POINT('Ctrl Pts',(535.999323213544,14.4002754442916,0.499523265098869));
#88442=CARTESIAN_POINT('Ctrl Pts',(535.958538851494,14.4152915483467,0.982908245004447));
#88443=CARTESIAN_POINT('Ctrl Pts',(535.88284271243,14.4448174223773,1.44744787340554));
#88444=CARTESIAN_POINT('',(535.882842712451,14.4448174223783,-1.44744787342017));
#88445=CARTESIAN_POINT('Ctrl Pts',(535.88284271243,14.4448174223773,-1.44744787340509));
#88446=CARTESIAN_POINT('Ctrl Pts',(535.95853884256,14.4152915518312,-0.982908299828285));
#88447=CARTESIAN_POINT('Ctrl Pts',(535.999323204044,14.400275447844,-0.499523379163677));
#88448=CARTESIAN_POINT('Ctrl Pts',(535.999990316963,14.4000036893836,-0.013296015930175));
#88449=CARTESIAN_POINT('Ctrl Pts',(535.99999639823,14.4000012120886,-0.00886366582987909));
#88450=CARTESIAN_POINT('Ctrl Pts',(536.,14.4,-0.00443220616197504));
#88451=CARTESIAN_POINT('Ctrl Pts',(536.,14.4,-5.90673343570102E-15));
#88452=CARTESIAN_POINT('',(535.517157287515,14.595923248119,-2.90826954389091));
#88453=CARTESIAN_POINT('Ctrl Pts',(535.517157287505,14.5959232481185,-2.90826954388764));
#88454=CARTESIAN_POINT('Ctrl Pts',(535.555140063964,14.5793579098114,-2.79703319648567));
#88455=CARTESIAN_POINT('Ctrl Pts',(535.591041329177,14.5639684796705,-2.68475891749877));
#88456=CARTESIAN_POINT('Ctrl Pts',(535.7347578526,14.5032163043335,-2.20277213098522));
#88457=CARTESIAN_POINT('Ctrl Pts',(535.821318884493,14.4688152750555,-1.82501344703992));
#88458=CARTESIAN_POINT('Ctrl Pts',(535.882842712428,14.444817422378,-1.44744787341649));
#88459=CARTESIAN_POINT('',(535.234314574639,14.5534853731784,-3.63263864053166));
#88460=CARTESIAN_POINT('Ctrl Pts',(535.517157287505,14.5959232481186,-2.90826954388765));
#88461=CARTESIAN_POINT('Ctrl Pts',(535.515661362816,14.5965756622085,-2.91265050846808));
#88462=CARTESIAN_POINT('Ctrl Pts',(535.514152055823,14.5972101270179,-2.91705961064816));
#88463=CARTESIAN_POINT('Ctrl Pts',(535.443707919668,14.6257255154874,-3.12231910261118));
#88464=CARTESIAN_POINT('Ctrl Pts',(535.346149783936,14.6167613702111,-3.37913522636925));
#88465=CARTESIAN_POINT('Ctrl Pts',(535.234314575051,14.5534853736448,-3.63263863866293));
#88466=CARTESIAN_POINT('',(532.963220606066,13.3999999999368,-6.74091981879216));
#88467=CARTESIAN_POINT('Ctrl Pts',(532.963220606081,13.39999999988,-6.74091981877961));
#88468=CARTESIAN_POINT('Ctrl Pts',(533.10195957815,13.4617411265306,-6.61818714737096));
#88469=CARTESIAN_POINT('Ctrl Pts',(533.23563646745,13.5229549178595,-6.49228559390813));
#88470=CARTESIAN_POINT('Ctrl Pts',(534.109491973282,13.932374822938,-5.61843008807619));
#88471=CARTESIAN_POINT('Ctrl Pts',(534.772472767005,14.2921767844317,-4.67952249017721));
#88472=CARTESIAN_POINT('Ctrl Pts',(535.23431457429,14.5534853732145,-3.63263864038694));
#88473=CARTESIAN_POINT('',(521.036779393934,13.3999999999368,-6.74091981879216));
#88474=CARTESIAN_POINT('Origin',(527.,13.4,0.));
#88475=CARTESIAN_POINT('',(518.765685425361,14.5534853731784,-3.63263864053138));
#88476=CARTESIAN_POINT('Ctrl Pts',(518.76568542571,14.5534853732145,-3.6326386403867));
#88477=CARTESIAN_POINT('Ctrl Pts',(519.227527232995,14.2921767844318,-4.67952249017704));
#88478=CARTESIAN_POINT('Ctrl Pts',(519.890508026718,13.932374822938,-5.61843008807613));
#88479=CARTESIAN_POINT('Ctrl Pts',(520.76436353255,13.5229549178595,-6.49228559390816));
#88480=CARTESIAN_POINT('Ctrl Pts',(520.89804042185,13.4617411265306,-6.61818714737101));
#88481=CARTESIAN_POINT('Ctrl Pts',(521.03677939392,13.39999999988,-6.74091981877968));
#88482=CARTESIAN_POINT('',(518.482842712485,14.5959232481191,-2.90826954389069));
#88483=CARTESIAN_POINT('Ctrl Pts',(518.765685424949,14.5534853736448,-3.63263863866275));
#88484=CARTESIAN_POINT('Ctrl Pts',(518.652057571071,14.6177756429034,-3.37507173306315));
#88485=CARTESIAN_POINT('Ctrl Pts',(518.552434758163,14.6262742621051,-3.11207678732333));
#88486=CARTESIAN_POINT('Ctrl Pts',(518.482842712495,14.5959232481186,-2.9082695438874));
#88487=CARTESIAN_POINT('',(518.117157287549,14.4448174223783,-1.44744787342002));
#88488=CARTESIAN_POINT('Ctrl Pts',(518.117157287572,14.4448174223781,-1.44744787341633));
#88489=CARTESIAN_POINT('Ctrl Pts',(518.178681115507,14.4688152750555,-1.82501344703981));
#88490=CARTESIAN_POINT('Ctrl Pts',(518.2652421474,14.5032163043335,-2.20277213098516));
#88491=CARTESIAN_POINT('Ctrl Pts',(518.408958670823,14.5639684796705,-2.6847589174987));
#88492=CARTESIAN_POINT('Ctrl Pts',(518.444859936036,14.5793579098115,-2.79703319648552));
#88493=CARTESIAN_POINT('Ctrl Pts',(518.482842712495,14.5959232481186,-2.90826954388741));
#88494=CARTESIAN_POINT('Ctrl Pts',(518.,14.4000000000001,-1.94289029309402E-15));
#88495=CARTESIAN_POINT('Ctrl Pts',(518.,14.4000000000001,-0.00443218895692087));
#88496=CARTESIAN_POINT('Ctrl Pts',(518.000003601749,14.4000012120789,-0.00886363141148919));
#88497=CARTESIAN_POINT('Ctrl Pts',(518.000009682959,14.4000036893552,-0.0132959643112483));
#88498=CARTESIAN_POINT('Ctrl Pts',(518.00067679229,14.4002754468243,-0.499523345966166));
#88499=CARTESIAN_POINT('Ctrl Pts',(518.041461154763,14.4152915507873,-0.982908283402282));
#88500=CARTESIAN_POINT('Ctrl Pts',(518.11715728757,14.4448174223773,-1.4474478734049));
#88501=CARTESIAN_POINT('Origin',(527.,27.5,0.));
#88502=CARTESIAN_POINT('Origin',(527.,13.4,0.));
#88503=CARTESIAN_POINT('',(522.762075979917,13.,7.48331477354788));
#88504=CARTESIAN_POINT('Ctrl Pts',(522.762075979917,13.,7.48331477354788));
#88505=CARTESIAN_POINT('Ctrl Pts',(522.758255200061,13.,7.48331477354788));
#88506=CARTESIAN_POINT('Ctrl Pts',(522.754457930714,13.0000132945833,7.48329167832103));
#88507=CARTESIAN_POINT('Ctrl Pts',(522.640184871778,13.0007813107163,7.48195746625073));
#88508=CARTESIAN_POINT('Ctrl Pts',(522.499127201908,13.0122592484113,7.46212072251574));
#88509=CARTESIAN_POINT('Ctrl Pts',(522.130810325902,13.0650070471598,7.36948010516466));
#88510=CARTESIAN_POINT('Ctrl Pts',(521.8916878721,13.1142349452338,7.28268176308246));
#88511=CARTESIAN_POINT('Ctrl Pts',(521.428177636549,13.2450263831268,7.04175578900627));
#88512=CARTESIAN_POINT('Ctrl Pts',(521.218157792946,13.3192836262514,6.90137261094146));
#88513=CARTESIAN_POINT('Ctrl Pts',(521.03677939365,13.4,6.7409198185411));
#88514=CARTESIAN_POINT('',(531.237924020083,13.,7.48331477354788));
#88515=CARTESIAN_POINT('Origin',(527.,13.,0.));
#88516=CARTESIAN_POINT('Ctrl Pts',(532.96322060635,13.4,6.74091981854106));
#88517=CARTESIAN_POINT('Ctrl Pts',(532.699729877776,13.2827422878942,6.97401164940602));
#88518=CARTESIAN_POINT('Ctrl Pts',(532.366534064585,13.1751277840526,7.17218290438412));
#88519=CARTESIAN_POINT('Ctrl Pts',(531.791717805958,13.0508542242612,7.39493792424501));
#88520=CARTESIAN_POINT('Ctrl Pts',(531.578769165016,13.0196868092363,7.44905510533166));
#88521=CARTESIAN_POINT('Ctrl Pts',(531.344918498116,13.0023281808315,7.47927425976839));
#88522=CARTESIAN_POINT('Ctrl Pts',(531.288493822179,13.,7.48331477354788));
#88523=CARTESIAN_POINT('Ctrl Pts',(531.237924020083,13.,7.48331477354788));
#88524=CARTESIAN_POINT('Origin',(527.,13.,0.));
#88525=CARTESIAN_POINT('',(527.,13.,7.48331477354788));
#88526=CARTESIAN_POINT('Origin',(527.,13.4,0.));
#88527=CARTESIAN_POINT('',(531.237924020083,13.,-7.48331477354788));
#88528=CARTESIAN_POINT('Ctrl Pts',(531.237924020083,13.,-7.48331477354788));
#88529=CARTESIAN_POINT('Ctrl Pts',(531.241744799939,13.,-7.48331477354788));
#88530=CARTESIAN_POINT('Ctrl Pts',(531.245542069286,13.0000132945833,-7.48329167832103));
#88531=CARTESIAN_POINT('Ctrl Pts',(531.359815128221,13.0007813107163,-7.48195746625072));
#88532=CARTESIAN_POINT('Ctrl Pts',(531.500872798091,13.0122592484112,-7.46212072251603));
#88533=CARTESIAN_POINT('Ctrl Pts',(531.869189674095,13.0650070471594,-7.36948010516544));
#88534=CARTESIAN_POINT('Ctrl Pts',(532.108312127896,13.1142349452328,-7.28268176308435));
#88535=CARTESIAN_POINT('Ctrl Pts',(532.571822363452,13.2450263831268,-7.04175578900614));
#88536=CARTESIAN_POINT('Ctrl Pts',(532.781842207054,13.3192836262514,-6.90137261094135));
#88537=CARTESIAN_POINT('Ctrl Pts',(532.96322060635,13.4,-6.74091981854107));
#88538=CARTESIAN_POINT('',(522.762075979917,13.,-7.48331477354788));
#88539=CARTESIAN_POINT('Origin',(527.,13.,0.));
#88540=CARTESIAN_POINT('Ctrl Pts',(521.03677939365,13.4,-6.7409198185411));
#88541=CARTESIAN_POINT('Ctrl Pts',(521.300270122226,13.2827422878936,-6.97401164940719));
#88542=CARTESIAN_POINT('Ctrl Pts',(521.633465935416,13.1751277840522,-7.17218290438478));
#88543=CARTESIAN_POINT('Ctrl Pts',(522.208282194043,13.050854224261,-7.39493792424534));
#88544=CARTESIAN_POINT('Ctrl Pts',(522.421230834985,13.0196868092362,-7.44905510533174));
#88545=CARTESIAN_POINT('Ctrl Pts',(522.655081501884,13.0023281808315,-7.47927425976842));
#88546=CARTESIAN_POINT('Ctrl Pts',(522.711506177821,13.,-7.48331477354788));
#88547=CARTESIAN_POINT('Ctrl Pts',(522.762075979917,13.,-7.48331477354788));
#88548=CARTESIAN_POINT('Origin',(527.,13.,0.));
#88549=CARTESIAN_POINT('',(527.,13.,-7.48331477354788));
#88550=CARTESIAN_POINT('Origin',(535.234314575051,0.,0.));
#88551=CARTESIAN_POINT('',(535.234314574639,-4.13078534111998,14.4200073670435));
#88552=CARTESIAN_POINT('Origin',(535.234314575051,0.,0.));
#88553=CARTESIAN_POINT('',(535.517157287515,-4.77932631799744,14.0945750965044));
#88554=CARTESIAN_POINT('Ctrl Pts',(535.517157287505,-4.77932631800001,14.0945750965023));
#88555=CARTESIAN_POINT('Ctrl Pts',(535.515267590893,-4.77494566505028,14.0980559128472));
#88556=CARTESIAN_POINT('Ctrl Pts',(535.513356428073,-4.77051154796902,14.1015345793545));
#88557=CARTESIAN_POINT('Ctrl Pts',(535.442576431487,-4.60618275816504,14.2288316588691));
#88558=CARTESIAN_POINT('Ctrl Pts',(535.345485582019,-4.38047195944321,14.3484816183326));
#88559=CARTESIAN_POINT('Ctrl Pts',(535.234314575051,-4.13078534297138,14.4200073665131));
#88560=CARTESIAN_POINT('Origin',(535.517157287525,5.55111512312578E-16,
-1.11022302462516E-15));
#88561=CARTESIAN_POINT('Origin',(527.,0.,0.));
#88562=CARTESIAN_POINT('',(518.765685425361,-4.13078534112005,14.4200073670435));
#88563=CARTESIAN_POINT('Origin',(518.765685424949,0.,0.));
#88564=CARTESIAN_POINT('',(521.036779393934,-0.862192192020416,14.9752003200529));
#88565=CARTESIAN_POINT('Ctrl Pts',(518.76568542571,-4.13078534126337,14.4200073670024));
#88566=CARTESIAN_POINT('Ctrl Pts',(519.227527232995,-3.09350303814188,14.7171494157847));
#88567=CARTESIAN_POINT('Ctrl Pts',(519.890508026718,-2.10048422580824,14.8750055757491));
#88568=CARTESIAN_POINT('Ctrl Pts',(520.76436353255,-1.13899320598154,14.9573652900521));
#88569=CARTESIAN_POINT('Ctrl Pts',(520.89804042185,-0.999352366642388,14.9673033684307));
#88570=CARTESIAN_POINT('Ctrl Pts',(521.036779393919,-0.862192192002862,
14.9752003199974));
#88571=CARTESIAN_POINT('',(522.762075979917,-0.0192593015921383,14.9999876359716));
#88572=CARTESIAN_POINT('Ctrl Pts',(521.03677939365,-0.86219219226942,14.975200319982));
#88573=CARTESIAN_POINT('Ctrl Pts',(521.300270122228,-0.601699889269615,
14.9901980779414));
#88574=CARTESIAN_POINT('Ctrl Pts',(521.633465935419,-0.376271296239237,
14.9960868112878));
#88575=CARTESIAN_POINT('Ctrl Pts',(522.208282194045,-0.121223010324114,
14.9998402614201));
#88576=CARTESIAN_POINT('Ctrl Pts',(522.421230834987,-0.0587724492104019,
14.9999070787816));
#88577=CARTESIAN_POINT('Ctrl Pts',(522.655081501885,-0.0239225795851385,
14.9999836428266));
#88578=CARTESIAN_POINT('Ctrl Pts',(522.711506177822,-0.0192593015921411,
14.9999876359716));
#88579=CARTESIAN_POINT('Ctrl Pts',(522.762075979917,-0.0192593015921407,
14.9999876359716));
#88580=CARTESIAN_POINT('',(531.237924020083,-0.0192593015921383,14.9999876359716));
#88581=CARTESIAN_POINT('',(527.,-0.0192593015921383,14.9999876359716));
#88582=CARTESIAN_POINT('',(532.963220606066,-0.862192192020414,14.9752003200529));
#88583=CARTESIAN_POINT('Ctrl Pts',(531.237924020083,-0.0192593015921382,
14.9999876359716));
#88584=CARTESIAN_POINT('Ctrl Pts',(531.241744799939,-0.0192593015921378,
14.9999876359716));
#88585=CARTESIAN_POINT('Ctrl Pts',(531.245542069286,-0.0192859499369423,
14.9999876018051));
#88586=CARTESIAN_POINT('Ctrl Pts',(531.35981512822,-0.0208254195503694,
14.9999856172516));
#88587=CARTESIAN_POINT('Ctrl Pts',(531.50087279809,-0.0437435124002363,
15.0000074310111));
#88588=CARTESIAN_POINT('Ctrl Pts',(531.869189674095,-0.150346539822359,
14.9993680560455));
#88589=CARTESIAN_POINT('Ctrl Pts',(532.108312127896,-0.250130058107601,
14.9986014953114));
#88590=CARTESIAN_POINT('Ctrl Pts',(532.571822363452,-0.524173791037977,
14.991407216086));
#88591=CARTESIAN_POINT('Ctrl Pts',(532.781842207054,-0.682877811068355,
14.9855242860145));
#88592=CARTESIAN_POINT('Ctrl Pts',(532.96322060635,-0.862192192269444,14.975200319982));
#88593=CARTESIAN_POINT('Ctrl Pts',(532.963220606081,-0.862192192002855,
14.9752003199974));
#88594=CARTESIAN_POINT('Ctrl Pts',(533.10195957815,-0.999352366642365,14.9673033684307));
#88595=CARTESIAN_POINT('Ctrl Pts',(533.23563646745,-1.13899320598154,14.9573652900521));
#88596=CARTESIAN_POINT('Ctrl Pts',(534.109491973282,-2.10048422580822,14.8750055757491));
#88597=CARTESIAN_POINT('Ctrl Pts',(534.772472767005,-3.09350303814185,14.7171494157847));
#88598=CARTESIAN_POINT('Ctrl Pts',(535.23431457429,-4.13078534126331,14.4200073670024));
#88599=CARTESIAN_POINT('Origin',(527.,-13.55,23.4692884425583));
#88600=CARTESIAN_POINT('',(518.4,-13.75,23.8156986040721));
#88601=CARTESIAN_POINT('Origin',(527.,-13.75,23.8156986040721));
#88602=CARTESIAN_POINT('',(518.,-13.55,23.4692884425583));
#88603=CARTESIAN_POINT('Origin',(518.4,-13.55,23.4692884425583));
#88604=CARTESIAN_POINT('Origin',(527.,-13.55,23.4692884425583));
#88605=CARTESIAN_POINT('Origin',(527.,-6.5,11.2583302491977));
#88606=CARTESIAN_POINT('',(518.,-7.20000000000156,12.470765814495));
#88607=CARTESIAN_POINT('',(518.,-6.5,11.2583302491977));
#88608=CARTESIAN_POINT('',(518.117157287549,-8.47593534022486,11.7858549040976));
#88609=CARTESIAN_POINT('Ctrl Pts',(518.11715728757,-8.47593534021129,11.7858549041043));
#88610=CARTESIAN_POINT('Ctrl Pts',(518.041461163612,-8.05886936716401,11.9925545200772));
#88611=CARTESIAN_POINT('Ctrl Pts',(518.000676796169,-7.63273773832445,12.2212426277938));
#88612=CARTESIAN_POINT('Ctrl Pts',(518.000009683192,-7.2115166354102,12.4641209421524));
#88613=CARTESIAN_POINT('Ctrl Pts',(518.000003601871,-7.20767683450791,12.4663349916484));
#88614=CARTESIAN_POINT('Ctrl Pts',(518.,-7.20383843749968,12.4685496915723));
#88615=CARTESIAN_POINT('Ctrl Pts',(518.,-7.20000000000003,12.470765814496));
#88616=CARTESIAN_POINT('',(518.482842712485,-9.81659693012145,11.1863055526137));
#88617=CARTESIAN_POINT('Ctrl Pts',(518.482842712495,-9.81659693011836,11.1863055526149));
#88618=CARTESIAN_POINT('Ctrl Pts',(518.444859936036,-9.71198075829059,11.2275777225196));
#88619=CARTESIAN_POINT('Ctrl Pts',(518.408958670823,-9.60705366542595,11.2703872245612));
#88620=CARTESIAN_POINT('Ctrl Pts',(518.2652421474,-9.15926477634836,11.4587676906409));
#88621=CARTESIAN_POINT('Ctrl Pts',(518.178681115507,-8.81491564491257,11.6178548673424));
#88622=CARTESIAN_POINT('Ctrl Pts',(518.117157287572,-8.47593534022153,11.7858549040992));
#88623=CARTESIAN_POINT('',(518.765685425361,-10.4227000320584,10.7873687265121));
#88624=CARTESIAN_POINT('Ctrl Pts',(518.482842712495,-9.81659693011828,11.1863055526149));
#88625=CARTESIAN_POINT('Ctrl Pts',(518.4835714073,-9.8186039782599,11.1855137512091));
#88626=CARTESIAN_POINT('Ctrl Pts',(518.484303140074,-9.82061430044638,11.1847150722895));
#88627=CARTESIAN_POINT('Ctrl Pts',(518.554092051407,-10.0118623131576,11.1082043938707));
#88628=CARTESIAN_POINT('Ctrl Pts',(518.652556551835,-10.2326240554321,10.9710191548411));
#88629=CARTESIAN_POINT('Ctrl Pts',(518.765685424949,-10.4227000306733,10.7873687278503));
#88630=CARTESIAN_POINT('',(521.036779393934,-12.5378078079164,8.23428050126071));
#88631=CARTESIAN_POINT('Ctrl Pts',(521.036779393919,-12.5378078078772,8.23428050121773));
#88632=CARTESIAN_POINT('Ctrl Pts',(520.89804042185,-12.4623887598882,8.34911622105974));
#88633=CARTESIAN_POINT('Ctrl Pts',(520.76436353255,-12.3839617118779,8.46507969614395));
#88634=CARTESIAN_POINT('Ctrl Pts',(519.890508026718,-11.8318905971298,9.25657548767299));
#88635=CARTESIAN_POINT('Ctrl Pts',(519.227527232995,-11.1986737462898,10.0376269256076));
#88636=CARTESIAN_POINT('Ctrl Pts',(518.76568542571,-10.4227000319511,10.7873687266157));
#88637=CARTESIAN_POINT('',(532.963220606066,-12.5378078079164,8.23428050126071));
#88638=CARTESIAN_POINT('Origin',(527.,-6.7,11.6047404107115));
#88639=CARTESIAN_POINT('',(535.234314574639,-10.4227000320585,10.7873687265119));
#88640=CARTESIAN_POINT('Ctrl Pts',(535.23431457429,-10.4227000319513,10.7873687266155));
#88641=CARTESIAN_POINT('Ctrl Pts',(534.772472767005,-11.1986737462899,10.0376269256075));
#88642=CARTESIAN_POINT('Ctrl Pts',(534.109491973282,-11.8318905971298,9.25657548767294));
#88643=CARTESIAN_POINT('Ctrl Pts',(533.23563646745,-12.3839617118779,8.46507969614396));
#88644=CARTESIAN_POINT('Ctrl Pts',(533.10195957815,-12.4623887598882,8.34911622105981));
#88645=CARTESIAN_POINT('Ctrl Pts',(532.963220606081,-12.5378078078771,8.23428050121781));
#88646=CARTESIAN_POINT('',(535.517157287515,-9.81659693012165,11.1863055526135));
#88647=CARTESIAN_POINT('Ctrl Pts',(535.234314575051,-10.4227000306734,10.7873687278502));
#88648=CARTESIAN_POINT('Ctrl Pts',(535.347921311572,-10.2318211626724,10.9717949056847));
#88649=CARTESIAN_POINT('Ctrl Pts',(535.447552756387,-10.0083090761463,11.110673113322));
#88650=CARTESIAN_POINT('Ctrl Pts',(535.517157287505,-9.81659693011858,11.1863055526147));
#88651=CARTESIAN_POINT('',(535.882842712451,-8.47593534022474,11.7858549040975));
#88652=CARTESIAN_POINT('Ctrl Pts',(535.882842712428,-8.47593534022145,11.7858549040992));
#88653=CARTESIAN_POINT('Ctrl Pts',(535.821318884493,-8.81491564491251,11.6178548673424));
#88654=CARTESIAN_POINT('Ctrl Pts',(535.7347578526,-9.1592647763483,11.4587676906408));
#88655=CARTESIAN_POINT('Ctrl Pts',(535.591041329177,-9.607053665426,11.2703872245611));
#88656=CARTESIAN_POINT('Ctrl Pts',(535.555140063964,-9.71198075829076,11.2275777225195));
#88657=CARTESIAN_POINT('Ctrl Pts',(535.517157287505,-9.81659693011864,11.1863055526147));
#88658=CARTESIAN_POINT('',(536.,-7.20000000000156,12.470765814495));
#88659=CARTESIAN_POINT('Ctrl Pts',(536.,-7.20000000000002,12.4707658144959));
#88660=CARTESIAN_POINT('Ctrl Pts',(536.,-7.20383835337878,12.4685497401394));
#88661=CARTESIAN_POINT('Ctrl Pts',(535.999996398286,-7.2076766662638,12.4663350887228));
#88662=CARTESIAN_POINT('Ctrl Pts',(535.999990317232,-7.2115163829872,12.4641210877021));
#88663=CARTESIAN_POINT('Ctrl Pts',(535.999323218915,-7.63273756686726,12.221242719787));
#88664=CARTESIAN_POINT('Ctrl Pts',(535.958538851494,-8.05886928393564,11.9925545613254));
#88665=CARTESIAN_POINT('Ctrl Pts',(535.88284271243,-8.47593534021115,11.7858549041042));
#88666=CARTESIAN_POINT('',(535.882842712451,-5.96888208215342,13.2333027775178));
#88667=CARTESIAN_POINT('Ctrl Pts',(535.88284271243,-5.96888208216602,13.2333027775093));
#88668=CARTESIAN_POINT('Ctrl Pts',(535.95853884256,-6.35642221867372,12.9754628367592));
#88669=CARTESIAN_POINT('Ctrl Pts',(535.999323210363,-6.76753777932651,12.7207660541882));
#88670=CARTESIAN_POINT('Ctrl Pts',(535.999990316982,-7.188487157105,12.4774170175749));
#88671=CARTESIAN_POINT('Ctrl Pts',(535.999996398191,-7.19232444631968,12.4751986970763));
#88672=CARTESIAN_POINT('Ctrl Pts',(536.,-7.19616159686892,12.4729819175769));
#88673=CARTESIAN_POINT('Ctrl Pts',(536.,-7.19999999999999,12.4707658144959));
#88674=CARTESIAN_POINT('Ctrl Pts',(535.517157287505,-4.77932631800001,14.0945750965023));
#88675=CARTESIAN_POINT('Ctrl Pts',(535.555140063964,-4.86737715152075,14.0246109190051));
#88676=CARTESIAN_POINT('Ctrl Pts',(535.591041329177,-4.95691481424451,13.9551461420599));
#88677=CARTESIAN_POINT('Ctrl Pts',(535.7347578526,-5.34395152798513,13.6615398216261));
#88678=CARTESIAN_POINT('Ctrl Pts',(535.821318884493,-5.65389963014295,13.4428683143823));
#88679=CARTESIAN_POINT('Ctrl Pts',(535.882842712428,-5.96888208215654,13.2333027775157));
#88680=CARTESIAN_POINT('Origin',(527.,-6.7,11.6047404107115));
#88681=CARTESIAN_POINT('',(518.482842712485,-4.77932631799753,14.0945750965044));
#88682=CARTESIAN_POINT('Ctrl Pts',(518.765685424949,-4.13078534297155,14.4200073665131));
#88683=CARTESIAN_POINT('Ctrl Pts',(518.65204849293,-4.38601035024533,14.3468950793686));
#88684=CARTESIAN_POINT('Ctrl Pts',(518.55242941068,-4.61801197111954,14.2227536173131));
#88685=CARTESIAN_POINT('Ctrl Pts',(518.482842712495,-4.7793263180001,14.0945750965024));
#88686=CARTESIAN_POINT('',(518.117157287549,-5.96888208215365,13.2333027775177));
#88687=CARTESIAN_POINT('Ctrl Pts',(518.117157287572,-5.96888208215675,13.2333027775156));
#88688=CARTESIAN_POINT('Ctrl Pts',(518.178681115507,-5.65389963014309,13.4428683143823));
#88689=CARTESIAN_POINT('Ctrl Pts',(518.2652421474,-5.34395152798522,13.6615398216261));
#88690=CARTESIAN_POINT('Ctrl Pts',(518.408958670823,-4.95691481424456,13.9551461420599));
#88691=CARTESIAN_POINT('Ctrl Pts',(518.444859936036,-4.86737715152084,14.0246109190052));
#88692=CARTESIAN_POINT('Ctrl Pts',(518.482842712495,-4.77932631800015,14.0945750965023));
#88693=CARTESIAN_POINT('Ctrl Pts',(518.,-7.20000000000001,12.470765814496));
#88694=CARTESIAN_POINT('Ctrl Pts',(518.,-7.19616161176896,12.4729819089744));
#88695=CARTESIAN_POINT('Ctrl Pts',(518.000003601789,-7.19232447611272,12.475198679864));
#88696=CARTESIAN_POINT('Ctrl Pts',(518.000009682939,-7.18848720178275,12.4774169917474));
#88697=CARTESIAN_POINT('Ctrl Pts',(518.000676785755,-6.76753780733218,12.7207660368554));
#88698=CARTESIAN_POINT('Ctrl Pts',(518.041461154763,-6.35642223237711,12.9754628276421));
#88699=CARTESIAN_POINT('Ctrl Pts',(518.11715728757,-5.96888208216625,13.2333027775093));
#88700=CARTESIAN_POINT('Origin',(527.,-13.75,23.8156986040721));
#88701=CARTESIAN_POINT('Origin',(527.,-6.7,11.6047404107115));
#88702=CARTESIAN_POINT('Origin',(527.,-6.5,11.2583302491977));
#88703=CARTESIAN_POINT('Origin',(527.,-6.5,11.2583302491977));
#88704=CARTESIAN_POINT('Origin',(527.,-6.7,11.6047404107115));
#88705=CARTESIAN_POINT('',(522.762075979917,-12.9807406984079,7.51667286242377));
#88706=CARTESIAN_POINT('Ctrl Pts',(522.762075979917,-12.9807406984079,7.51667286242377));
#88707=CARTESIAN_POINT('Ctrl Pts',(522.758255200061,-12.9807406984079,7.51667286242377));
#88708=CARTESIAN_POINT('Ctrl Pts',(522.754457930714,-12.9807273446463,7.51669592348406));
#88709=CARTESIAN_POINT('Ctrl Pts',(522.64018487178,-12.9799558911659,7.51802815100091));
#88710=CARTESIAN_POINT('Ctrl Pts',(522.49912720191,-12.9685157360108,7.53788670849498));
#88711=CARTESIAN_POINT('Ctrl Pts',(522.130810325905,-12.914660507337,7.62988795088002));
#88712=CARTESIAN_POINT('Ctrl Pts',(521.891687872103,-12.864104887125,7.71591973222724));
#88713=CARTESIAN_POINT('Ctrl Pts',(521.428177636548,-12.7208525920888,7.94965142708));
#88714=CARTESIAN_POINT('Ctrl Pts',(521.218157792946,-12.636405815183,8.08415167507323));
#88715=CARTESIAN_POINT('Ctrl Pts',(521.03677939365,-12.5378078077306,8.23428050144093));
#88716=CARTESIAN_POINT('',(531.237924020083,-12.9807406984079,7.51667286242377));
#88717=CARTESIAN_POINT('Origin',(527.,-6.5,11.2583302491977));
#88718=CARTESIAN_POINT('Ctrl Pts',(532.96322060635,-12.5378078077306,8.23428050144094));
#88719=CARTESIAN_POINT('Ctrl Pts',(532.699729877775,-12.6810423986217,8.01618642853462));
#88720=CARTESIAN_POINT('Ctrl Pts',(532.366534064584,-12.7988564878116,7.82390390690329));
#88721=CARTESIAN_POINT('Ctrl Pts',(531.791717805958,-12.9296312139358,7.60490233717503));
#88722=CARTESIAN_POINT('Ctrl Pts',(531.578769165016,-12.9609143600255,7.55085197344993));
#88723=CARTESIAN_POINT('Ctrl Pts',(531.344918498116,-12.9784056012462,7.52070938305816));
#88724=CARTESIAN_POINT('Ctrl Pts',(531.288493822179,-12.9807406984079,7.51667286242377));
#88725=CARTESIAN_POINT('Ctrl Pts',(531.237924020083,-12.9807406984079,7.51667286242377));
#88726=CARTESIAN_POINT('Origin',(527.,-6.5,11.2583302491977));
#88727=CARTESIAN_POINT('',(527.,-12.9807406984079,7.51667286242377));
#88728=CARTESIAN_POINT('Origin',(527.,-13.55,-23.4692884425583));
#88729=CARTESIAN_POINT('',(535.6,-13.75,-23.8156986040721));
#88730=CARTESIAN_POINT('Origin',(527.,-13.75,-23.8156986040721));
#88731=CARTESIAN_POINT('',(536.,-13.55,-23.4692884425583));
#88732=CARTESIAN_POINT('Origin',(535.6,-13.55,-23.4692884425583));
#88733=CARTESIAN_POINT('',(518.,-13.55,-23.4692884425583));
#88734=CARTESIAN_POINT('Origin',(527.,-13.55,-23.4692884425583));
#88735=CARTESIAN_POINT('Origin',(527.,-13.55,-23.4692884425583));
#88736=CARTESIAN_POINT('Origin',(527.,-6.50000000000001,-11.2583302491977));
#88737=CARTESIAN_POINT('',(518.,-7.19999999999891,-12.4707658144965));
#88738=CARTESIAN_POINT('',(518.,-6.5,-11.2583302491977));
#88739=CARTESIAN_POINT('',(518.117157287549,-5.9688820821539,-13.2333027775175));
#88740=CARTESIAN_POINT('Ctrl Pts',(518.11715728757,-5.96888208216648,-13.2333027775091));
#88741=CARTESIAN_POINT('Ctrl Pts',(518.041432655893,-6.35656813753687,-12.9753657533672));
#88742=CARTESIAN_POINT('Ctrl Pts',(518.000677557365,-6.76744956600244,-12.7208173836523));
#88743=CARTESIAN_POINT('Ctrl Pts',(518.00000968508,-7.18848724210988,-12.4774169695489));
#88744=CARTESIAN_POINT('Ctrl Pts',(518.000003599129,-7.19232392599177,-12.4751989959597));
#88745=CARTESIAN_POINT('Ctrl Pts',(518.,-7.19616156249294,-12.472981937424));
#88746=CARTESIAN_POINT('Ctrl Pts',(518.,-7.20000000000004,-12.470765814496));
#88747=CARTESIAN_POINT('',(518.482842712485,-4.77932631799762,-14.0945750965043));
#88748=CARTESIAN_POINT('Ctrl Pts',(518.482842712495,-4.7793263180002,-14.0945750965023));
#88749=CARTESIAN_POINT('Ctrl Pts',(518.444859936036,-4.86737715152089,-14.0246109190051));
#88750=CARTESIAN_POINT('Ctrl Pts',(518.408958670823,-4.95691481424459,-13.9551461420599));
#88751=CARTESIAN_POINT('Ctrl Pts',(518.2652421474,-5.3439515279853,-13.661539821626));
#88752=CARTESIAN_POINT('Ctrl Pts',(518.178681115507,-5.65389963014324,-13.4428683143822));
#88753=CARTESIAN_POINT('Ctrl Pts',(518.117157287572,-5.96888208215698,-13.2333027775155));
#88754=CARTESIAN_POINT('',(518.765685425361,-4.13078534112017,-14.4200073670434));
#88755=CARTESIAN_POINT('Ctrl Pts',(518.482842712495,-4.77932631800019,-14.0945750965023));
#88756=CARTESIAN_POINT('Ctrl Pts',(518.484732409107,-4.77494566505047,-14.0980559128472));
#88757=CARTESIAN_POINT('Ctrl Pts',(518.486643571927,-4.77051154796919,-14.1015345793544));
#88758=CARTESIAN_POINT('Ctrl Pts',(518.557423568513,-4.60618275816552,-14.2288316588688));
#88759=CARTESIAN_POINT('Ctrl Pts',(518.654514417981,-4.38047195944378,-14.3484816183325));
#88760=CARTESIAN_POINT('Ctrl Pts',(518.765685424949,-4.13078534297155,-14.4200073665131));
#88761=CARTESIAN_POINT('',(521.036779393934,-0.86219219202042,-14.9752003200529));
#88762=CARTESIAN_POINT('Ctrl Pts',(521.036779393919,-0.862192192002859,
-14.9752003199974));
#88763=CARTESIAN_POINT('Ctrl Pts',(520.89804042185,-0.999352366642366,-14.9673033684307));
#88764=CARTESIAN_POINT('Ctrl Pts',(520.76436353255,-1.13899320598156,-14.9573652900521));
#88765=CARTESIAN_POINT('Ctrl Pts',(519.890508026718,-2.10048422580825,-14.8750055757491));
#88766=CARTESIAN_POINT('Ctrl Pts',(519.227527232995,-3.09350303814205,-14.7171494157846));
#88767=CARTESIAN_POINT('Ctrl Pts',(518.76568542571,-4.13078534126348,-14.4200073670024));
#88768=CARTESIAN_POINT('',(532.963220606066,-0.862192192020421,-14.9752003200529));
#88769=CARTESIAN_POINT('Origin',(527.,-6.70000000000001,-11.6047404107115));
#88770=CARTESIAN_POINT('',(535.234314574639,-4.13078534111982,-14.4200073670435));
#88771=CARTESIAN_POINT('Ctrl Pts',(535.23431457429,-4.13078534126319,-14.4200073670025));
#88772=CARTESIAN_POINT('Ctrl Pts',(534.772472767005,-3.09350303814179,-14.7171494157847));
#88773=CARTESIAN_POINT('Ctrl Pts',(534.109491973282,-2.10048422580818,-14.8750055757491));
#88774=CARTESIAN_POINT('Ctrl Pts',(533.23563646745,-1.13899320598156,-14.9573652900521));
#88775=CARTESIAN_POINT('Ctrl Pts',(533.10195957815,-0.999352366642402,-14.9673033684307));
#88776=CARTESIAN_POINT('Ctrl Pts',(532.963220606081,-0.862192192002894,
-14.9752003199974));
#88777=CARTESIAN_POINT('',(535.517157287515,-4.77932631799747,-14.0945750965044));
#88778=CARTESIAN_POINT('Ctrl Pts',(535.234314575051,-4.1307853429714,-14.4200073665131));
#88779=CARTESIAN_POINT('Ctrl Pts',(535.347951507068,-4.38601035024165,-14.3468950793696));
#88780=CARTESIAN_POINT('Ctrl Pts',(535.447570589319,-4.61801197111726,-14.2227536173149));
#88781=CARTESIAN_POINT('Ctrl Pts',(535.517157287505,-4.77932631800005,-14.0945750965023));
#88782=CARTESIAN_POINT('',(535.882842712451,-5.96888208215344,-13.2333027775177));
#88783=CARTESIAN_POINT('Ctrl Pts',(535.882842712428,-5.96888208215652,-13.2333027775157));
#88784=CARTESIAN_POINT('Ctrl Pts',(535.821318884493,-5.65389963014293,-13.4428683143823));
#88785=CARTESIAN_POINT('Ctrl Pts',(535.7347578526,-5.34395152798514,-13.6615398216261));
#88786=CARTESIAN_POINT('Ctrl Pts',(535.591041329177,-4.95691481424452,-13.9551461420598));
#88787=CARTESIAN_POINT('Ctrl Pts',(535.555140063964,-4.86737715152078,-14.0246109190051));
#88788=CARTESIAN_POINT('Ctrl Pts',(535.517157287505,-4.77932631800004,-14.0945750965023));
#88789=CARTESIAN_POINT('',(536.,-7.19999999999891,-12.4707658144965));
#88790=CARTESIAN_POINT('Ctrl Pts',(536.,-7.20000000000001,-12.4707658144959));
#88791=CARTESIAN_POINT('Ctrl Pts',(536.,-7.19616164662126,-12.4729818888524));
#88792=CARTESIAN_POINT('Ctrl Pts',(535.99999639828,-7.19232454578702,-12.4751986396123));
#88793=CARTESIAN_POINT('Ctrl Pts',(535.999990317235,-7.18848730628792,-12.4774169313338));
#88794=CARTESIAN_POINT('Ctrl Pts',(535.99932321985,-6.76753787666126,-12.7207659938898));
#88795=CARTESIAN_POINT('Ctrl Pts',(535.958538851494,-6.35642226441092,-12.9754628063291));
#88796=CARTESIAN_POINT('Ctrl Pts',(535.88284271243,-5.96888208216602,-13.2333027775093));
#88797=CARTESIAN_POINT('',(535.882842712451,-8.47593534022476,-11.7858549040975));
#88798=CARTESIAN_POINT('Ctrl Pts',(535.88284271243,-8.47593534021119,-11.7858549041042));
#88799=CARTESIAN_POINT('Ctrl Pts',(535.95853884256,-8.05886933315747,-11.9925545369309));
#88800=CARTESIAN_POINT('Ctrl Pts',(535.999323209414,-7.6327376674167,-12.2212426658364));
#88801=CARTESIAN_POINT('Ctrl Pts',(535.999990316979,-7.21151653228314,-12.4641210016164));
#88802=CARTESIAN_POINT('Ctrl Pts',(535.999996398197,-7.2076767657835,-12.4663350313016));
#88803=CARTESIAN_POINT('Ctrl Pts',(536.,-7.20383840313102,-12.468549711415));
#88804=CARTESIAN_POINT('Ctrl Pts',(536.,-7.20000000000001,-12.4707658144959));
#88805=CARTESIAN_POINT('',(535.517157287515,-9.81659693012166,-11.1863055526135));
#88806=CARTESIAN_POINT('Ctrl Pts',(535.517157287505,-9.8165969301186,-11.1863055526147));
#88807=CARTESIAN_POINT('Ctrl Pts',(535.555140063964,-9.71198075829077,-11.2275777225195));
#88808=CARTESIAN_POINT('Ctrl Pts',(535.591041329177,-9.60705366542601,-11.2703872245611));
#88809=CARTESIAN_POINT('Ctrl Pts',(535.7347578526,-9.15926477634832,-11.4587676906408));
#88810=CARTESIAN_POINT('Ctrl Pts',(535.821318884493,-8.81491564491253,-11.6178548673424));
#88811=CARTESIAN_POINT('Ctrl Pts',(535.882842712428,-8.47593534022146,-11.7858549040992));
#88812=CARTESIAN_POINT('',(535.234314574639,-10.4227000320585,-10.787368726512));
#88813=CARTESIAN_POINT('Ctrl Pts',(535.517157287505,-9.81659693011848,-11.1863055526148));
#88814=CARTESIAN_POINT('Ctrl Pts',(535.5164285927,-9.81860397826011,-11.185513751209));
#88815=CARTESIAN_POINT('Ctrl Pts',(535.515696859926,-9.82061430044658,-11.1847150722893));
#88816=CARTESIAN_POINT('Ctrl Pts',(535.445907948593,-10.0118623131575,-11.1082043938707));
#88817=CARTESIAN_POINT('Ctrl Pts',(535.347443448165,-10.232624055432,-10.9710191548412));
#88818=CARTESIAN_POINT('Ctrl Pts',(535.234314575051,-10.4227000306734,-10.7873687278502));
#88819=CARTESIAN_POINT('',(532.963220606066,-12.5378078079164,-8.2342805012607));
#88820=CARTESIAN_POINT('Ctrl Pts',(532.963220606081,-12.5378078078772,-8.23428050121772));
#88821=CARTESIAN_POINT('Ctrl Pts',(533.101959573956,-12.4623887621683,-8.34911621758802));
#88822=CARTESIAN_POINT('Ctrl Pts',(533.235636462502,-12.3839617150039,-8.46507969166234));
#88823=CARTESIAN_POINT('Ctrl Pts',(534.109491973282,-11.8318905971298,-9.25657548767295));
#88824=CARTESIAN_POINT('Ctrl Pts',(534.772472767005,-11.1986737462899,-10.0376269256075));
#88825=CARTESIAN_POINT('Ctrl Pts',(535.23431457429,-10.4227000319513,-10.7873687266156));
#88826=CARTESIAN_POINT('',(521.036779393934,-12.5378078079164,-8.2342805012607));
#88827=CARTESIAN_POINT('Origin',(527.,-6.70000000000001,-11.6047404107115));
#88828=CARTESIAN_POINT('',(518.765685425361,-10.4227000320584,-10.7873687265121));
#88829=CARTESIAN_POINT('Ctrl Pts',(518.76568542571,-10.4227000319511,-10.7873687266157));
#88830=CARTESIAN_POINT('Ctrl Pts',(519.227527232995,-11.1986737462898,-10.0376269256076));
#88831=CARTESIAN_POINT('Ctrl Pts',(519.890508026718,-11.8318905971298,-9.25657548767298));
#88832=CARTESIAN_POINT('Ctrl Pts',(520.76436353255,-12.3839617118779,-8.46507969614394));
#88833=CARTESIAN_POINT('Ctrl Pts',(520.89804042185,-12.4623887598882,-8.34911622105977));
#88834=CARTESIAN_POINT('Ctrl Pts',(521.036779393919,-12.5378078078771,-8.23428050121775));
#88835=CARTESIAN_POINT('',(518.482842712485,-9.81659693012145,-11.1863055526136));
#88836=CARTESIAN_POINT('Ctrl Pts',(518.765685424949,-10.4227000306733,-10.7873687278503));
#88837=CARTESIAN_POINT('Ctrl Pts',(518.652078688429,-10.2318211626746,-10.9717949056826));
#88838=CARTESIAN_POINT('Ctrl Pts',(518.552447243613,-10.0083090761484,-11.1106731133212));
#88839=CARTESIAN_POINT('Ctrl Pts',(518.482842712495,-9.81659693011839,-11.1863055526149));
#88840=CARTESIAN_POINT('',(518.117157287549,-8.47593534022466,-11.7858549040977));
#88841=CARTESIAN_POINT('Ctrl Pts',(518.117157287572,-8.47593534022136,-11.7858549040993));
#88842=CARTESIAN_POINT('Ctrl Pts',(518.178681115507,-8.81491564491246,-11.6178548673425));
#88843=CARTESIAN_POINT('Ctrl Pts',(518.2652421474,-9.1592647763483,-11.4587676906409));
#88844=CARTESIAN_POINT('Ctrl Pts',(518.408958670823,-9.60705366542596,-11.2703872245612));
#88845=CARTESIAN_POINT('Ctrl Pts',(518.444859936036,-9.7119807582906,-11.2275777225196));
#88846=CARTESIAN_POINT('Ctrl Pts',(518.482842712495,-9.81659693011839,-11.1863055526149));
#88847=CARTESIAN_POINT('Ctrl Pts',(518.,-7.20000000000004,-12.470765814496));
#88848=CARTESIAN_POINT('Ctrl Pts',(518.,-7.20383838823105,-12.4685497200175));
#88849=CARTESIAN_POINT('Ctrl Pts',(518.000003601783,-7.20767673596133,-12.4663350485081));
#88850=CARTESIAN_POINT('Ctrl Pts',(518.000009682942,-7.21151648755889,-12.4641210274051));
#88851=CARTESIAN_POINT('Ctrl Pts',(518.000676786757,-7.63273763852262,-12.2212426813519));
#88852=CARTESIAN_POINT('Ctrl Pts',(518.041461154763,-8.05886931841019,-11.9925545442398));
#88853=CARTESIAN_POINT('Ctrl Pts',(518.11715728757,-8.47593534021109,-11.7858549041044));
#88854=CARTESIAN_POINT('Origin',(527.,-13.75,-23.8156986040721));
#88855=CARTESIAN_POINT('Origin',(527.,-6.70000000000001,-11.6047404107115));
#88856=CARTESIAN_POINT('',(522.762075979917,-0.0192593015921494,-14.9999876359716));
#88857=CARTESIAN_POINT('Ctrl Pts',(522.762075979917,-0.0192593015921408,
-14.9999876359716));
#88858=CARTESIAN_POINT('Ctrl Pts',(522.758255200061,-0.0192593015921405,
-14.9999876359716));
#88859=CARTESIAN_POINT('Ctrl Pts',(522.754457930714,-0.0192859499369469,
-14.9999876018051));
#88860=CARTESIAN_POINT('Ctrl Pts',(522.640184871779,-0.0208254195503758,
-14.9999856172516));
#88861=CARTESIAN_POINT('Ctrl Pts',(522.499127201909,-0.04374351240062,-15.0000074310111));
#88862=CARTESIAN_POINT('Ctrl Pts',(522.130810325905,-0.150346539822266,
-14.9993680560455));
#88863=CARTESIAN_POINT('Ctrl Pts',(521.891687872104,-0.250130058107573,
-14.9986014953114));
#88864=CARTESIAN_POINT('Ctrl Pts',(521.428177636548,-0.524173791038048,
-14.991407216086));
#88865=CARTESIAN_POINT('Ctrl Pts',(521.218157792946,-0.682877811068399,
-14.9855242860145));
#88866=CARTESIAN_POINT('Ctrl Pts',(521.03677939365,-0.862192192269424,-14.975200319982));
#88867=CARTESIAN_POINT('',(531.237924020083,-0.0192593015921494,-14.9999876359716));
#88868=CARTESIAN_POINT('Origin',(527.,-6.50000000000001,-11.2583302491977));
#88869=CARTESIAN_POINT('Ctrl Pts',(532.96322060635,-0.86219219226947,-14.975200319982));
#88870=CARTESIAN_POINT('Ctrl Pts',(532.699729877774,-0.601699889270847,
-14.9901980779414));
#88871=CARTESIAN_POINT('Ctrl Pts',(532.366534064582,-0.376271296239959,
-14.9960868112878));
#88872=CARTESIAN_POINT('Ctrl Pts',(531.791717805957,-0.121223010324898,
-14.9998402614201));
#88873=CARTESIAN_POINT('Ctrl Pts',(531.578769165015,-0.0587724492106223,
-14.9999070787816));
#88874=CARTESIAN_POINT('Ctrl Pts',(531.344918498116,-0.0239225795852008,
-14.9999836428266));
#88875=CARTESIAN_POINT('Ctrl Pts',(531.288493822179,-0.0192593015921421,
-14.9999876359716));
#88876=CARTESIAN_POINT('Ctrl Pts',(531.237924020083,-0.0192593015921448,
-14.9999876359716));
#88877=CARTESIAN_POINT('Origin',(527.,-6.50000000000001,-11.2583302491977));
#88878=CARTESIAN_POINT('',(527.,-0.0192593015921494,-14.9999876359716));
#88879=CARTESIAN_POINT('Origin',(527.,-6.70000000000001,-11.6047404107115));
#88880=CARTESIAN_POINT('',(531.237924020083,-12.9807406984079,-7.51667286242375));
#88881=CARTESIAN_POINT('Ctrl Pts',(531.237924020083,-12.9807406984079,-7.51667286242375));
#88882=CARTESIAN_POINT('Ctrl Pts',(531.241744799939,-12.9807406984079,-7.51667286242375));
#88883=CARTESIAN_POINT('Ctrl Pts',(531.245542069285,-12.9807273446464,-7.51669592348404));
#88884=CARTESIAN_POINT('Ctrl Pts',(531.359815128221,-12.979955891166,-7.51802815100086));
#88885=CARTESIAN_POINT('Ctrl Pts',(531.500872798091,-12.9685157360107,-7.53788670849509));
#88886=CARTESIAN_POINT('Ctrl Pts',(531.869189674096,-12.914660507337,-7.62988795088001));
#88887=CARTESIAN_POINT('Ctrl Pts',(532.108312127897,-12.8641048871248,-7.71591973222749));
#88888=CARTESIAN_POINT('Ctrl Pts',(532.571822363451,-12.7208525920891,-7.94965142707956));
#88889=CARTESIAN_POINT('Ctrl Pts',(532.781842207053,-12.6364058151837,-8.08415167507281));
#88890=CARTESIAN_POINT('Ctrl Pts',(532.963220606349,-12.5378078077313,-8.23428050144051));
#88891=CARTESIAN_POINT('',(522.762075979917,-12.9807406984079,-7.51667286242375));
#88892=CARTESIAN_POINT('Origin',(527.,-6.50000000000001,-11.2583302491977));
#88893=CARTESIAN_POINT('Ctrl Pts',(521.036779393651,-12.537807807731,-8.23428050144024));
#88894=CARTESIAN_POINT('Ctrl Pts',(521.300270122226,-12.6810423986223,-8.0161864285338));
#88895=CARTESIAN_POINT('Ctrl Pts',(521.633465935417,-12.7988564878118,-7.82390390690293));
#88896=CARTESIAN_POINT('Ctrl Pts',(522.208282194043,-12.929631213936,-7.6049023371746));
#88897=CARTESIAN_POINT('Ctrl Pts',(522.421230834985,-12.9609143600256,-7.5508519734498));
#88898=CARTESIAN_POINT('Ctrl Pts',(522.655081501884,-12.9784056012462,-7.52070938305814));
#88899=CARTESIAN_POINT('Ctrl Pts',(522.711506177821,-12.9807406984079,-7.51667286242375));
#88900=CARTESIAN_POINT('Ctrl Pts',(522.762075979917,-12.9807406984079,-7.51667286242375));
#88901=CARTESIAN_POINT('Origin',(527.,-6.50000000000001,-11.2583302491977));
#88902=CARTESIAN_POINT('',(527.,-12.9807406984079,-7.51667286242375));
#88903=CARTESIAN_POINT('Origin',(518.,11.5,0.3));
#88904=CARTESIAN_POINT('',(536.,11.1,0.3));
#88905=CARTESIAN_POINT('',(536.,11.5,0.7));
#88906=CARTESIAN_POINT('Origin',(536.,11.5,0.3));
#88907=CARTESIAN_POINT('',(518.,11.5,0.7));
#88908=CARTESIAN_POINT('',(518.,11.5,0.7));
#88909=CARTESIAN_POINT('',(518.,11.1,0.3));
#88910=CARTESIAN_POINT('Origin',(518.,11.5,0.3));
#88911=CARTESIAN_POINT('',(518.,11.1,0.3));
#88912=CARTESIAN_POINT('Origin',(518.,12.4,0.7));
#88913=CARTESIAN_POINT('',(536.,11.9795659353751,0.7));
#88914=CARTESIAN_POINT('',(536.,12.4,0.7));
#88915=CARTESIAN_POINT('',(518.,11.9795659353751,0.7));
#88916=CARTESIAN_POINT('',(527.,11.9795659353751,0.7));
#88917=CARTESIAN_POINT('',(518.,12.4,0.7));
#88918=CARTESIAN_POINT('Origin',(536.,12.,0.));
#88919=CARTESIAN_POINT('',(536.,-8.31079580944086,11.5562270847921));
#88920=CARTESIAN_POINT('Ctrl Pts',(536.,-8.31079580944085,11.5562270847921));
#88921=CARTESIAN_POINT('Ctrl Pts',(536.,-7.9249330284473,11.8337248147531));
#88922=CARTESIAN_POINT('Ctrl Pts',(536.000000000004,-7.56211366310163,12.1432120305888));
#88923=CARTESIAN_POINT('Ctrl Pts',(536.,-7.20642267737424,12.4649492081416));
#88924=CARTESIAN_POINT('Ctrl Pts',(536.,-7.20321107037281,12.4678572228852));
#88925=CARTESIAN_POINT('Ctrl Pts',(536.,-7.20000000000002,12.4707658144959));
#88926=CARTESIAN_POINT('',(536.,-8.31079580944088,-11.5562270847921));
#88927=CARTESIAN_POINT('Origin',(536.,0.,0.));
#88928=CARTESIAN_POINT('Ctrl Pts',(536.,-7.2,-12.4707658144959));
#88929=CARTESIAN_POINT('Ctrl Pts',(536.,-7.20321111198339,-12.4678571851766));
#88930=CARTESIAN_POINT('Ctrl Pts',(536.,-7.20642276063924,-12.4649491327435));
#88931=CARTESIAN_POINT('Ctrl Pts',(536.000000000003,-7.56211374877667,-12.1432119579598));
#88932=CARTESIAN_POINT('Ctrl Pts',(536.,-7.92493307398652,-11.833724782003));
#88933=CARTESIAN_POINT('Ctrl Pts',(536.,-8.31079580944087,-11.5562270847921));
#88934=CARTESIAN_POINT('',(536.,-5.85258832261126,-12.9754738390371));
#88935=CARTESIAN_POINT('Ctrl Pts',(536.,-5.85258832261122,-12.9754738390371));
#88936=CARTESIAN_POINT('Ctrl Pts',(536.,-6.28583979674674,-12.7800557333022));
#88937=CARTESIAN_POINT('Ctrl Pts',(535.999999999986,-6.73527327116365,-12.6205885550169));
#88938=CARTESIAN_POINT('Ctrl Pts',(536.,-7.19175133243048,-12.4734197130817));
#88939=CARTESIAN_POINT('Ctrl Pts',(536.,-7.19587555058959,-12.4720923872068));
#88940=CARTESIAN_POINT('Ctrl Pts',(536.,-7.20000000000006,-12.4707658144959));
#88941=CARTESIAN_POINT('',(536.,14.1633841320522,-1.419246754245));
#88942=CARTESIAN_POINT('Origin',(536.,0.,0.));
#88943=CARTESIAN_POINT('Ctrl Pts',(536.,14.4,-4.71844785465692E-15));
#88944=CARTESIAN_POINT('Ctrl Pts',(536.,14.3990866091107,-0.00423521921160987));
#88945=CARTESIAN_POINT('Ctrl Pts',(536.,14.3981739862025,-0.00847061475408605));
#88946=CARTESIAN_POINT('Ctrl Pts',(536.000000000003,14.297386906149,-0.477376632577604));
#88947=CARTESIAN_POINT('Ctrl Pts',(536.,14.2107728196014,-0.946330974362331));
#88948=CARTESIAN_POINT('Ctrl Pts',(536.,14.1633841320521,-1.41924675424501));
#88949=CARTESIAN_POINT('',(536.,14.1633841320521,1.41924675424547));
#88950=CARTESIAN_POINT('Ctrl Pts',(536.,14.1633841320521,1.41924675424546));
#88951=CARTESIAN_POINT('Ctrl Pts',(536.,14.210772825194,0.946330918549924));
#88952=CARTESIAN_POINT('Ctrl Pts',(535.999999999999,14.2973869261308,0.4773765220558));
#88953=CARTESIAN_POINT('Ctrl Pts',(536.,14.3981740098758,0.00847050495900394));
#88954=CARTESIAN_POINT('Ctrl Pts',(536.,14.3990866209829,0.00423516432177781));
#88955=CARTESIAN_POINT('Ctrl Pts',(536.,14.4,-7.49400541621981E-15));
#88956=CARTESIAN_POINT('',(536.,-5.85258832261124,12.9754738390372));
#88957=CARTESIAN_POINT('Origin',(536.,0.,0.));
#88958=CARTESIAN_POINT('Ctrl Pts',(536.,-7.2,12.4707658144959));
#88959=CARTESIAN_POINT('Ctrl Pts',(536.,-7.1958754971275,12.472092404388));
#88960=CARTESIAN_POINT('Ctrl Pts',(536.,-7.19175122552344,12.4734197474849));
#88961=CARTESIAN_POINT('Ctrl Pts',(536.,-6.73527316506757,12.6205885930199));
#88962=CARTESIAN_POINT('Ctrl Pts',(536.,-6.28583974561473,12.7800557563653));
#88963=CARTESIAN_POINT('Ctrl Pts',(536.,-5.8525883226112,12.9754738390371));
#88964=CARTESIAN_POINT('',(536.,11.1,-0.3));
#88965=CARTESIAN_POINT('',(536.,11.1,0.7));
#88966=CARTESIAN_POINT('',(536.,11.5,-0.7));
#88967=CARTESIAN_POINT('Origin',(536.,11.5,-0.3));
#88968=CARTESIAN_POINT('',(536.,11.9795659353751,-0.7));
#88969=CARTESIAN_POINT('',(536.,11.1,-0.7));
#88970=CARTESIAN_POINT('',(536.,11.7525454562834,-2.42439173773414));
#88971=CARTESIAN_POINT('Origin',(536.,0.,0.));
#88972=CARTESIAN_POINT('',(536.,11.289320333896,-2.30027094027665));
#88973=CARTESIAN_POINT('',(536.,12.1586535775562,-2.53320808086892));
#88974=CARTESIAN_POINT('',(536.,10.7994223853394,-2.58311365275127));
#88975=CARTESIAN_POINT('Origin',(536.,11.185792715855,-2.68664127079228));
#88976=CARTESIAN_POINT('',(536.,10.6441309582779,-3.16266914852471));
#88977=CARTESIAN_POINT('',(536.,10.9029500033804,-2.19674332223564));
#88978=CARTESIAN_POINT('',(536.,10.9269736707525,-3.65256709708134));
#88979=CARTESIAN_POINT('Origin',(536.,11.0305012887935,-3.26619676656572));
#88980=CARTESIAN_POINT('',(536.,11.3901987931398,-3.77668789453883));
#88981=CARTESIAN_POINT('',(536.,10.5406033402369,-3.54903947904034));
#88982=CARTESIAN_POINT('',(536.,10.7246084263455,-5.38356518503846));
#88983=CARTESIAN_POINT('Origin',(536.,0.,0.));
#88984=CARTESIAN_POINT('',(536.,10.309292143521,-5.1437822173509));
#88985=CARTESIAN_POINT('',(536.,11.088715006927,-5.5937822173509));
#88986=CARTESIAN_POINT('',(536.,9.76288198200726,-5.29019237886467));
#88987=CARTESIAN_POINT('Origin',(536.,10.109292143521,-5.49019237886467));
#88988=CARTESIAN_POINT('',(536.,9.46288198200726,-5.80980762113534));
#88989=CARTESIAN_POINT('',(536.,9.96288198200727,-4.9437822173509));
#88990=CARTESIAN_POINT('',(536.,9.60929214352104,-6.35621778264911));
#88991=CARTESIAN_POINT('Origin',(536.,9.80929214352104,-6.00980762113534));
#88992=CARTESIAN_POINT('',(536.,10.0246084263455,-6.59600075033667));
#88993=CARTESIAN_POINT('',(536.,9.26288198200726,-6.15621778264911));
#88994=CARTESIAN_POINT('',(536.,8.96580705540569,-7.97585756174453));
#88995=CARTESIAN_POINT('Origin',(536.,0.,0.));
#88996=CARTESIAN_POINT('',(536.,8.62670273047588,-7.63675323681471));
#88997=CARTESIAN_POINT('',(536.,9.26309883354377,-8.27314933988261));
#88998=CARTESIAN_POINT('',(536.,8.06101730552664,-7.63675323681472));
#88999=CARTESIAN_POINT('Origin',(536.,8.34386001800126,-7.91959594928933));
#89000=CARTESIAN_POINT('',(536.,7.63675323681471,-8.06101730552664));
#89001=CARTESIAN_POINT('',(536.,8.34386001800126,-7.35391052434009));
#89002=CARTESIAN_POINT('',(536.,7.63675323681471,-8.62670273047588));
#89003=CARTESIAN_POINT('Origin',(536.,7.91959594928933,-8.34386001800126));
#89004=CARTESIAN_POINT('',(536.,7.97585756174453,-8.9658070554057));
#89005=CARTESIAN_POINT('',(536.,7.35391052434009,-8.34386001800126));
#89006=CARTESIAN_POINT('',(536.,6.59600075033666,-10.0246084263456));
#89007=CARTESIAN_POINT('Origin',(536.,0.,0.));
#89008=CARTESIAN_POINT('',(536.,6.3562177826491,-9.60929214352105));
#89009=CARTESIAN_POINT('',(536.,6.8062177826491,-10.388715006927));
#89010=CARTESIAN_POINT('',(536.,5.80980762113532,-9.46288198200727));
#89011=CARTESIAN_POINT('Origin',(536.,6.00980762113532,-9.80929214352105));
#89012=CARTESIAN_POINT('',(536.,5.29019237886466,-9.76288198200727));
#89013=CARTESIAN_POINT('',(536.,6.1562177826491,-9.26288198200727));
#89014=CARTESIAN_POINT('',(536.,5.14378221735088,-10.309292143521));
#89015=CARTESIAN_POINT('Origin',(536.,5.49019237886466,-10.109292143521));
#89016=CARTESIAN_POINT('',(536.,5.38356518503845,-10.7246084263456));
#89017=CARTESIAN_POINT('',(536.,4.94378221735088,-9.96288198200727));
#89018=CARTESIAN_POINT('',(536.,3.77668789453882,-11.3901987931398));
#89019=CARTESIAN_POINT('Origin',(536.,0.,0.));
#89020=CARTESIAN_POINT('',(536.,3.65256709708133,-10.9269736707525));
#89021=CARTESIAN_POINT('',(536.,3.8855042376736,-11.7963069144127));
#89022=CARTESIAN_POINT('',(536.,3.1626691485247,-10.6441309582779));
#89023=CARTESIAN_POINT('Origin',(536.,3.2661967665657,-11.0305012887935));
#89024=CARTESIAN_POINT('',(536.,2.58311365275125,-10.7994223853394));
#89025=CARTESIAN_POINT('',(536.,3.54903947904032,-10.5406033402369));
#89026=CARTESIAN_POINT('',(536.,2.30027094027664,-11.2893203338961));
#89027=CARTESIAN_POINT('Origin',(536.,2.68664127079226,-11.185792715855));
#89028=CARTESIAN_POINT('',(536.,2.42439173773412,-11.7525454562834));
#89029=CARTESIAN_POINT('',(536.,2.19674332223563,-10.9029500033804));
#89030=CARTESIAN_POINT('',(536.,0.699999999999998,-11.9795659353751));
#89031=CARTESIAN_POINT('Origin',(536.,0.,0.));
#89032=CARTESIAN_POINT('',(536.,0.699999999999998,-11.5));
#89033=CARTESIAN_POINT('',(536.,0.699999999999998,-12.4));
#89034=CARTESIAN_POINT('',(536.,0.299999999999998,-11.1));
#89035=CARTESIAN_POINT('Origin',(536.,0.299999999999998,-11.5));
#89036=CARTESIAN_POINT('',(536.,-0.300000000000002,-11.1));
#89037=CARTESIAN_POINT('',(536.,0.699999999999998,-11.1));
#89038=CARTESIAN_POINT('',(536.,-0.700000000000002,-11.5));
#89039=CARTESIAN_POINT('Origin',(536.,-0.300000000000002,-11.5));
#89040=CARTESIAN_POINT('',(536.,-0.700000000000002,-11.9795659353751));
#89041=CARTESIAN_POINT('',(536.,-0.700000000000002,-11.1));
#89042=CARTESIAN_POINT('',(536.,-2.42439173773414,-11.7525454562834));
#89043=CARTESIAN_POINT('Origin',(536.,0.,0.));
#89044=CARTESIAN_POINT('',(536.,-2.30027094027665,-11.289320333896));
#89045=CARTESIAN_POINT('',(536.,-2.53320808086892,-12.1586535775562));
#89046=CARTESIAN_POINT('',(536.,-2.58311365275127,-10.7994223853394));
#89047=CARTESIAN_POINT('Origin',(536.,-2.68664127079228,-11.185792715855));
#89048=CARTESIAN_POINT('',(536.,-3.16266914852471,-10.6441309582779));
#89049=CARTESIAN_POINT('',(536.,-2.19674332223564,-10.9029500033804));
#89050=CARTESIAN_POINT('',(536.,-3.65256709708134,-10.9269736707525));
#89051=CARTESIAN_POINT('Origin',(536.,-3.26619676656572,-11.0305012887935));
#89052=CARTESIAN_POINT('',(536.,-3.77668789453883,-11.3901987931398));
#89053=CARTESIAN_POINT('',(536.,-3.54903947904034,-10.5406033402369));
#89054=CARTESIAN_POINT('',(536.,-5.38356518503846,-10.7246084263455));
#89055=CARTESIAN_POINT('Origin',(536.,0.,0.));
#89056=CARTESIAN_POINT('',(536.,-5.1437822173509,-10.309292143521));
#89057=CARTESIAN_POINT('',(536.,-5.5937822173509,-11.088715006927));
#89058=CARTESIAN_POINT('',(536.,-5.29019237886467,-9.76288198200726));
#89059=CARTESIAN_POINT('Origin',(536.,-5.49019237886467,-10.109292143521));
#89060=CARTESIAN_POINT('',(536.,-5.80980762113534,-9.46288198200726));
#89061=CARTESIAN_POINT('',(536.,-4.9437822173509,-9.96288198200727));
#89062=CARTESIAN_POINT('',(536.,-6.35621778264911,-9.60929214352104));
#89063=CARTESIAN_POINT('Origin',(536.,-6.00980762113534,-9.80929214352104));
#89064=CARTESIAN_POINT('',(536.,-6.59600075033667,-10.0246084263455));
#89065=CARTESIAN_POINT('',(536.,-6.15621778264911,-9.26288198200726));
#89066=CARTESIAN_POINT('',(536.,-7.97585756174453,-8.96580705540569));
#89067=CARTESIAN_POINT('Origin',(536.,0.,0.));
#89068=CARTESIAN_POINT('',(536.,-7.63675323681472,-8.62670273047588));
#89069=CARTESIAN_POINT('',(536.,-8.27314933988261,-9.26309883354377));
#89070=CARTESIAN_POINT('',(536.,-7.63675323681472,-8.06101730552664));
#89071=CARTESIAN_POINT('Origin',(536.,-7.91959594928934,-8.34386001800125));
#89072=CARTESIAN_POINT('',(536.,-8.06101730552665,-7.63675323681471));
#89073=CARTESIAN_POINT('',(536.,-7.3539105243401,-8.34386001800125));
#89074=CARTESIAN_POINT('',(536.,-8.62670273047588,-7.63675323681471));
#89075=CARTESIAN_POINT('Origin',(536.,-8.34386001800126,-7.91959594928933));
#89076=CARTESIAN_POINT('',(536.,-8.9658070554057,-7.97585756174453));
#89077=CARTESIAN_POINT('',(536.,-8.34386001800126,-7.35391052434009));
#89078=CARTESIAN_POINT('',(536.,-10.0246084263455,-6.59600075033666));
#89079=CARTESIAN_POINT('Origin',(536.,0.,0.));
#89080=CARTESIAN_POINT('',(536.,-9.60929214352105,-6.3562177826491));
#89081=CARTESIAN_POINT('',(536.,-10.388715006927,-6.8062177826491));
#89082=CARTESIAN_POINT('',(536.,-9.46288198200727,-5.80980762113533));
#89083=CARTESIAN_POINT('Origin',(536.,-9.80929214352104,-6.00980762113533));
#89084=CARTESIAN_POINT('',(536.,-9.76288198200727,-5.29019237886466));
#89085=CARTESIAN_POINT('',(536.,-9.26288198200727,-6.1562177826491));
#89086=CARTESIAN_POINT('',(536.,-10.309292143521,-5.14378221735089));
#89087=CARTESIAN_POINT('Origin',(536.,-10.109292143521,-5.49019237886466));
#89088=CARTESIAN_POINT('',(536.,-10.7246084263455,-5.38356518503845));
#89089=CARTESIAN_POINT('',(536.,-9.96288198200727,-4.94378221735089));
#89090=CARTESIAN_POINT('',(536.,-11.3901987931398,-3.77668789453882));
#89091=CARTESIAN_POINT('Origin',(536.,0.,0.));
#89092=CARTESIAN_POINT('',(536.,-10.9269736707525,-3.65256709708133));
#89093=CARTESIAN_POINT('',(536.,-11.7963069144127,-3.8855042376736));
#89094=CARTESIAN_POINT('',(536.,-10.6441309582779,-3.1626691485247));
#89095=CARTESIAN_POINT('Origin',(536.,-11.0305012887935,-3.2661967665657));
#89096=CARTESIAN_POINT('',(536.,-10.7994223853394,-2.58311365275126));
#89097=CARTESIAN_POINT('',(536.,-10.5406033402369,-3.54903947904032));
#89098=CARTESIAN_POINT('',(536.,-11.2893203338961,-2.30027094027664));
#89099=CARTESIAN_POINT('Origin',(536.,-11.185792715855,-2.68664127079226));
#89100=CARTESIAN_POINT('',(536.,-11.7525454562834,-2.42439173773412));
#89101=CARTESIAN_POINT('',(536.,-10.9029500033804,-2.19674332223563));
#89102=CARTESIAN_POINT('',(536.,-11.9795659353751,-0.699999999999998));
#89103=CARTESIAN_POINT('Origin',(536.,0.,0.));
#89104=CARTESIAN_POINT('',(536.,-11.5,-0.699999999999999));
#89105=CARTESIAN_POINT('',(536.,-12.4,-0.699999999999998));
#89106=CARTESIAN_POINT('',(536.,-11.1,-0.299999999999998));
#89107=CARTESIAN_POINT('Origin',(536.,-11.5,-0.299999999999998));
#89108=CARTESIAN_POINT('',(536.,-11.1,0.300000000000001));
#89109=CARTESIAN_POINT('',(536.,-11.1,-0.699999999999999));
#89110=CARTESIAN_POINT('',(536.,-11.5,0.700000000000001));
#89111=CARTESIAN_POINT('Origin',(536.,-11.5,0.300000000000001));
#89112=CARTESIAN_POINT('',(536.,-11.9795659353751,0.700000000000002));
#89113=CARTESIAN_POINT('',(536.,-11.1,0.700000000000001));
#89114=CARTESIAN_POINT('',(536.,-11.7525454562834,2.42439173773413));
#89115=CARTESIAN_POINT('Origin',(536.,0.,0.));
#89116=CARTESIAN_POINT('',(536.,-11.289320333896,2.30027094027664));
#89117=CARTESIAN_POINT('',(536.,-12.1586535775562,2.53320808086891));
#89118=CARTESIAN_POINT('',(536.,-10.7994223853394,2.58311365275126));
#89119=CARTESIAN_POINT('Origin',(536.,-11.185792715855,2.68664127079227));
#89120=CARTESIAN_POINT('',(536.,-10.6441309582779,3.1626691485247));
#89121=CARTESIAN_POINT('',(536.,-10.9029500033804,2.19674332223564));
#89122=CARTESIAN_POINT('',(536.,-10.9269736707525,3.65256709708134));
#89123=CARTESIAN_POINT('Origin',(536.,-11.0305012887935,3.26619676656571));
#89124=CARTESIAN_POINT('',(536.,-11.3901987931398,3.77668789453883));
#89125=CARTESIAN_POINT('',(536.,-10.5406033402369,3.54903947904033));
#89126=CARTESIAN_POINT('',(536.,-10.7246084263455,5.38356518503846));
#89127=CARTESIAN_POINT('Origin',(536.,0.,0.));
#89128=CARTESIAN_POINT('',(536.,-10.309292143521,5.1437822173509));
#89129=CARTESIAN_POINT('',(536.,-11.088715006927,5.5937822173509));
#89130=CARTESIAN_POINT('',(536.,-9.76288198200727,5.29019237886467));
#89131=CARTESIAN_POINT('Origin',(536.,-10.109292143521,5.49019237886467));
#89132=CARTESIAN_POINT('',(536.,-9.46288198200727,5.80980762113533));
#89133=CARTESIAN_POINT('',(536.,-9.96288198200727,4.9437822173509));
#89134=CARTESIAN_POINT('',(536.,-9.60929214352104,6.35621778264911));
#89135=CARTESIAN_POINT('Origin',(536.,-9.80929214352104,6.00980762113534));
#89136=CARTESIAN_POINT('',(536.,-10.0246084263455,6.59600075033667));
#89137=CARTESIAN_POINT('',(536.,-9.26288198200727,6.15621778264911));
#89138=CARTESIAN_POINT('',(536.,-8.9658070554057,7.97585756174453));
#89139=CARTESIAN_POINT('Origin',(536.,0.,0.));
#89140=CARTESIAN_POINT('',(536.,-8.62670273047588,7.63675323681471));
#89141=CARTESIAN_POINT('',(536.,-9.26309883354377,8.27314933988261));
#89142=CARTESIAN_POINT('',(536.,-8.06101730552664,7.63675323681471));
#89143=CARTESIAN_POINT('Origin',(536.,-8.34386001800126,7.91959594928933));
#89144=CARTESIAN_POINT('',(536.,-7.63675323681471,8.06101730552664));
#89145=CARTESIAN_POINT('',(536.,-8.34386001800126,7.35391052434009));
#89146=CARTESIAN_POINT('',(536.,-7.63675323681471,8.62670273047588));
#89147=CARTESIAN_POINT('Origin',(536.,-7.91959594928933,8.34386001800126));
#89148=CARTESIAN_POINT('',(536.,-7.97585756174453,8.9658070554057));
#89149=CARTESIAN_POINT('',(536.,-7.35391052434009,8.34386001800126));
#89150=CARTESIAN_POINT('',(536.,-6.59600075033666,10.0246084263455));
#89151=CARTESIAN_POINT('Origin',(536.,0.,0.));
#89152=CARTESIAN_POINT('',(536.,-6.3562177826491,9.60929214352105));
#89153=CARTESIAN_POINT('',(536.,-6.8062177826491,10.388715006927));
#89154=CARTESIAN_POINT('',(536.,-5.80980762113533,9.46288198200727));
#89155=CARTESIAN_POINT('Origin',(536.,-6.00980762113533,9.80929214352104));
#89156=CARTESIAN_POINT('',(536.,-5.29019237886467,9.76288198200727));
#89157=CARTESIAN_POINT('',(536.,-6.1562177826491,9.26288198200727));
#89158=CARTESIAN_POINT('',(536.,-5.14378221735089,10.309292143521));
#89159=CARTESIAN_POINT('Origin',(536.,-5.49019237886467,10.109292143521));
#89160=CARTESIAN_POINT('',(536.,-5.38356518503845,10.7246084263455));
#89161=CARTESIAN_POINT('',(536.,-4.94378221735089,9.96288198200727));
#89162=CARTESIAN_POINT('',(536.,-3.77668789453882,11.3901987931398));
#89163=CARTESIAN_POINT('Origin',(536.,0.,0.));
#89164=CARTESIAN_POINT('',(536.,-3.65256709708133,10.9269736707525));
#89165=CARTESIAN_POINT('',(536.,-3.8855042376736,11.7963069144127));
#89166=CARTESIAN_POINT('',(536.,-3.1626691485247,10.6441309582779));
#89167=CARTESIAN_POINT('Origin',(536.,-3.26619676656571,11.0305012887935));
#89168=CARTESIAN_POINT('',(536.,-2.58311365275126,10.7994223853394));
#89169=CARTESIAN_POINT('',(536.,-3.54903947904033,10.5406033402369));
#89170=CARTESIAN_POINT('',(536.,-2.30027094027664,11.289320333896));
#89171=CARTESIAN_POINT('Origin',(536.,-2.68664127079227,11.185792715855));
#89172=CARTESIAN_POINT('',(536.,-2.42439173773413,11.7525454562834));
#89173=CARTESIAN_POINT('',(536.,-2.19674332223563,10.9029500033804));
#89174=CARTESIAN_POINT('',(536.,-0.699999999999999,11.9795659353751));
#89175=CARTESIAN_POINT('Origin',(536.,0.,0.));
#89176=CARTESIAN_POINT('',(536.,-0.699999999999999,11.5));
#89177=CARTESIAN_POINT('',(536.,-0.699999999999999,12.4));
#89178=CARTESIAN_POINT('',(536.,-0.299999999999999,11.1));
#89179=CARTESIAN_POINT('Origin',(536.,-0.299999999999999,11.5));
#89180=CARTESIAN_POINT('',(536.,0.300000000000001,11.1));
#89181=CARTESIAN_POINT('',(536.,-0.699999999999999,11.1));
#89182=CARTESIAN_POINT('',(536.,0.700000000000001,11.5));
#89183=CARTESIAN_POINT('Origin',(536.,0.300000000000001,11.5));
#89184=CARTESIAN_POINT('',(536.,0.700000000000001,11.9795659353751));
#89185=CARTESIAN_POINT('',(536.,0.700000000000001,11.1));
#89186=CARTESIAN_POINT('',(536.,2.42439173773413,11.7525454562834));
#89187=CARTESIAN_POINT('Origin',(536.,0.,0.));
#89188=CARTESIAN_POINT('',(536.,2.30027094027664,11.289320333896));
#89189=CARTESIAN_POINT('',(536.,2.53320808086891,12.1586535775562));
#89190=CARTESIAN_POINT('',(536.,2.58311365275126,10.7994223853394));
#89191=CARTESIAN_POINT('Origin',(536.,2.68664127079227,11.185792715855));
#89192=CARTESIAN_POINT('',(536.,3.1626691485247,10.6441309582779));
#89193=CARTESIAN_POINT('',(536.,2.19674332223563,10.9029500033804));
#89194=CARTESIAN_POINT('',(536.,3.65256709708134,10.9269736707525));
#89195=CARTESIAN_POINT('Origin',(536.,3.26619676656571,11.0305012887935));
#89196=CARTESIAN_POINT('',(536.,3.77668789453883,11.3901987931398));
#89197=CARTESIAN_POINT('',(536.,3.54903947904033,10.5406033402369));
#89198=CARTESIAN_POINT('',(536.,5.38356518503846,10.7246084263455));
#89199=CARTESIAN_POINT('Origin',(536.,0.,0.));
#89200=CARTESIAN_POINT('',(536.,5.14378221735089,10.309292143521));
#89201=CARTESIAN_POINT('',(536.,5.59378221735089,11.088715006927));
#89202=CARTESIAN_POINT('',(536.,5.29019237886467,9.76288198200727));
#89203=CARTESIAN_POINT('Origin',(536.,5.49019237886467,10.109292143521));
#89204=CARTESIAN_POINT('',(536.,5.80980762113533,9.46288198200727));
#89205=CARTESIAN_POINT('',(536.,4.94378221735089,9.96288198200727));
#89206=CARTESIAN_POINT('',(536.,6.35621778264911,9.60929214352104));
#89207=CARTESIAN_POINT('Origin',(536.,6.00980762113533,9.80929214352104));
#89208=CARTESIAN_POINT('',(536.,6.59600075033667,10.0246084263455));
#89209=CARTESIAN_POINT('',(536.,6.15621778264911,9.26288198200727));
#89210=CARTESIAN_POINT('',(536.,7.97585756174453,8.9658070554057));
#89211=CARTESIAN_POINT('Origin',(536.,0.,0.));
#89212=CARTESIAN_POINT('',(536.,7.63675323681471,8.62670273047588));
#89213=CARTESIAN_POINT('',(536.,8.27314933988261,9.26309883354377));
#89214=CARTESIAN_POINT('',(536.,7.63675323681471,8.06101730552664));
#89215=CARTESIAN_POINT('Origin',(536.,7.91959594928933,8.34386001800126));
#89216=CARTESIAN_POINT('',(536.,8.06101730552664,7.63675323681471));
#89217=CARTESIAN_POINT('',(536.,7.35391052434009,8.34386001800126));
#89218=CARTESIAN_POINT('',(536.,8.62670273047588,7.63675323681471));
#89219=CARTESIAN_POINT('Origin',(536.,8.34386001800126,7.91959594928933));
#89220=CARTESIAN_POINT('',(536.,8.9658070554057,7.97585756174453));
#89221=CARTESIAN_POINT('',(536.,8.34386001800126,7.35391052434009));
#89222=CARTESIAN_POINT('',(536.,10.0246084263455,6.59600075033667));
#89223=CARTESIAN_POINT('Origin',(536.,0.,0.));
#89224=CARTESIAN_POINT('',(536.,9.60929214352104,6.35621778264911));
#89225=CARTESIAN_POINT('',(536.,10.388715006927,6.80621778264911));
#89226=CARTESIAN_POINT('',(536.,9.46288198200727,5.80980762113533));
#89227=CARTESIAN_POINT('Origin',(536.,9.80929214352104,6.00980762113533));
#89228=CARTESIAN_POINT('',(536.,9.76288198200727,5.29019237886467));
#89229=CARTESIAN_POINT('',(536.,9.26288198200727,6.1562177826491));
#89230=CARTESIAN_POINT('',(536.,10.309292143521,5.14378221735089));
#89231=CARTESIAN_POINT('Origin',(536.,10.109292143521,5.49019237886467));
#89232=CARTESIAN_POINT('',(536.,10.7246084263455,5.38356518503845));
#89233=CARTESIAN_POINT('',(536.,9.96288198200727,4.94378221735089));
#89234=CARTESIAN_POINT('',(536.,11.3901987931398,3.77668789453882));
#89235=CARTESIAN_POINT('Origin',(536.,0.,0.));
#89236=CARTESIAN_POINT('',(536.,10.9269736707525,3.65256709708134));
#89237=CARTESIAN_POINT('',(536.,11.7963069144127,3.8855042376736));
#89238=CARTESIAN_POINT('',(536.,10.6441309582779,3.1626691485247));
#89239=CARTESIAN_POINT('Origin',(536.,11.0305012887935,3.26619676656571));
#89240=CARTESIAN_POINT('',(536.,10.7994223853394,2.58311365275126));
#89241=CARTESIAN_POINT('',(536.,10.5406033402369,3.54903947904033));
#89242=CARTESIAN_POINT('',(536.,11.289320333896,2.30027094027664));
#89243=CARTESIAN_POINT('Origin',(536.,11.185792715855,2.68664127079227));
#89244=CARTESIAN_POINT('',(536.,11.7525454562834,2.42439173773413));
#89245=CARTESIAN_POINT('',(536.,10.9029500033804,2.19674332223563));
#89246=CARTESIAN_POINT('Origin',(536.,0.,0.));
#89247=CARTESIAN_POINT('Origin',(518.,11.5,-0.3));
#89248=CARTESIAN_POINT('',(518.,11.1,-0.3));
#89249=CARTESIAN_POINT('',(518.,11.1,-0.3));
#89250=CARTESIAN_POINT('',(518.,11.5,-0.7));
#89251=CARTESIAN_POINT('Origin',(518.,11.5,-0.3));
#89252=CARTESIAN_POINT('',(518.,11.5,-0.7));
#89253=CARTESIAN_POINT('Origin',(518.,11.1,-0.7));
#89254=CARTESIAN_POINT('',(518.,11.9795659353751,-0.7));
#89255=CARTESIAN_POINT('',(518.,11.1,-0.7));
#89256=CARTESIAN_POINT('',(527.,11.9795659353751,-0.7));
#89257=CARTESIAN_POINT('Origin',(518.,14.4,0.));
#89258=CARTESIAN_POINT('',(518.,-8.31079580944076,-11.5562270847922));
#89259=CARTESIAN_POINT('Ctrl Pts',(518.,-8.31079580944073,-11.5562270847922));
#89260=CARTESIAN_POINT('Ctrl Pts',(518.,-7.92493306034251,-11.8337247918152));
#89261=CARTESIAN_POINT('Ctrl Pts',(517.999999999999,-7.56211372395728,-12.1432119810277));
#89262=CARTESIAN_POINT('Ctrl Pts',(518.,-7.20642273568582,-12.4649491553181));
#89263=CARTESIAN_POINT('Ctrl Pts',(518.,-7.20321109951219,-12.467857196463));
#89264=CARTESIAN_POINT('Ctrl Pts',(518.,-7.20000000000004,-12.470765814496));
#89265=CARTESIAN_POINT('',(518.,-8.31079580944094,11.5562270847921));
#89266=CARTESIAN_POINT('Origin',(518.,0.,0.));
#89267=CARTESIAN_POINT('Ctrl Pts',(518.,-7.20000000000003,12.470765814496));
#89268=CARTESIAN_POINT('Ctrl Pts',(518.,-7.20321114074589,12.4678571591407));
#89269=CARTESIAN_POINT('Ctrl Pts',(518.,-7.20642281814689,12.464949080675));
#89270=CARTESIAN_POINT('Ctrl Pts',(518.000000000001,-7.56211380885965,12.1432119087018));
#89271=CARTESIAN_POINT('Ctrl Pts',(518.,-7.92493310544876,11.8337247593766));
#89272=CARTESIAN_POINT('Ctrl Pts',(518.,-8.31079580944093,11.5562270847921));
#89273=CARTESIAN_POINT('',(518.,-5.85258832261145,12.9754738390371));
#89274=CARTESIAN_POINT('Ctrl Pts',(518.,-5.85258832261145,12.975473839037));
#89275=CARTESIAN_POINT('Ctrl Pts',(518.,-6.28583976093444,12.7800557494554));
#89276=CARTESIAN_POINT('Ctrl Pts',(518.000000000003,-6.73527319767247,12.6205885830549));
#89277=CARTESIAN_POINT('Ctrl Pts',(518.,-7.19175125752897,12.4734197371684));
#89278=CARTESIAN_POINT('Ctrl Pts',(518.,-7.19587551313739,12.4720923992309));
#89279=CARTESIAN_POINT('Ctrl Pts',(518.,-7.20000000000001,12.470765814496));
#89280=CARTESIAN_POINT('',(518.,14.1633841320522,1.41924675424466));
#89281=CARTESIAN_POINT('Origin',(518.,0.,0.));
#89282=CARTESIAN_POINT('Ctrl Pts',(518.,14.4000000000001,3.05311331771918E-15));
#89283=CARTESIAN_POINT('Ctrl Pts',(518.,14.3990866009235,0.00423525713834081));
#89284=CARTESIAN_POINT('Ctrl Pts',(518.,14.3981739698498,0.00847069060670547));
#89285=CARTESIAN_POINT('Ctrl Pts',(518.000000000002,14.2973868934641,0.477376708780995));
#89286=CARTESIAN_POINT('Ctrl Pts',(518.,14.2107728157373,0.946331012921918));
#89287=CARTESIAN_POINT('Ctrl Pts',(518.,14.1633841320521,1.41924675424464));
#89288=CARTESIAN_POINT('',(518.,14.1633841320522,-1.41924675424485));
#89289=CARTESIAN_POINT('Ctrl Pts',(518.,14.1633841320522,-1.41924675424483));
#89290=CARTESIAN_POINT('Ctrl Pts',(518.,14.210772821277,-0.946330957640153));
#89291=CARTESIAN_POINT('Ctrl Pts',(517.999999999997,14.2973869135097,-0.477376599365992));
#89292=CARTESIAN_POINT('Ctrl Pts',(518.,14.3981739932752,-0.00847058186628403));
#89293=CARTESIAN_POINT('Ctrl Pts',(518.,14.3990866126494,-0.00423520276807552));
#89294=CARTESIAN_POINT('Ctrl Pts',(518.,14.4000000000001,-1.94289029309402E-15));
#89295=CARTESIAN_POINT('',(518.,-5.85258832261171,-12.9754738390369));
#89296=CARTESIAN_POINT('Origin',(518.,0.,0.));
#89297=CARTESIAN_POINT('Ctrl Pts',(518.,-7.20000000000004,-12.470765814496));
#89298=CARTESIAN_POINT('Ctrl Pts',(518.,-7.19587546018855,-12.4720924162615));
#89299=CARTESIAN_POINT('Ctrl Pts',(518.,-7.19175066797431,-12.4734199188406));
#89300=CARTESIAN_POINT('Ctrl Pts',(518.000000000003,-6.73517810085928,-12.6206205967494));
#89301=CARTESIAN_POINT('Ctrl Pts',(518.,-6.28600287595523,-12.7799821764146));
#89302=CARTESIAN_POINT('Ctrl Pts',(518.,-5.8525883226117,-12.9754738390369));
#89303=CARTESIAN_POINT('',(518.,11.7525454562834,2.42439173773413));
#89304=CARTESIAN_POINT('Origin',(518.,0.,0.));
#89305=CARTESIAN_POINT('',(518.,11.289320333896,2.30027094027664));
#89306=CARTESIAN_POINT('',(518.,10.9029500033804,2.19674332223563));
#89307=CARTESIAN_POINT('',(518.,10.7994223853394,2.58311365275126));
#89308=CARTESIAN_POINT('Origin',(518.,11.185792715855,2.68664127079227));
#89309=CARTESIAN_POINT('',(518.,10.6441309582779,3.1626691485247));
#89310=CARTESIAN_POINT('',(518.,10.5406033402369,3.54903947904033));
#89311=CARTESIAN_POINT('',(518.,10.9269736707525,3.65256709708134));
#89312=CARTESIAN_POINT('Origin',(518.,11.0305012887935,3.26619676656571));
#89313=CARTESIAN_POINT('',(518.,11.3901987931398,3.77668789453882));
#89314=CARTESIAN_POINT('',(518.,11.7963069144127,3.8855042376736));
#89315=CARTESIAN_POINT('',(518.,10.7246084263455,5.38356518503845));
#89316=CARTESIAN_POINT('Origin',(518.,0.,0.));
#89317=CARTESIAN_POINT('',(518.,10.309292143521,5.14378221735089));
#89318=CARTESIAN_POINT('',(518.,9.96288198200727,4.94378221735089));
#89319=CARTESIAN_POINT('',(518.,9.76288198200727,5.29019237886467));
#89320=CARTESIAN_POINT('Origin',(518.,10.109292143521,5.49019237886467));
#89321=CARTESIAN_POINT('',(518.,9.46288198200727,5.80980762113533));
#89322=CARTESIAN_POINT('',(518.,9.26288198200727,6.1562177826491));
#89323=CARTESIAN_POINT('',(518.,9.60929214352104,6.35621778264911));
#89324=CARTESIAN_POINT('Origin',(518.,9.80929214352104,6.00980762113533));
#89325=CARTESIAN_POINT('',(518.,10.0246084263455,6.59600075033667));
#89326=CARTESIAN_POINT('',(518.,10.388715006927,6.80621778264911));
#89327=CARTESIAN_POINT('',(518.,8.9658070554057,7.97585756174453));
#89328=CARTESIAN_POINT('Origin',(518.,0.,0.));
#89329=CARTESIAN_POINT('',(518.,8.62670273047588,7.63675323681471));
#89330=CARTESIAN_POINT('',(518.,8.34386001800126,7.35391052434009));
#89331=CARTESIAN_POINT('',(518.,8.06101730552664,7.63675323681471));
#89332=CARTESIAN_POINT('Origin',(518.,8.34386001800126,7.91959594928933));
#89333=CARTESIAN_POINT('',(518.,7.63675323681471,8.06101730552664));
#89334=CARTESIAN_POINT('',(518.,7.35391052434009,8.34386001800126));
#89335=CARTESIAN_POINT('',(518.,7.63675323681471,8.62670273047588));
#89336=CARTESIAN_POINT('Origin',(518.,7.91959594928933,8.34386001800126));
#89337=CARTESIAN_POINT('',(518.,7.97585756174453,8.9658070554057));
#89338=CARTESIAN_POINT('',(518.,8.27314933988261,9.26309883354377));
#89339=CARTESIAN_POINT('',(518.,6.59600075033667,10.0246084263455));
#89340=CARTESIAN_POINT('Origin',(518.,0.,0.));
#89341=CARTESIAN_POINT('',(518.,6.35621778264911,9.60929214352104));
#89342=CARTESIAN_POINT('',(518.,6.15621778264911,9.26288198200727));
#89343=CARTESIAN_POINT('',(518.,5.80980762113533,9.46288198200727));
#89344=CARTESIAN_POINT('Origin',(518.,6.00980762113533,9.80929214352104));
#89345=CARTESIAN_POINT('',(518.,5.29019237886467,9.76288198200727));
#89346=CARTESIAN_POINT('',(518.,4.94378221735089,9.96288198200727));
#89347=CARTESIAN_POINT('',(518.,5.14378221735089,10.309292143521));
#89348=CARTESIAN_POINT('Origin',(518.,5.49019237886467,10.109292143521));
#89349=CARTESIAN_POINT('',(518.,5.38356518503846,10.7246084263455));
#89350=CARTESIAN_POINT('',(518.,5.59378221735089,11.088715006927));
#89351=CARTESIAN_POINT('',(518.,3.77668789453883,11.3901987931398));
#89352=CARTESIAN_POINT('Origin',(518.,0.,0.));
#89353=CARTESIAN_POINT('',(518.,3.65256709708134,10.9269736707525));
#89354=CARTESIAN_POINT('',(518.,3.54903947904033,10.5406033402369));
#89355=CARTESIAN_POINT('',(518.,3.1626691485247,10.6441309582779));
#89356=CARTESIAN_POINT('Origin',(518.,3.26619676656571,11.0305012887935));
#89357=CARTESIAN_POINT('',(518.,2.58311365275126,10.7994223853394));
#89358=CARTESIAN_POINT('',(518.,2.19674332223563,10.9029500033804));
#89359=CARTESIAN_POINT('',(518.,2.30027094027664,11.289320333896));
#89360=CARTESIAN_POINT('Origin',(518.,2.68664127079227,11.185792715855));
#89361=CARTESIAN_POINT('',(518.,2.42439173773413,11.7525454562834));
#89362=CARTESIAN_POINT('',(518.,2.53320808086891,12.1586535775562));
#89363=CARTESIAN_POINT('',(518.,0.700000000000001,11.9795659353751));
#89364=CARTESIAN_POINT('Origin',(518.,0.,0.));
#89365=CARTESIAN_POINT('',(518.,0.700000000000001,11.5));
#89366=CARTESIAN_POINT('',(518.,0.700000000000001,11.1));
#89367=CARTESIAN_POINT('',(518.,0.300000000000001,11.1));
#89368=CARTESIAN_POINT('Origin',(518.,0.300000000000001,11.5));
#89369=CARTESIAN_POINT('',(518.,-0.299999999999999,11.1));
#89370=CARTESIAN_POINT('',(518.,-0.699999999999999,11.1));
#89371=CARTESIAN_POINT('',(518.,-0.699999999999999,11.5));
#89372=CARTESIAN_POINT('Origin',(518.,-0.299999999999999,11.5));
#89373=CARTESIAN_POINT('',(518.,-0.699999999999999,11.9795659353751));
#89374=CARTESIAN_POINT('',(518.,-0.699999999999999,12.4));
#89375=CARTESIAN_POINT('',(518.,-2.42439173773413,11.7525454562834));
#89376=CARTESIAN_POINT('Origin',(518.,0.,0.));
#89377=CARTESIAN_POINT('',(518.,-2.30027094027664,11.289320333896));
#89378=CARTESIAN_POINT('',(518.,-2.19674332223563,10.9029500033804));
#89379=CARTESIAN_POINT('',(518.,-2.58311365275126,10.7994223853394));
#89380=CARTESIAN_POINT('Origin',(518.,-2.68664127079227,11.185792715855));
#89381=CARTESIAN_POINT('',(518.,-3.1626691485247,10.6441309582779));
#89382=CARTESIAN_POINT('',(518.,-3.54903947904033,10.5406033402369));
#89383=CARTESIAN_POINT('',(518.,-3.65256709708133,10.9269736707525));
#89384=CARTESIAN_POINT('Origin',(518.,-3.26619676656571,11.0305012887935));
#89385=CARTESIAN_POINT('',(518.,-3.77668789453882,11.3901987931398));
#89386=CARTESIAN_POINT('',(518.,-3.8855042376736,11.7963069144127));
#89387=CARTESIAN_POINT('',(518.,-5.38356518503845,10.7246084263455));
#89388=CARTESIAN_POINT('Origin',(518.,0.,0.));
#89389=CARTESIAN_POINT('',(518.,-5.14378221735089,10.309292143521));
#89390=CARTESIAN_POINT('',(518.,-4.94378221735089,9.96288198200727));
#89391=CARTESIAN_POINT('',(518.,-5.29019237886467,9.76288198200727));
#89392=CARTESIAN_POINT('Origin',(518.,-5.49019237886467,10.109292143521));
#89393=CARTESIAN_POINT('',(518.,-5.80980762113533,9.46288198200727));
#89394=CARTESIAN_POINT('',(518.,-6.1562177826491,9.26288198200727));
#89395=CARTESIAN_POINT('',(518.,-6.3562177826491,9.60929214352105));
#89396=CARTESIAN_POINT('Origin',(518.,-6.00980762113533,9.80929214352104));
#89397=CARTESIAN_POINT('',(518.,-6.59600075033666,10.0246084263455));
#89398=CARTESIAN_POINT('',(518.,-6.8062177826491,10.388715006927));
#89399=CARTESIAN_POINT('',(518.,-7.97585756174453,8.9658070554057));
#89400=CARTESIAN_POINT('Origin',(518.,0.,0.));
#89401=CARTESIAN_POINT('',(518.,-7.63675323681471,8.62670273047588));
#89402=CARTESIAN_POINT('',(518.,-7.35391052434009,8.34386001800126));
#89403=CARTESIAN_POINT('',(518.,-7.63675323681471,8.06101730552664));
#89404=CARTESIAN_POINT('Origin',(518.,-7.91959594928933,8.34386001800126));
#89405=CARTESIAN_POINT('',(518.,-8.06101730552664,7.63675323681471));
#89406=CARTESIAN_POINT('',(518.,-8.34386001800126,7.35391052434009));
#89407=CARTESIAN_POINT('',(518.,-8.62670273047588,7.63675323681471));
#89408=CARTESIAN_POINT('Origin',(518.,-8.34386001800126,7.91959594928933));
#89409=CARTESIAN_POINT('',(518.,-8.9658070554057,7.97585756174453));
#89410=CARTESIAN_POINT('',(518.,-9.26309883354377,8.27314933988261));
#89411=CARTESIAN_POINT('',(518.,-10.0246084263455,6.59600075033667));
#89412=CARTESIAN_POINT('Origin',(518.,0.,0.));
#89413=CARTESIAN_POINT('',(518.,-9.60929214352104,6.35621778264911));
#89414=CARTESIAN_POINT('',(518.,-9.26288198200727,6.15621778264911));
#89415=CARTESIAN_POINT('',(518.,-9.46288198200727,5.80980762113533));
#89416=CARTESIAN_POINT('Origin',(518.,-9.80929214352104,6.00980762113534));
#89417=CARTESIAN_POINT('',(518.,-9.76288198200727,5.29019237886467));
#89418=CARTESIAN_POINT('',(518.,-9.96288198200727,4.9437822173509));
#89419=CARTESIAN_POINT('',(518.,-10.309292143521,5.1437822173509));
#89420=CARTESIAN_POINT('Origin',(518.,-10.109292143521,5.49019237886467));
#89421=CARTESIAN_POINT('',(518.,-10.7246084263455,5.38356518503846));
#89422=CARTESIAN_POINT('',(518.,-11.088715006927,5.5937822173509));
#89423=CARTESIAN_POINT('',(518.,-11.3901987931398,3.77668789453883));
#89424=CARTESIAN_POINT('Origin',(518.,0.,0.));
#89425=CARTESIAN_POINT('',(518.,-10.9269736707525,3.65256709708134));
#89426=CARTESIAN_POINT('',(518.,-10.5406033402369,3.54903947904033));
#89427=CARTESIAN_POINT('',(518.,-10.6441309582779,3.1626691485247));
#89428=CARTESIAN_POINT('Origin',(518.,-11.0305012887935,3.26619676656571));
#89429=CARTESIAN_POINT('',(518.,-10.7994223853394,2.58311365275126));
#89430=CARTESIAN_POINT('',(518.,-10.9029500033804,2.19674332223564));
#89431=CARTESIAN_POINT('',(518.,-11.289320333896,2.30027094027664));
#89432=CARTESIAN_POINT('Origin',(518.,-11.185792715855,2.68664127079227));
#89433=CARTESIAN_POINT('',(518.,-11.7525454562834,2.42439173773413));
#89434=CARTESIAN_POINT('',(518.,-12.1586535775562,2.53320808086891));
#89435=CARTESIAN_POINT('',(518.,-11.9795659353751,0.700000000000002));
#89436=CARTESIAN_POINT('Origin',(518.,0.,0.));
#89437=CARTESIAN_POINT('',(518.,-11.5,0.700000000000001));
#89438=CARTESIAN_POINT('',(518.,-11.1,0.700000000000001));
#89439=CARTESIAN_POINT('',(518.,-11.1,0.300000000000001));
#89440=CARTESIAN_POINT('Origin',(518.,-11.5,0.300000000000001));
#89441=CARTESIAN_POINT('',(518.,-11.1,-0.299999999999998));
#89442=CARTESIAN_POINT('',(518.,-11.1,-0.699999999999999));
#89443=CARTESIAN_POINT('',(518.,-11.5,-0.699999999999999));
#89444=CARTESIAN_POINT('Origin',(518.,-11.5,-0.299999999999998));
#89445=CARTESIAN_POINT('',(518.,-11.9795659353751,-0.699999999999998));
#89446=CARTESIAN_POINT('',(518.,-12.4,-0.699999999999998));
#89447=CARTESIAN_POINT('',(518.,-11.7525454562834,-2.42439173773412));
#89448=CARTESIAN_POINT('Origin',(518.,0.,0.));
#89449=CARTESIAN_POINT('',(518.,-11.2893203338961,-2.30027094027664));
#89450=CARTESIAN_POINT('',(518.,-10.9029500033804,-2.19674332223563));
#89451=CARTESIAN_POINT('',(518.,-10.7994223853394,-2.58311365275126));
#89452=CARTESIAN_POINT('Origin',(518.,-11.185792715855,-2.68664127079226));
#89453=CARTESIAN_POINT('',(518.,-10.6441309582779,-3.1626691485247));
#89454=CARTESIAN_POINT('',(518.,-10.5406033402369,-3.54903947904032));
#89455=CARTESIAN_POINT('',(518.,-10.9269736707525,-3.65256709708133));
#89456=CARTESIAN_POINT('Origin',(518.,-11.0305012887935,-3.2661967665657));
#89457=CARTESIAN_POINT('',(518.,-11.3901987931398,-3.77668789453882));
#89458=CARTESIAN_POINT('',(518.,-11.7963069144127,-3.8855042376736));
#89459=CARTESIAN_POINT('',(518.,-10.7246084263455,-5.38356518503845));
#89460=CARTESIAN_POINT('Origin',(518.,0.,0.));
#89461=CARTESIAN_POINT('',(518.,-10.309292143521,-5.14378221735089));
#89462=CARTESIAN_POINT('',(518.,-9.96288198200727,-4.94378221735089));
#89463=CARTESIAN_POINT('',(518.,-9.76288198200727,-5.29019237886466));
#89464=CARTESIAN_POINT('Origin',(518.,-10.109292143521,-5.49019237886466));
#89465=CARTESIAN_POINT('',(518.,-9.46288198200727,-5.80980762113533));
#89466=CARTESIAN_POINT('',(518.,-9.26288198200727,-6.1562177826491));
#89467=CARTESIAN_POINT('',(518.,-9.60929214352105,-6.3562177826491));
#89468=CARTESIAN_POINT('Origin',(518.,-9.80929214352104,-6.00980762113533));
#89469=CARTESIAN_POINT('',(518.,-10.0246084263455,-6.59600075033666));
#89470=CARTESIAN_POINT('',(518.,-10.388715006927,-6.8062177826491));
#89471=CARTESIAN_POINT('',(518.,-8.9658070554057,-7.97585756174453));
#89472=CARTESIAN_POINT('Origin',(518.,0.,0.));
#89473=CARTESIAN_POINT('',(518.,-8.62670273047588,-7.63675323681471));
#89474=CARTESIAN_POINT('',(518.,-8.34386001800126,-7.35391052434009));
#89475=CARTESIAN_POINT('',(518.,-8.06101730552665,-7.63675323681471));
#89476=CARTESIAN_POINT('Origin',(518.,-8.34386001800126,-7.91959594928933));
#89477=CARTESIAN_POINT('',(518.,-7.63675323681472,-8.06101730552664));
#89478=CARTESIAN_POINT('',(518.,-7.3539105243401,-8.34386001800125));
#89479=CARTESIAN_POINT('',(518.,-7.63675323681472,-8.62670273047588));
#89480=CARTESIAN_POINT('Origin',(518.,-7.91959594928934,-8.34386001800125));
#89481=CARTESIAN_POINT('',(518.,-7.97585756174453,-8.96580705540569));
#89482=CARTESIAN_POINT('',(518.,-8.27314933988261,-9.26309883354377));
#89483=CARTESIAN_POINT('',(518.,-6.59600075033667,-10.0246084263455));
#89484=CARTESIAN_POINT('Origin',(518.,0.,0.));
#89485=CARTESIAN_POINT('',(518.,-6.35621778264911,-9.60929214352104));
#89486=CARTESIAN_POINT('',(518.,-6.15621778264911,-9.26288198200726));
#89487=CARTESIAN_POINT('',(518.,-5.80980762113534,-9.46288198200726));
#89488=CARTESIAN_POINT('Origin',(518.,-6.00980762113534,-9.80929214352104));
#89489=CARTESIAN_POINT('',(518.,-5.29019237886467,-9.76288198200726));
#89490=CARTESIAN_POINT('',(518.,-4.9437822173509,-9.96288198200727));
#89491=CARTESIAN_POINT('',(518.,-5.1437822173509,-10.309292143521));
#89492=CARTESIAN_POINT('Origin',(518.,-5.49019237886467,-10.109292143521));
#89493=CARTESIAN_POINT('',(518.,-5.38356518503846,-10.7246084263455));
#89494=CARTESIAN_POINT('',(518.,-5.5937822173509,-11.088715006927));
#89495=CARTESIAN_POINT('',(518.,-3.77668789453883,-11.3901987931398));
#89496=CARTESIAN_POINT('Origin',(518.,0.,0.));
#89497=CARTESIAN_POINT('',(518.,-3.65256709708134,-10.9269736707525));
#89498=CARTESIAN_POINT('',(518.,-3.54903947904034,-10.5406033402369));
#89499=CARTESIAN_POINT('',(518.,-3.16266914852471,-10.6441309582779));
#89500=CARTESIAN_POINT('Origin',(518.,-3.26619676656572,-11.0305012887935));
#89501=CARTESIAN_POINT('',(518.,-2.58311365275127,-10.7994223853394));
#89502=CARTESIAN_POINT('',(518.,-2.19674332223564,-10.9029500033804));
#89503=CARTESIAN_POINT('',(518.,-2.30027094027665,-11.289320333896));
#89504=CARTESIAN_POINT('Origin',(518.,-2.68664127079228,-11.185792715855));
#89505=CARTESIAN_POINT('',(518.,-2.42439173773414,-11.7525454562834));
#89506=CARTESIAN_POINT('',(518.,-2.53320808086892,-12.1586535775562));
#89507=CARTESIAN_POINT('',(518.,-0.700000000000002,-11.9795659353751));
#89508=CARTESIAN_POINT('Origin',(518.,0.,0.));
#89509=CARTESIAN_POINT('',(518.,-0.700000000000002,-11.5));
#89510=CARTESIAN_POINT('',(518.,-0.700000000000002,-11.1));
#89511=CARTESIAN_POINT('',(518.,-0.300000000000002,-11.1));
#89512=CARTESIAN_POINT('Origin',(518.,-0.300000000000002,-11.5));
#89513=CARTESIAN_POINT('',(518.,0.299999999999998,-11.1));
#89514=CARTESIAN_POINT('',(518.,0.699999999999998,-11.1));
#89515=CARTESIAN_POINT('',(518.,0.699999999999998,-11.5));
#89516=CARTESIAN_POINT('Origin',(518.,0.299999999999998,-11.5));
#89517=CARTESIAN_POINT('',(518.,0.699999999999998,-11.9795659353751));
#89518=CARTESIAN_POINT('',(518.,0.699999999999998,-12.4));
#89519=CARTESIAN_POINT('',(518.,2.42439173773412,-11.7525454562834));
#89520=CARTESIAN_POINT('Origin',(518.,0.,0.));
#89521=CARTESIAN_POINT('',(518.,2.30027094027664,-11.2893203338961));
#89522=CARTESIAN_POINT('',(518.,2.19674332223563,-10.9029500033804));
#89523=CARTESIAN_POINT('',(518.,2.58311365275125,-10.7994223853394));
#89524=CARTESIAN_POINT('Origin',(518.,2.68664127079226,-11.185792715855));
#89525=CARTESIAN_POINT('',(518.,3.1626691485247,-10.6441309582779));
#89526=CARTESIAN_POINT('',(518.,3.54903947904032,-10.5406033402369));
#89527=CARTESIAN_POINT('',(518.,3.65256709708133,-10.9269736707525));
#89528=CARTESIAN_POINT('Origin',(518.,3.2661967665657,-11.0305012887935));
#89529=CARTESIAN_POINT('',(518.,3.77668789453882,-11.3901987931398));
#89530=CARTESIAN_POINT('',(518.,3.8855042376736,-11.7963069144127));
#89531=CARTESIAN_POINT('',(518.,5.38356518503844,-10.7246084263456));
#89532=CARTESIAN_POINT('Origin',(518.,0.,0.));
#89533=CARTESIAN_POINT('',(518.,5.14378221735088,-10.309292143521));
#89534=CARTESIAN_POINT('',(518.,4.94378221735088,-9.96288198200727));
#89535=CARTESIAN_POINT('',(518.,5.29019237886466,-9.76288198200727));
#89536=CARTESIAN_POINT('Origin',(518.,5.49019237886466,-10.109292143521));
#89537=CARTESIAN_POINT('',(518.,5.80980762113532,-9.46288198200727));
#89538=CARTESIAN_POINT('',(518.,6.1562177826491,-9.26288198200727));
#89539=CARTESIAN_POINT('',(518.,6.3562177826491,-9.60929214352105));
#89540=CARTESIAN_POINT('Origin',(518.,6.00980762113532,-9.80929214352105));
#89541=CARTESIAN_POINT('',(518.,6.59600075033666,-10.0246084263456));
#89542=CARTESIAN_POINT('',(518.,6.8062177826491,-10.388715006927));
#89543=CARTESIAN_POINT('',(518.,7.97585756174453,-8.9658070554057));
#89544=CARTESIAN_POINT('Origin',(518.,0.,0.));
#89545=CARTESIAN_POINT('',(518.,7.63675323681471,-8.62670273047588));
#89546=CARTESIAN_POINT('',(518.,7.35391052434009,-8.34386001800126));
#89547=CARTESIAN_POINT('',(518.,7.63675323681471,-8.06101730552664));
#89548=CARTESIAN_POINT('Origin',(518.,7.91959594928933,-8.34386001800126));
#89549=CARTESIAN_POINT('',(518.,8.06101730552664,-7.63675323681472));
#89550=CARTESIAN_POINT('',(518.,8.34386001800126,-7.35391052434009));
#89551=CARTESIAN_POINT('',(518.,8.62670273047588,-7.63675323681471));
#89552=CARTESIAN_POINT('Origin',(518.,8.34386001800126,-7.91959594928933));
#89553=CARTESIAN_POINT('',(518.,8.96580705540569,-7.97585756174453));
#89554=CARTESIAN_POINT('',(518.,9.26309883354377,-8.27314933988261));
#89555=CARTESIAN_POINT('',(518.,10.0246084263455,-6.59600075033667));
#89556=CARTESIAN_POINT('Origin',(518.,0.,0.));
#89557=CARTESIAN_POINT('',(518.,9.60929214352104,-6.35621778264911));
#89558=CARTESIAN_POINT('',(518.,9.26288198200726,-6.15621778264911));
#89559=CARTESIAN_POINT('',(518.,9.46288198200726,-5.80980762113534));
#89560=CARTESIAN_POINT('Origin',(518.,9.80929214352104,-6.00980762113534));
#89561=CARTESIAN_POINT('',(518.,9.76288198200726,-5.29019237886467));
#89562=CARTESIAN_POINT('',(518.,9.96288198200727,-4.9437822173509));
#89563=CARTESIAN_POINT('',(518.,10.309292143521,-5.1437822173509));
#89564=CARTESIAN_POINT('Origin',(518.,10.109292143521,-5.49019237886467));
#89565=CARTESIAN_POINT('',(518.,10.7246084263455,-5.38356518503846));
#89566=CARTESIAN_POINT('',(518.,11.088715006927,-5.5937822173509));
#89567=CARTESIAN_POINT('',(518.,11.3901987931398,-3.77668789453883));
#89568=CARTESIAN_POINT('Origin',(518.,0.,0.));
#89569=CARTESIAN_POINT('',(518.,10.9269736707525,-3.65256709708134));
#89570=CARTESIAN_POINT('',(518.,10.5406033402369,-3.54903947904034));
#89571=CARTESIAN_POINT('',(518.,10.6441309582779,-3.16266914852471));
#89572=CARTESIAN_POINT('Origin',(518.,11.0305012887935,-3.26619676656572));
#89573=CARTESIAN_POINT('',(518.,10.7994223853394,-2.58311365275127));
#89574=CARTESIAN_POINT('',(518.,10.9029500033804,-2.19674332223564));
#89575=CARTESIAN_POINT('',(518.,11.289320333896,-2.30027094027665));
#89576=CARTESIAN_POINT('Origin',(518.,11.185792715855,-2.68664127079228));
#89577=CARTESIAN_POINT('',(518.,11.7525454562834,-2.42439173773414));
#89578=CARTESIAN_POINT('',(518.,12.1586535775562,-2.53320808086892));
#89579=CARTESIAN_POINT('Origin',(518.,0.,0.));
#89580=CARTESIAN_POINT('',(518.,11.1,0.7));
#89581=CARTESIAN_POINT('Origin',(518.,11.0305012887935,3.26619676656571));
#89582=CARTESIAN_POINT('',(518.,10.9269736707525,3.65256709708134));
#89583=CARTESIAN_POINT('',(518.,10.6441309582779,3.1626691485247));
#89584=CARTESIAN_POINT('Origin',(518.,10.5406033402369,3.54903947904033));
#89585=CARTESIAN_POINT('',(518.,10.7994223853394,2.58311365275126));
#89586=CARTESIAN_POINT('Origin',(518.,11.185792715855,2.68664127079227));
#89587=CARTESIAN_POINT('',(518.,11.289320333896,2.30027094027664));
#89588=CARTESIAN_POINT('Origin',(518.,10.109292143521,5.49019237886467));
#89589=CARTESIAN_POINT('',(518.,9.76288198200727,5.29019237886467));
#89590=CARTESIAN_POINT('',(518.,10.309292143521,5.14378221735089));
#89591=CARTESIAN_POINT('Origin',(518.,9.96288198200727,4.94378221735089));
#89592=CARTESIAN_POINT('',(527.,10.7246084263455,5.38356518503845));
#89593=CARTESIAN_POINT('Origin',(518.,9.80929214352104,6.00980762113533));
#89594=CARTESIAN_POINT('',(518.,9.60929214352104,6.35621778264911));
#89595=CARTESIAN_POINT('',(518.,9.46288198200727,5.80980762113533));
#89596=CARTESIAN_POINT('Origin',(518.,10.388715006927,6.80621778264911));
#89597=CARTESIAN_POINT('',(527.,10.0246084263455,6.59600075033667));
#89598=CARTESIAN_POINT('Origin',(518.,8.34386001800126,7.91959594928933));
#89599=CARTESIAN_POINT('',(518.,8.06101730552664,7.63675323681471));
#89600=CARTESIAN_POINT('',(518.,8.62670273047588,7.63675323681471));
#89601=CARTESIAN_POINT('Origin',(518.,7.35391052434009,8.34386001800126));
#89602=CARTESIAN_POINT('',(518.,7.63675323681471,8.06101730552664));
#89603=CARTESIAN_POINT('Origin',(518.,7.91959594928933,8.34386001800126));
#89604=CARTESIAN_POINT('',(518.,7.63675323681471,8.62670273047588));
#89605=CARTESIAN_POINT('Origin',(518.,5.49019237886467,10.109292143521));
#89606=CARTESIAN_POINT('',(518.,5.14378221735089,10.309292143521));
#89607=CARTESIAN_POINT('',(518.,5.29019237886467,9.76288198200727));
#89608=CARTESIAN_POINT('Origin',(518.,4.94378221735089,9.96288198200727));
#89609=CARTESIAN_POINT('',(518.,5.80980762113533,9.46288198200727));
#89610=CARTESIAN_POINT('Origin',(518.,6.00980762113533,9.80929214352104));
#89611=CARTESIAN_POINT('',(518.,6.35621778264911,9.60929214352104));
#89612=CARTESIAN_POINT('Origin',(518.,3.26619676656571,11.0305012887935));
#89613=CARTESIAN_POINT('',(518.,3.1626691485247,10.6441309582779));
#89614=CARTESIAN_POINT('',(518.,3.65256709708134,10.9269736707525));
#89615=CARTESIAN_POINT('Origin',(518.,3.54903947904033,10.5406033402369));
#89616=CARTESIAN_POINT('',(527.,3.77668789453883,11.3901987931398));
#89617=CARTESIAN_POINT('Origin',(518.,2.68664127079227,11.185792715855));
#89618=CARTESIAN_POINT('',(518.,2.30027094027664,11.289320333896));
#89619=CARTESIAN_POINT('',(518.,2.58311365275126,10.7994223853394));
#89620=CARTESIAN_POINT('Origin',(518.,2.53320808086891,12.1586535775562));
#89621=CARTESIAN_POINT('',(527.,2.42439173773413,11.7525454562834));
#89622=CARTESIAN_POINT('Origin',(518.,0.300000000000001,11.5));
#89623=CARTESIAN_POINT('',(518.,0.3,11.1));
#89624=CARTESIAN_POINT('',(518.,0.700000000000001,11.5));
#89625=CARTESIAN_POINT('Origin',(518.,-0.699999999999999,11.1));
#89626=CARTESIAN_POINT('',(518.,-0.299999999999999,11.1));
#89627=CARTESIAN_POINT('Origin',(518.,-0.299999999999999,11.5));
#89628=CARTESIAN_POINT('',(518.,-0.699999999999999,11.5));
#89629=CARTESIAN_POINT('Origin',(518.,-3.26619676656571,11.0305012887935));
#89630=CARTESIAN_POINT('',(518.,-3.65256709708133,10.9269736707525));
#89631=CARTESIAN_POINT('',(518.,-3.1626691485247,10.6441309582779));
#89632=CARTESIAN_POINT('Origin',(518.,-3.54903947904033,10.5406033402369));
#89633=CARTESIAN_POINT('',(518.,-2.58311365275126,10.7994223853394));
#89634=CARTESIAN_POINT('Origin',(518.,-2.68664127079227,11.185792715855));
#89635=CARTESIAN_POINT('',(518.,-2.30027094027664,11.289320333896));
#89636=CARTESIAN_POINT('Origin',(518.,-5.49019237886467,10.109292143521));
#89637=CARTESIAN_POINT('',(518.,-5.29019237886467,9.76288198200727));
#89638=CARTESIAN_POINT('',(518.,-5.14378221735089,10.309292143521));
#89639=CARTESIAN_POINT('Origin',(518.,-4.94378221735089,9.96288198200727));
#89640=CARTESIAN_POINT('',(527.,-5.38356518503845,10.7246084263455));
#89641=CARTESIAN_POINT('Origin',(518.,-6.00980762113533,9.80929214352104));
#89642=CARTESIAN_POINT('',(518.,-6.3562177826491,9.60929214352105));
#89643=CARTESIAN_POINT('',(518.,-5.80980762113533,9.46288198200727));
#89644=CARTESIAN_POINT('Origin',(518.,-6.8062177826491,10.388715006927));
#89645=CARTESIAN_POINT('',(527.,-6.59600075033666,10.0246084263455));
#89646=CARTESIAN_POINT('Origin',(518.,-7.91959594928933,8.34386001800126));
#89647=CARTESIAN_POINT('',(518.,-7.63675323681471,8.06101730552664));
#89648=CARTESIAN_POINT('',(518.,-7.63675323681471,8.62670273047588));
#89649=CARTESIAN_POINT('Origin',(518.,-8.34386001800126,7.35391052434009));
#89650=CARTESIAN_POINT('',(518.,-8.06101730552664,7.63675323681471));
#89651=CARTESIAN_POINT('Origin',(518.,-8.34386001800126,7.91959594928933));
#89652=CARTESIAN_POINT('',(518.,-8.62670273047588,7.63675323681471));
#89653=CARTESIAN_POINT('Origin',(518.,-10.109292143521,5.49019237886467));
#89654=CARTESIAN_POINT('',(518.,-10.309292143521,5.1437822173509));
#89655=CARTESIAN_POINT('',(518.,-9.76288198200727,5.29019237886467));
#89656=CARTESIAN_POINT('Origin',(518.,-9.96288198200727,4.9437822173509));
#89657=CARTESIAN_POINT('',(518.,-9.46288198200727,5.80980762113533));
#89658=CARTESIAN_POINT('Origin',(518.,-9.80929214352104,6.00980762113534));
#89659=CARTESIAN_POINT('',(518.,-9.60929214352104,6.35621778264911));
#89660=CARTESIAN_POINT('Origin',(518.,-11.0305012887935,3.26619676656571));
#89661=CARTESIAN_POINT('',(518.,-10.6441309582779,3.1626691485247));
#89662=CARTESIAN_POINT('',(518.,-10.9269736707525,3.65256709708134));
#89663=CARTESIAN_POINT('Origin',(518.,-10.5406033402369,3.54903947904033));
#89664=CARTESIAN_POINT('',(527.,-11.3901987931398,3.77668789453883));
#89665=CARTESIAN_POINT('Origin',(518.,-11.185792715855,2.68664127079227));
#89666=CARTESIAN_POINT('',(518.,-11.289320333896,2.30027094027664));
#89667=CARTESIAN_POINT('',(518.,-10.7994223853394,2.58311365275126));
#89668=CARTESIAN_POINT('Origin',(518.,-12.1586535775562,2.53320808086891));
#89669=CARTESIAN_POINT('',(527.,-11.7525454562834,2.42439173773413));
#89670=CARTESIAN_POINT('Origin',(518.,-11.5,0.300000000000001));
#89671=CARTESIAN_POINT('',(518.,-11.1,0.300000000000001));
#89672=CARTESIAN_POINT('',(518.,-11.5,0.700000000000001));
#89673=CARTESIAN_POINT('Origin',(518.,-11.1,-0.699999999999999));
#89674=CARTESIAN_POINT('',(518.,-11.1,-0.299999999999998));
#89675=CARTESIAN_POINT('Origin',(518.,-11.5,-0.299999999999998));
#89676=CARTESIAN_POINT('',(518.,-11.5,-0.699999999999999));
#89677=CARTESIAN_POINT('Origin',(518.,-11.0305012887935,-3.2661967665657));
#89678=CARTESIAN_POINT('',(518.,-10.9269736707525,-3.65256709708133));
#89679=CARTESIAN_POINT('',(518.,-10.6441309582779,-3.1626691485247));
#89680=CARTESIAN_POINT('Origin',(518.,-10.5406033402369,-3.54903947904032));
#89681=CARTESIAN_POINT('',(518.,-10.7994223853394,-2.58311365275126));
#89682=CARTESIAN_POINT('Origin',(518.,-11.185792715855,-2.68664127079226));
#89683=CARTESIAN_POINT('',(518.,-11.2893203338961,-2.30027094027664));
#89684=CARTESIAN_POINT('Origin',(518.,-10.109292143521,-5.49019237886466));
#89685=CARTESIAN_POINT('',(518.,-9.76288198200727,-5.29019237886466));
#89686=CARTESIAN_POINT('',(518.,-10.309292143521,-5.14378221735089));
#89687=CARTESIAN_POINT('Origin',(518.,-9.96288198200727,-4.94378221735089));
#89688=CARTESIAN_POINT('',(527.,-10.7246084263455,-5.38356518503845));
#89689=CARTESIAN_POINT('Origin',(518.,-9.80929214352104,-6.00980762113533));
#89690=CARTESIAN_POINT('',(518.,-9.60929214352105,-6.3562177826491));
#89691=CARTESIAN_POINT('',(518.,-9.46288198200727,-5.80980762113533));
#89692=CARTESIAN_POINT('Origin',(518.,-10.388715006927,-6.8062177826491));
#89693=CARTESIAN_POINT('',(527.,-10.0246084263455,-6.59600075033666));
#89694=CARTESIAN_POINT('Origin',(518.,-8.34386001800126,-7.91959594928933));
#89695=CARTESIAN_POINT('',(518.,-8.06101730552665,-7.63675323681471));
#89696=CARTESIAN_POINT('',(518.,-8.62670273047588,-7.63675323681471));
#89697=CARTESIAN_POINT('Origin',(518.,-7.3539105243401,-8.34386001800125));
#89698=CARTESIAN_POINT('',(518.,-7.63675323681472,-8.06101730552664));
#89699=CARTESIAN_POINT('Origin',(518.,-7.91959594928934,-8.34386001800125));
#89700=CARTESIAN_POINT('',(518.,-7.63675323681472,-8.62670273047588));
#89701=CARTESIAN_POINT('Origin',(518.,-5.49019237886467,-10.109292143521));
#89702=CARTESIAN_POINT('',(518.,-5.1437822173509,-10.309292143521));
#89703=CARTESIAN_POINT('',(518.,-5.29019237886467,-9.76288198200726));
#89704=CARTESIAN_POINT('Origin',(518.,-4.9437822173509,-9.96288198200727));
#89705=CARTESIAN_POINT('',(518.,-5.80980762113534,-9.46288198200726));
#89706=CARTESIAN_POINT('Origin',(518.,-6.00980762113534,-9.80929214352104));
#89707=CARTESIAN_POINT('',(518.,-6.35621778264911,-9.60929214352104));
#89708=CARTESIAN_POINT('Origin',(518.765685424949,0.,0.));
#89709=CARTESIAN_POINT('Origin',(518.482842712475,-5.55111512312578E-16,
0.));
#89710=CARTESIAN_POINT('Origin',(518.765685424949,0.,0.));
#89711=CARTESIAN_POINT('Origin',(518.3,0.,0.));
#89712=CARTESIAN_POINT('Origin',(518.117157287525,0.,0.));
#89713=CARTESIAN_POINT('Origin',(518.,-3.26619676656572,-11.0305012887935));
#89714=CARTESIAN_POINT('',(518.,-3.16266914852471,-10.6441309582779));
#89715=CARTESIAN_POINT('',(518.,-3.65256709708134,-10.9269736707525));
#89716=CARTESIAN_POINT('Origin',(518.,-3.54903947904034,-10.5406033402369));
#89717=CARTESIAN_POINT('',(527.,-3.77668789453883,-11.3901987931398));
#89718=CARTESIAN_POINT('Origin',(518.,-2.68664127079228,-11.185792715855));
#89719=CARTESIAN_POINT('',(518.,-2.30027094027665,-11.289320333896));
#89720=CARTESIAN_POINT('',(518.,-2.58311365275127,-10.7994223853394));
#89721=CARTESIAN_POINT('Origin',(518.,-2.53320808086892,-12.1586535775562));
#89722=CARTESIAN_POINT('',(527.,-2.42439173773414,-11.7525454562834));
#89723=CARTESIAN_POINT('Origin',(518.,-0.300000000000002,-11.5));
#89724=CARTESIAN_POINT('',(518.,-0.300000000000002,-11.1));
#89725=CARTESIAN_POINT('',(518.,-0.700000000000002,-11.5));
#89726=CARTESIAN_POINT('Origin',(518.,0.699999999999998,-11.1));
#89727=CARTESIAN_POINT('',(518.,0.299999999999998,-11.1));
#89728=CARTESIAN_POINT('Origin',(518.,0.299999999999998,-11.5));
#89729=CARTESIAN_POINT('',(518.,0.699999999999998,-11.5));
#89730=CARTESIAN_POINT('Origin',(518.,3.2661967665657,-11.0305012887935));
#89731=CARTESIAN_POINT('',(518.,3.65256709708133,-10.9269736707525));
#89732=CARTESIAN_POINT('',(518.,3.1626691485247,-10.6441309582779));
#89733=CARTESIAN_POINT('Origin',(518.,3.54903947904032,-10.5406033402369));
#89734=CARTESIAN_POINT('',(518.,2.58311365275125,-10.7994223853394));
#89735=CARTESIAN_POINT('Origin',(518.,2.68664127079226,-11.185792715855));
#89736=CARTESIAN_POINT('',(518.,2.30027094027664,-11.2893203338961));
#89737=CARTESIAN_POINT('Origin',(535.234314575051,0.,0.));
#89738=CARTESIAN_POINT('Origin',(535.234314575051,0.,0.));
#89739=CARTESIAN_POINT('Origin',(535.517157287525,0.,-2.27827821125569E-15));
#89740=CARTESIAN_POINT('Origin',(527.,0.,0.));
#89741=CARTESIAN_POINT('Origin',(518.765685424949,0.,0.));
#89742=CARTESIAN_POINT('Origin',(535.234314575051,0.,0.));
#89743=CARTESIAN_POINT('Origin',(535.234314575051,0.,0.));
#89744=CARTESIAN_POINT('Origin',(535.517157287525,-5.55111512312578E-16,
0.));
#89745=CARTESIAN_POINT('Origin',(527.,0.,0.));
#89746=CARTESIAN_POINT('Origin',(518.,5.49019237886466,-10.109292143521));
#89747=CARTESIAN_POINT('',(518.,5.29019237886466,-9.76288198200727));
#89748=CARTESIAN_POINT('',(518.,5.14378221735088,-10.309292143521));
#89749=CARTESIAN_POINT('Origin',(518.,4.94378221735088,-9.96288198200727));
#89750=CARTESIAN_POINT('',(527.,5.38356518503844,-10.7246084263456));
#89751=CARTESIAN_POINT('Origin',(518.,6.00980762113532,-9.80929214352105));
#89752=CARTESIAN_POINT('',(518.,6.3562177826491,-9.60929214352105));
#89753=CARTESIAN_POINT('',(518.,5.80980762113532,-9.46288198200727));
#89754=CARTESIAN_POINT('Origin',(518.,6.8062177826491,-10.388715006927));
#89755=CARTESIAN_POINT('',(527.,6.59600075033666,-10.0246084263456));
#89756=CARTESIAN_POINT('Origin',(518.765685424949,0.,0.));
#89757=CARTESIAN_POINT('Origin',(518.482842712475,0.,-2.2782782112557E-15));
#89758=CARTESIAN_POINT('Origin',(518.3,0.,0.));
#89759=CARTESIAN_POINT('Origin',(518.117157287525,0.,1.00115767893202E-15));
#89760=CARTESIAN_POINT('Origin',(518.765685424949,0.,0.));
#89761=CARTESIAN_POINT('Origin',(518.482842712475,5.55111512312578E-16,
-1.11022302462516E-15));
#89762=CARTESIAN_POINT('Origin',(518.3,0.,0.));
#89763=CARTESIAN_POINT('Origin',(518.117157287525,5.55111512312578E-16,
0.));
#89764=CARTESIAN_POINT('Origin',(535.6,0.,0.));
#89765=CARTESIAN_POINT('Origin',(535.6,14.1633841320521,1.41924675424547));
#89766=CARTESIAN_POINT('Origin',(535.882842712475,5.55111512312578E-16,
0.));
#89767=CARTESIAN_POINT('Origin',(535.6,-5.85258832261124,12.9754738390372));
#89768=CARTESIAN_POINT('Ctrl Pts',(536.,14.4,-7.49400541621981E-15));
#89769=CARTESIAN_POINT('Ctrl Pts',(536.,14.4,0.00443214870431098));
#89770=CARTESIAN_POINT('Ctrl Pts',(535.999996398319,14.4000012120569,0.00886355094690701));
#89771=CARTESIAN_POINT('Ctrl Pts',(535.999323213544,14.4002754442916,0.499523265098869));
#89772=CARTESIAN_POINT('Ctrl Pts',(535.958538851494,14.4152915483467,0.982908245004447));
#89773=CARTESIAN_POINT('Ctrl Pts',(535.88284271243,14.4448174223773,1.44744787340554));
#89774=CARTESIAN_POINT('Ctrl Pts',(536.,14.4,-7.49400541621981E-15));
#89775=CARTESIAN_POINT('Ctrl Pts',(535.999989114725,14.3996961036921,0.00435706973747238));
#89776=CARTESIAN_POINT('Ctrl Pts',(536.000009671027,14.3993917043225,0.00874191430361652));
#89777=CARTESIAN_POINT('Ctrl Pts',(535.999419832006,14.3659794521317,0.491855343046162));
#89778=CARTESIAN_POINT('Ctrl Pts',(535.987158077032,14.3474420887423,0.971514735757601));
#89779=CARTESIAN_POINT('Ctrl Pts',(535.956890761426,14.3711383592723,1.44006483767503));
#89780=CARTESIAN_POINT('Ctrl Pts',(536.,14.4,-7.49400541621981E-15));
#89781=CARTESIAN_POINT('Ctrl Pts',(536.,14.3993908437431,0.00429837984413543));
#89782=CARTESIAN_POINT('Ctrl Pts',(536.,14.3987831887276,0.00860412071986771));
#89783=CARTESIAN_POINT('Ctrl Pts',(535.999999999999,14.3316957191485,0.484660136504454));
#89784=CARTESIAN_POINT('Ctrl Pts',(536.,14.2788648366151,0.95900379733823));
#89785=CARTESIAN_POINT('Ctrl Pts',(536.,14.2675820623746,1.42968794350869));
#89786=CARTESIAN_POINT('Ctrl Pts',(536.,14.4,-7.49400541621981E-15));
#89787=CARTESIAN_POINT('Ctrl Pts',(536.,14.3990866209829,0.00423516432177781));
#89788=CARTESIAN_POINT('Ctrl Pts',(536.,14.3981740098758,0.00847050495900394));
#89789=CARTESIAN_POINT('Ctrl Pts',(535.999999999999,14.2973869261308,0.4773765220558));
#89790=CARTESIAN_POINT('Ctrl Pts',(536.,14.210772825194,0.946330918549924));
#89791=CARTESIAN_POINT('Ctrl Pts',(536.,14.1633841320521,1.41924675424546));
#89792=CARTESIAN_POINT('Ctrl Pts',(535.88284271243,-5.96888208216603,13.2333027775094));
#89793=CARTESIAN_POINT('Ctrl Pts',(535.95853884256,-6.35642221867374,12.9754628367592));
#89794=CARTESIAN_POINT('Ctrl Pts',(535.999323210363,-6.76753777932651,12.7207660541882));
#89795=CARTESIAN_POINT('Ctrl Pts',(535.999996398191,-7.19232444631968,12.4751986970763));
#89796=CARTESIAN_POINT('Ctrl Pts',(536.,-7.19616159686892,12.4729819175769));
#89797=CARTESIAN_POINT('Ctrl Pts',(536.,-7.2,12.4707658144959));
#89798=CARTESIAN_POINT('Ctrl Pts',(535.956890761426,-5.93843644711319,13.1658033192681));
#89799=CARTESIAN_POINT('Ctrl Pts',(535.987020238062,-6.33187599931295,12.9108800111187));
#89800=CARTESIAN_POINT('Ctrl Pts',(535.999610153754,-6.75686986112659,12.6872975364447));
#89801=CARTESIAN_POINT('Ctrl Pts',(535.999999818284,-7.19213281099715,12.4746061969206));
#89802=CARTESIAN_POINT('Ctrl Pts',(536.,-7.19606623028845,12.4726854131806));
#89803=CARTESIAN_POINT('Ctrl Pts',(536.,-7.2,12.4707658144959));
#89804=CARTESIAN_POINT('Ctrl Pts',(536.,-5.89564495262476,13.0709324883497));
#89805=CARTESIAN_POINT('Ctrl Pts',(535.999439468893,-6.30871501018977,12.8452020184884));
#89806=CARTESIAN_POINT('Ctrl Pts',(535.999956364857,-6.74608206403723,12.6539602383552));
#89807=CARTESIAN_POINT('Ctrl Pts',(536.000000244009,-7.19194194870236,12.4740128582116));
#89808=CARTESIAN_POINT('Ctrl Pts',(536.,-7.19597086370798,12.4723889087843));
#89809=CARTESIAN_POINT('Ctrl Pts',(536.,-7.2,12.4707658144959));
#89810=CARTESIAN_POINT('Ctrl Pts',(536.,-5.8525883226112,12.9754738390371));
#89811=CARTESIAN_POINT('Ctrl Pts',(536.,-6.28583974561473,12.7800557563653));
#89812=CARTESIAN_POINT('Ctrl Pts',(536.,-6.73527316506757,12.6205885930199));
#89813=CARTESIAN_POINT('Ctrl Pts',(536.,-7.19175122552344,12.4734197474849));
#89814=CARTESIAN_POINT('Ctrl Pts',(536.,-7.1958754971275,12.472092404388));
#89815=CARTESIAN_POINT('Ctrl Pts',(536.,-7.2,12.4707658144959));
#89816=CARTESIAN_POINT('Origin',(535.6,0.,0.));
#89817=CARTESIAN_POINT('Origin',(535.6,-5.85258832261126,-12.9754738390371));
#89818=CARTESIAN_POINT('Origin',(535.882842712475,0.,0.));
#89819=CARTESIAN_POINT('Origin',(535.6,14.1633841320522,-1.419246754245));
#89820=CARTESIAN_POINT('Ctrl Pts',(536.,-7.20000000000006,-12.4707658144959));
#89821=CARTESIAN_POINT('Ctrl Pts',(536.,-7.1961616466213,-12.4729818888524));
#89822=CARTESIAN_POINT('Ctrl Pts',(535.99999639828,-7.19232454578704,-12.4751986396123));
#89823=CARTESIAN_POINT('Ctrl Pts',(535.99932321985,-6.76753787666127,-12.7207659938899));
#89824=CARTESIAN_POINT('Ctrl Pts',(535.958538851494,-6.35642226441094,-12.9754628063292));
#89825=CARTESIAN_POINT('Ctrl Pts',(535.88284271243,-5.96888208216605,-13.2333027775094));
#89826=CARTESIAN_POINT('Ctrl Pts',(536.,-7.20000000000006,-12.4707658144959));
#89827=CARTESIAN_POINT('Ctrl Pts',(535.999989114725,-7.19607471875817,-12.4726811674377));
#89828=CARTESIAN_POINT('Ctrl Pts',(536.000009670988,-7.19212513234199,-12.4746099721072));
#89829=CARTESIAN_POINT('Ctrl Pts',(535.999419838313,-6.75703049587399,-12.6872308324062));
#89830=CARTESIAN_POINT('Ctrl Pts',(535.987158077033,-6.3323646030542,-12.9110066960544));
#89831=CARTESIAN_POINT('Ctrl Pts',(535.956890761426,-5.93843644711321,-13.1658033192681));
#89832=CARTESIAN_POINT('Ctrl Pts',(536.,-7.20000000000006,-12.4707658144959));
#89833=CARTESIAN_POINT('Ctrl Pts',(536.,-7.19597291572316,-12.4723874596152));
#89834=CARTESIAN_POINT('Ctrl Pts',(536.,-7.19194020721408,-12.4740140853249));
#89835=CARTESIAN_POINT('Ctrl Pts',(535.999999999986,-6.74611987252778,-12.6539426485665));
#89836=CARTESIAN_POINT('Ctrl Pts',(536.,-6.30891076748819,-12.8453615843829));
#89837=CARTESIAN_POINT('Ctrl Pts',(536.,-5.89564495262477,-13.0709324883497));
#89838=CARTESIAN_POINT('Ctrl Pts',(536.,-7.20000000000006,-12.4707658144959));
#89839=CARTESIAN_POINT('Ctrl Pts',(536.,-7.19587555058959,-12.4720923872068));
#89840=CARTESIAN_POINT('Ctrl Pts',(536.,-7.19175133243048,-12.4734197130817));
#89841=CARTESIAN_POINT('Ctrl Pts',(535.999999999986,-6.73527327116365,-12.6205885550169));
#89842=CARTESIAN_POINT('Ctrl Pts',(536.,-6.28583979674674,-12.7800557333022));
#89843=CARTESIAN_POINT('Ctrl Pts',(536.,-5.85258832261122,-12.9754738390371));
#89844=CARTESIAN_POINT('Ctrl Pts',(535.88284271243,14.4448174223773,-1.44744787340509));
#89845=CARTESIAN_POINT('Ctrl Pts',(535.95853884256,14.4152915518313,-0.982908299828289));
#89846=CARTESIAN_POINT('Ctrl Pts',(535.999323204044,14.400275447844,-0.49952337916368));
#89847=CARTESIAN_POINT('Ctrl Pts',(535.99999639823,14.4000012120886,-0.00886366582987818));
#89848=CARTESIAN_POINT('Ctrl Pts',(536.,14.4,-0.00443220616197399));
#89849=CARTESIAN_POINT('Ctrl Pts',(536.,14.4,-4.71844785465692E-15));
#89850=CARTESIAN_POINT('Ctrl Pts',(535.956890761426,14.3711383592723,-1.44006483767457));
#89851=CARTESIAN_POINT('Ctrl Pts',(535.987020238062,14.347088074498,-0.971874536541306));
#89852=CARTESIAN_POINT('Ctrl Pts',(535.999610150543,14.3659568909306,-0.492027825466466));
#89853=CARTESIAN_POINT('Ctrl Pts',(535.999999818304,14.3993922743092,-0.00873337670539355));
#89854=CARTESIAN_POINT('Ctrl Pts',(536.,14.3996955363702,-0.00436654384518595));
#89855=CARTESIAN_POINT('Ctrl Pts',(536.,14.4,-4.71844785465692E-15));
#89856=CARTESIAN_POINT('Ctrl Pts',(536.,14.2675820623746,-1.42968794350823));
#89857=CARTESIAN_POINT('Ctrl Pts',(535.999439468893,14.278628769849,-0.959093545183618));
#89858=CARTESIAN_POINT('Ctrl Pts',(535.999956346761,14.3316920411956,-0.484701678326892));
#89859=CARTESIAN_POINT('Ctrl Pts',(536.00000024412,14.398782996792,-0.00860199897387956));
#89860=CARTESIAN_POINT('Ctrl Pts',(536.,14.3993910727405,-0.00430088152839791));
#89861=CARTESIAN_POINT('Ctrl Pts',(536.,14.4,-4.71844785465692E-15));
#89862=CARTESIAN_POINT('Ctrl Pts',(536.,14.1633841320521,-1.41924675424501));
#89863=CARTESIAN_POINT('Ctrl Pts',(536.,14.2107728196014,-0.946330974362331));
#89864=CARTESIAN_POINT('Ctrl Pts',(536.000000000003,14.297386906149,-0.477376632577604));
#89865=CARTESIAN_POINT('Ctrl Pts',(536.,14.3981739862025,-0.00847061475408605));
#89866=CARTESIAN_POINT('Ctrl Pts',(536.,14.3990866091107,-0.00423521921160987));
#89867=CARTESIAN_POINT('Ctrl Pts',(536.,14.4,-4.71844785465692E-15));
#89868=CARTESIAN_POINT('Origin',(535.6,0.,0.));
#89869=CARTESIAN_POINT('Origin',(535.6,-8.31079580944086,11.5562270847921));
#89870=CARTESIAN_POINT('Origin',(535.882842712475,0.,1.00115767893202E-15));
#89871=CARTESIAN_POINT('Origin',(535.6,-8.31079580944088,-11.5562270847921));
#89872=CARTESIAN_POINT('Ctrl Pts',(536.,-7.20000000000002,12.4707658144959));
#89873=CARTESIAN_POINT('Ctrl Pts',(536.,-7.20383835337878,12.4685497401394));
#89874=CARTESIAN_POINT('Ctrl Pts',(535.999996398286,-7.2076766662638,12.4663350887228));
#89875=CARTESIAN_POINT('Ctrl Pts',(535.999323218915,-7.63273756686728,12.221242719787));
#89876=CARTESIAN_POINT('Ctrl Pts',(535.958538851494,-8.05886928393568,11.9925545613255));
#89877=CARTESIAN_POINT('Ctrl Pts',(535.88284271243,-8.4759353402112,11.7858549041043));
#89878=CARTESIAN_POINT('Ctrl Pts',(536.,-7.20000000000002,12.4707658144959));
#89879=CARTESIAN_POINT('Ctrl Pts',(535.999989114725,-7.20362138492575,12.4683240976943));
#89880=CARTESIAN_POINT('Ctrl Pts',(536.000009670994,-7.20726657197257,12.465868057861));
#89881=CARTESIAN_POINT('Ctrl Pts',(535.999419837377,-7.60894895549618,12.1953754803564));
#89882=CARTESIAN_POINT('Ctrl Pts',(535.987158077033,-8.0150774856869,11.9394919602974));
#89883=CARTESIAN_POINT('Ctrl Pts',(535.956890761426,-8.43270191215901,11.7257384815935));
#89884=CARTESIAN_POINT('Ctrl Pts',(536.,-7.20000000000002,12.4707658144959));
#89885=CARTESIAN_POINT('Ctrl Pts',(536.,-7.20341792800768,12.4680890797686));
#89886=CARTESIAN_POINT('Ctrl Pts',(536.,-7.2068429814443,12.4654099646239));
#89887=CARTESIAN_POINT('Ctrl Pts',(536.000000000004,-7.58557585475362,12.1692825096895));
#89888=CARTESIAN_POINT('Ctrl Pts',(536.,-7.96995406912831,11.8863577870457));
#89889=CARTESIAN_POINT('Ctrl Pts',(536.,-8.37193710974973,11.6412445448415));
#89890=CARTESIAN_POINT('Ctrl Pts',(536.,-7.20000000000002,12.4707658144959));
#89891=CARTESIAN_POINT('Ctrl Pts',(536.,-7.20321107037281,12.4678572228852));
#89892=CARTESIAN_POINT('Ctrl Pts',(536.,-7.20642267737424,12.4649492081416));
#89893=CARTESIAN_POINT('Ctrl Pts',(536.000000000004,-7.56211366310163,12.1432120305888));
#89894=CARTESIAN_POINT('Ctrl Pts',(536.,-7.9249330284473,11.8337248147531));
#89895=CARTESIAN_POINT('Ctrl Pts',(536.,-8.31079580944085,11.5562270847921));
#89896=CARTESIAN_POINT('Ctrl Pts',(535.88284271243,-8.47593534021121,-11.7858549041042));
#89897=CARTESIAN_POINT('Ctrl Pts',(535.95853884256,-8.05886933315749,-11.9925545369309));
#89898=CARTESIAN_POINT('Ctrl Pts',(535.999323209414,-7.63273766741671,-12.2212426658364));
#89899=CARTESIAN_POINT('Ctrl Pts',(535.999996398197,-7.20767676578349,-12.4663350313016));
#89900=CARTESIAN_POINT('Ctrl Pts',(536.,-7.20383840313102,-12.468549711415));
#89901=CARTESIAN_POINT('Ctrl Pts',(536.,-7.2,-12.4707658144959));
#89902=CARTESIAN_POINT('Ctrl Pts',(535.956890761426,-8.43270191215902,-11.7257384815935));
#89903=CARTESIAN_POINT('Ctrl Pts',(535.987020238062,-8.01521207518498,-11.9390054745774));
#89904=CARTESIAN_POINT('Ctrl Pts',(535.999610153273,-7.6090870413046,-12.1952697160563));
#89905=CARTESIAN_POINT('Ctrl Pts',(535.999999818287,-7.20725946324932,-12.4658728201825));
#89906=CARTESIAN_POINT('Ctrl Pts',(536.,-7.20362930608181,-12.4683188693355));
#89907=CARTESIAN_POINT('Ctrl Pts',(536.,-7.2,-12.4707658144959));
#89908=CARTESIAN_POINT('Ctrl Pts',(536.,-8.37193710974974,-11.6412445448415));
#89909=CARTESIAN_POINT('Ctrl Pts',(535.999439468893,-7.9699137596592,-11.8861084733048));
#89910=CARTESIAN_POINT('Ctrl Pts',(535.999956362134,-7.58560999192519,-12.1692585604787));
#89911=CARTESIAN_POINT('Ctrl Pts',(536.000000244026,-7.20684104800673,-12.4654108592329));
#89912=CARTESIAN_POINT('Ctrl Pts',(536.,-7.2034202090326,-12.4680880272561));
#89913=CARTESIAN_POINT('Ctrl Pts',(536.,-7.2,-12.4707658144959));
#89914=CARTESIAN_POINT('Ctrl Pts',(536.,-8.31079580944087,-11.5562270847921));
#89915=CARTESIAN_POINT('Ctrl Pts',(536.,-7.92493307398652,-11.833724782003));
#89916=CARTESIAN_POINT('Ctrl Pts',(536.000000000003,-7.56211374877667,-12.1432119579598));
#89917=CARTESIAN_POINT('Ctrl Pts',(536.,-7.20642276063924,-12.4649491327435));
#89918=CARTESIAN_POINT('Ctrl Pts',(536.,-7.20321111198339,-12.4678571851766));
#89919=CARTESIAN_POINT('Ctrl Pts',(536.,-7.2,-12.4707658144959));
#89920=CARTESIAN_POINT('Origin',(535.7,0.,0.));
#89921=CARTESIAN_POINT('Origin',(535.7,0.,0.));
#89922=CARTESIAN_POINT('Origin',(518.,7.91959594928933,-8.34386001800126));
#89923=CARTESIAN_POINT('',(518.,7.63675323681471,-8.06101730552664));
#89924=CARTESIAN_POINT('',(518.,7.63675323681471,-8.62670273047588));
#89925=CARTESIAN_POINT('Origin',(518.,8.34386001800126,-7.35391052434009));
#89926=CARTESIAN_POINT('',(518.,8.06101730552664,-7.63675323681472));
#89927=CARTESIAN_POINT('Origin',(518.,8.34386001800126,-7.91959594928933));
#89928=CARTESIAN_POINT('',(518.,8.62670273047588,-7.63675323681471));
#89929=CARTESIAN_POINT('Origin',(518.,10.109292143521,-5.49019237886467));
#89930=CARTESIAN_POINT('',(518.,10.309292143521,-5.1437822173509));
#89931=CARTESIAN_POINT('',(518.,9.76288198200726,-5.29019237886467));
#89932=CARTESIAN_POINT('Origin',(518.,11.088715006927,-5.5937822173509));
#89933=CARTESIAN_POINT('',(527.,10.7246084263455,-5.38356518503846));
#89934=CARTESIAN_POINT('Origin',(518.,9.80929214352104,-6.00980762113534));
#89935=CARTESIAN_POINT('',(518.,9.46288198200726,-5.80980762113534));
#89936=CARTESIAN_POINT('',(518.,9.60929214352104,-6.35621778264911));
#89937=CARTESIAN_POINT('Origin',(518.,9.26288198200726,-6.15621778264911));
#89938=CARTESIAN_POINT('',(527.,10.0246084263455,-6.59600075033667));
#89939=CARTESIAN_POINT('Origin',(518.4,0.,0.));
#89940=CARTESIAN_POINT('Origin',(518.4,14.1633841320522,1.41924675424466));
#89941=CARTESIAN_POINT('Origin',(518.4,-5.85258832261145,12.9754738390371));
#89942=CARTESIAN_POINT('Ctrl Pts',(518.11715728757,14.4448174223773,1.4474478734047));
#89943=CARTESIAN_POINT('Ctrl Pts',(518.041461163612,14.4152915542388,0.982908337704882));
#89944=CARTESIAN_POINT('Ctrl Pts',(518.000676801706,14.4002754503427,0.49952345888792));
#89945=CARTESIAN_POINT('Ctrl Pts',(518.000003601837,14.4000012121102,0.00886374519088989));
#89946=CARTESIAN_POINT('Ctrl Pts',(518.,14.4000000000001,0.00443224585609561));
#89947=CARTESIAN_POINT('Ctrl Pts',(518.,14.4000000000001,3.05311331771918E-15));
#89948=CARTESIAN_POINT('Ctrl Pts',(518.043109238574,14.3711383592723,1.44006483767419));
#89949=CARTESIAN_POINT('Ctrl Pts',(518.012979764394,14.347088076459,0.971874574715578));
#89950=CARTESIAN_POINT('Ctrl Pts',(518.000389851206,14.3659568894899,0.492027902208947));
#89951=CARTESIAN_POINT('Ctrl Pts',(518.00000018171,14.3993922688672,0.00873345491462824));
#89952=CARTESIAN_POINT('Ctrl Pts',(518.,14.3996955336412,0.00436658295017734));
#89953=CARTESIAN_POINT('Ctrl Pts',(518.,14.4000000000001,3.05311331771918E-15));
#89954=CARTESIAN_POINT('Ctrl Pts',(518.,14.2675820623746,1.42968794350786));
#89955=CARTESIAN_POINT('Ctrl Pts',(518.000560531062,14.2786287689483,0.959093583553918));
#89956=CARTESIAN_POINT('Ctrl Pts',(518.000043650911,14.3316920348535,0.484701754815541));
#89957=CARTESIAN_POINT('Ctrl Pts',(517.999999755893,14.398782985889,0.00860207600473767));
#89958=CARTESIAN_POINT('Ctrl Pts',(518.,14.3993910672824,0.00430092004425908));
#89959=CARTESIAN_POINT('Ctrl Pts',(518.,14.4000000000001,3.05311331771918E-15));
#89960=CARTESIAN_POINT('Ctrl Pts',(518.,14.1633841320521,1.41924675424464));
#89961=CARTESIAN_POINT('Ctrl Pts',(518.,14.2107728157373,0.946331012921918));
#89962=CARTESIAN_POINT('Ctrl Pts',(518.000000000002,14.2973868934641,0.477376708780995));
#89963=CARTESIAN_POINT('Ctrl Pts',(518.,14.3981739698498,0.00847069060670547));
#89964=CARTESIAN_POINT('Ctrl Pts',(518.,14.3990866009235,0.00423525713834081));
#89965=CARTESIAN_POINT('Ctrl Pts',(518.,14.4000000000001,3.05311331771918E-15));
#89966=CARTESIAN_POINT('Ctrl Pts',(518.,-7.20000000000001,12.470765814496));
#89967=CARTESIAN_POINT('Ctrl Pts',(518.,-7.19616161176896,12.4729819089744));
#89968=CARTESIAN_POINT('Ctrl Pts',(518.000003601789,-7.19232447611272,12.475198679864));
#89969=CARTESIAN_POINT('Ctrl Pts',(518.000676785755,-6.76753780733218,12.7207660368554));
#89970=CARTESIAN_POINT('Ctrl Pts',(518.041461154763,-6.35642223237711,12.9754628276421));
#89971=CARTESIAN_POINT('Ctrl Pts',(518.11715728757,-5.96888208216626,13.2333027775093));
#89972=CARTESIAN_POINT('Ctrl Pts',(518.,-7.20000000000001,12.470765814496));
#89973=CARTESIAN_POINT('Ctrl Pts',(518.000010885289,-7.19607468304915,12.4726811848558));
#89974=CARTESIAN_POINT('Ctrl Pts',(517.999990329019,-7.19212506091541,12.474610006982));
#89975=CARTESIAN_POINT('Ctrl Pts',(518.000580162732,-6.75703042442209,12.6872308702133));
#89976=CARTESIAN_POINT('Ctrl Pts',(518.012841925383,-6.33236457042605,12.9110067171452));
#89977=CARTESIAN_POINT('Ctrl Pts',(518.043109238574,-5.93843644711342,13.1658033192681));
#89978=CARTESIAN_POINT('Ctrl Pts',(518.,-7.20000000000001,12.470765814496));
#89979=CARTESIAN_POINT('Ctrl Pts',(518.,-7.19597287913992,12.4723874743366));
#89980=CARTESIAN_POINT('Ctrl Pts',(518.,-7.19194013404502,12.4740141147993));
#89981=CARTESIAN_POINT('Ctrl Pts',(518.000000000003,-6.74611980107996,12.653942681858));
#89982=CARTESIAN_POINT('Ctrl Pts',(518.,-6.30891073331362,12.845361603042));
#89983=CARTESIAN_POINT('Ctrl Pts',(518.,-5.89564495262499,13.0709324883496));
#89984=CARTESIAN_POINT('Ctrl Pts',(518.,-7.20000000000001,12.470765814496));
#89985=CARTESIAN_POINT('Ctrl Pts',(518.,-7.19587551313739,12.4720923992309));
#89986=CARTESIAN_POINT('Ctrl Pts',(518.,-7.19175125752897,12.4734197371684));
#89987=CARTESIAN_POINT('Ctrl Pts',(518.000000000003,-6.73527319767247,12.6205885830549));
#89988=CARTESIAN_POINT('Ctrl Pts',(518.,-6.28583976093444,12.7800557494554));
#89989=CARTESIAN_POINT('Ctrl Pts',(518.,-5.85258832261145,12.975473839037));
#89990=CARTESIAN_POINT('Origin',(518.4,0.,0.));
#89991=CARTESIAN_POINT('Origin',(518.4,-5.85258832261171,-12.9754738390369));
#89992=CARTESIAN_POINT('Origin',(518.4,14.1633841320522,-1.41924675424485));
#89993=CARTESIAN_POINT('Ctrl Pts',(518.11715728757,-5.9688820821665,-13.2333027775091));
#89994=CARTESIAN_POINT('Ctrl Pts',(518.041432655893,-6.35656813753688,-12.9753657533672));
#89995=CARTESIAN_POINT('Ctrl Pts',(518.000677557365,-6.76744956600245,-12.7208173836523));
#89996=CARTESIAN_POINT('Ctrl Pts',(518.000003599129,-7.19232392599177,-12.4751989959597));
#89997=CARTESIAN_POINT('Ctrl Pts',(518.,-7.19616156249294,-12.472981937424));
#89998=CARTESIAN_POINT('Ctrl Pts',(518.,-7.20000000000004,-12.470765814496));
#89999=CARTESIAN_POINT('Ctrl Pts',(518.043109238574,-5.93843644711366,-13.1658033192679));
#90000=CARTESIAN_POINT('Ctrl Pts',(518.012968417412,-6.33202413945791,-12.9107840259143));
#90001=CARTESIAN_POINT('Ctrl Pts',(518.000390350054,-6.7567797810577,-12.6873431349195));
#90002=CARTESIAN_POINT('Ctrl Pts',(518.000000179606,-7.19213227583273,-12.4746064486523));
#90003=CARTESIAN_POINT('Ctrl Pts',(518.,-7.19606619505814,-12.4726854303698));
#90004=CARTESIAN_POINT('Ctrl Pts',(518.,-7.20000000000004,-12.470765814496));
#90005=CARTESIAN_POINT('Ctrl Pts',(518.,-5.89564495262524,-13.0709324883495));
#90006=CARTESIAN_POINT('Ctrl Pts',(518.000560742162,-6.30887054172597,-12.8451170251414));
#90007=CARTESIAN_POINT('Ctrl Pts',(518.000043603454,-6.74598950673795,-12.6539990699213));
#90008=CARTESIAN_POINT('Ctrl Pts',(517.999999756269,-7.19194140227681,-12.4740130696039));
#90009=CARTESIAN_POINT('Ctrl Pts',(518.,-7.19597082762334,-12.4723889233156));
#90010=CARTESIAN_POINT('Ctrl Pts',(518.,-7.20000000000004,-12.470765814496));
#90011=CARTESIAN_POINT('Ctrl Pts',(518.,-5.8525883226117,-12.9754738390369));
#90012=CARTESIAN_POINT('Ctrl Pts',(518.,-6.28600287595523,-12.7799821764146));
#90013=CARTESIAN_POINT('Ctrl Pts',(518.000000000003,-6.73517810085928,-12.6206205967494));
#90014=CARTESIAN_POINT('Ctrl Pts',(518.,-7.19175066797431,-12.4734199188406));
#90015=CARTESIAN_POINT('Ctrl Pts',(518.,-7.19587546018855,-12.4720924162615));
#90016=CARTESIAN_POINT('Ctrl Pts',(518.,-7.20000000000004,-12.470765814496));
#90017=CARTESIAN_POINT('Ctrl Pts',(518.,14.4000000000001,-1.94289029309402E-15));
#90018=CARTESIAN_POINT('Ctrl Pts',(518.,14.4000000000001,-0.00443218895692105));
#90019=CARTESIAN_POINT('Ctrl Pts',(518.000003601749,14.4000012120789,-0.00886363141148958));
#90020=CARTESIAN_POINT('Ctrl Pts',(518.00067679229,14.4002754468243,-0.499523345966166));
#90021=CARTESIAN_POINT('Ctrl Pts',(518.041461154763,14.4152915507873,-0.982908283402282));
#90022=CARTESIAN_POINT('Ctrl Pts',(518.11715728757,14.4448174223773,-1.4474478734049));
#90023=CARTESIAN_POINT('Ctrl Pts',(518.,14.4000000000001,-1.94289029309402E-15));
#90024=CARTESIAN_POINT('Ctrl Pts',(518.000010885289,14.399696100914,-0.00435710937729983));
#90025=CARTESIAN_POINT('Ctrl Pts',(517.999990328979,14.3993916988099,-0.00874199359722324));
#90026=CARTESIAN_POINT('Ctrl Pts',(518.000580169267,14.365979449137,-0.491855423172552));
#90027=CARTESIAN_POINT('Ctrl Pts',(518.012841925383,14.3474420906923,-0.971514774559103));
#90028=CARTESIAN_POINT('Ctrl Pts',(518.043109238574,14.3711383592723,-1.44006483767439));
#90029=CARTESIAN_POINT('Ctrl Pts',(518.,14.4000000000001,-1.94289029309402E-15));
#90030=CARTESIAN_POINT('Ctrl Pts',(518.,14.3993908381882,-0.00429841888924513));
#90031=CARTESIAN_POINT('Ctrl Pts',(518.,14.398783177661,-0.0086041988206578));
#90032=CARTESIAN_POINT('Ctrl Pts',(517.999999999997,14.3316957120973,-0.484660214671882));
#90033=CARTESIAN_POINT('Ctrl Pts',(518.,14.2788648356883,-0.95900383626306));
#90034=CARTESIAN_POINT('Ctrl Pts',(518.,14.2675820623746,-1.42968794350805));
#90035=CARTESIAN_POINT('Ctrl Pts',(518.,14.4000000000001,-1.94289029309402E-15));
#90036=CARTESIAN_POINT('Ctrl Pts',(518.,14.3990866126494,-0.00423520276807552));
#90037=CARTESIAN_POINT('Ctrl Pts',(518.,14.3981739932752,-0.00847058186628403));
#90038=CARTESIAN_POINT('Ctrl Pts',(517.999999999997,14.2973869135097,-0.477376599365992));
#90039=CARTESIAN_POINT('Ctrl Pts',(518.,14.210772821277,-0.946330957640153));
#90040=CARTESIAN_POINT('Ctrl Pts',(518.,14.1633841320522,-1.41924675424483));
#90041=CARTESIAN_POINT('Origin',(518.4,0.,0.));
#90042=CARTESIAN_POINT('Origin',(518.4,-8.31079580944094,11.5562270847921));
#90043=CARTESIAN_POINT('Origin',(518.4,-8.31079580944076,-11.5562270847922));
#90044=CARTESIAN_POINT('Ctrl Pts',(518.11715728757,-8.47593534021129,11.7858549041043));
#90045=CARTESIAN_POINT('Ctrl Pts',(518.041461163612,-8.05886936716401,11.9925545200772));
#90046=CARTESIAN_POINT('Ctrl Pts',(518.000676796169,-7.63273773832444,12.2212426277938));
#90047=CARTESIAN_POINT('Ctrl Pts',(518.000003601871,-7.20767683450791,12.4663349916484));
#90048=CARTESIAN_POINT('Ctrl Pts',(518.,-7.20383843749968,12.4685496915723));
#90049=CARTESIAN_POINT('Ctrl Pts',(518.,-7.20000000000003,12.470765814496));
#90050=CARTESIAN_POINT('Ctrl Pts',(518.043109238574,-8.43270191215911,11.7257384815936));
#90051=CARTESIAN_POINT('Ctrl Pts',(518.012979764394,-8.01521210922605,11.9390054571882));
#90052=CARTESIAN_POINT('Ctrl Pts',(518.00038984839,-7.60908710738131,12.1952696765398));
#90053=CARTESIAN_POINT('Ctrl Pts',(518.000000181728,-7.20725952824866,12.4658727763748));
#90054=CARTESIAN_POINT('Ctrl Pts',(518.,-7.20362933858175,12.4683188474284));
#90055=CARTESIAN_POINT('Ctrl Pts',(518.,-7.20000000000003,12.470765814496));
#90056=CARTESIAN_POINT('Ctrl Pts',(518.,-8.37193710974981,11.6412445448415));
#90057=CARTESIAN_POINT('Ctrl Pts',(518.000560531062,-7.96991379243915,11.8861084533393));
#90058=CARTESIAN_POINT('Ctrl Pts',(518.000043635046,-7.58561005545744,12.169258516837));
#90059=CARTESIAN_POINT('Ctrl Pts',(517.99999975599,-7.20684110925685,12.4654108112892));
#90060=CARTESIAN_POINT('Ctrl Pts',(518.,-7.20342023966382,12.4680880032846));
#90061=CARTESIAN_POINT('Ctrl Pts',(518.,-7.20000000000003,12.470765814496));
#90062=CARTESIAN_POINT('Ctrl Pts',(518.,-8.31079580944093,11.5562270847921));
#90063=CARTESIAN_POINT('Ctrl Pts',(518.,-7.92493310544876,11.8337247593766));
#90064=CARTESIAN_POINT('Ctrl Pts',(518.000000000001,-7.56211380885965,12.1432119087018));
#90065=CARTESIAN_POINT('Ctrl Pts',(518.,-7.20642281814689,12.464949080675));
#90066=CARTESIAN_POINT('Ctrl Pts',(518.,-7.20321114074589,12.4678571591407));
#90067=CARTESIAN_POINT('Ctrl Pts',(518.,-7.20000000000003,12.470765814496));
#90068=CARTESIAN_POINT('Ctrl Pts',(518.,-7.20000000000004,-12.470765814496));
#90069=CARTESIAN_POINT('Ctrl Pts',(518.,-7.20383838823105,-12.4685497200175));
#90070=CARTESIAN_POINT('Ctrl Pts',(518.000003601783,-7.20767673596133,-12.4663350485081));
#90071=CARTESIAN_POINT('Ctrl Pts',(518.000676786757,-7.63273763852262,-12.2212426813519));
#90072=CARTESIAN_POINT('Ctrl Pts',(518.041461154763,-8.05886931841019,-11.9925545442398));
#90073=CARTESIAN_POINT('Ctrl Pts',(518.11715728757,-8.47593534021109,-11.7858549041044));
#90074=CARTESIAN_POINT('Ctrl Pts',(518.,-7.20000000000004,-12.470765814496));
#90075=CARTESIAN_POINT('Ctrl Pts',(518.000010885289,-7.20362141786473,-12.4683240754786));
#90076=CARTESIAN_POINT('Ctrl Pts',(517.999990329013,-7.20726663788961,-12.4658680134404));
#90077=CARTESIAN_POINT('Ctrl Pts',(518.000580163734,-7.60894902374548,-12.1953754375035));
#90078=CARTESIAN_POINT('Ctrl Pts',(518.012841925383,-8.01507752026624,-11.9394919425861));
#90079=CARTESIAN_POINT('Ctrl Pts',(518.043109238574,-8.43270191215891,-11.7257384815937));
#90080=CARTESIAN_POINT('Ctrl Pts',(518.,-7.20000000000004,-12.470765814496));
#90081=CARTESIAN_POINT('Ctrl Pts',(518.,-7.20341795904844,-12.4680890554475));
#90082=CARTESIAN_POINT('Ctrl Pts',(518.,-7.20684304355558,-12.4654099159946));
#90083=CARTESIAN_POINT('Ctrl Pts',(517.999999999999,-7.58557591913735,-12.1692824645249));
#90084=CARTESIAN_POINT('Ctrl Pts',(518.,-7.96995410237473,-11.8863577667789));
#90085=CARTESIAN_POINT('Ctrl Pts',(518.,-8.37193710974962,-11.6412445448416));
#90086=CARTESIAN_POINT('Ctrl Pts',(518.,-7.20000000000004,-12.470765814496));
#90087=CARTESIAN_POINT('Ctrl Pts',(518.,-7.20321109951219,-12.467857196463));
#90088=CARTESIAN_POINT('Ctrl Pts',(518.,-7.20642273568582,-12.4649491553181));
#90089=CARTESIAN_POINT('Ctrl Pts',(517.999999999999,-7.56211372395728,-12.1432119810277));
#90090=CARTESIAN_POINT('Ctrl Pts',(518.,-7.92493306034251,-11.8337247918152));
#90091=CARTESIAN_POINT('Ctrl Pts',(518.,-8.31079580944073,-11.5562270847922));
#90092=CARTESIAN_POINT('Origin',(518.,11.0305012887935,-3.26619676656572));
#90093=CARTESIAN_POINT('',(518.,10.6441309582779,-3.16266914852471));
#90094=CARTESIAN_POINT('',(518.,10.9269736707525,-3.65256709708134));
#90095=CARTESIAN_POINT('Origin',(518.,10.9029500033804,-2.19674332223564));
#90096=CARTESIAN_POINT('',(518.,10.7994223853394,-2.58311365275127));
#90097=CARTESIAN_POINT('Origin',(518.,11.185792715855,-2.68664127079228));
#90098=CARTESIAN_POINT('',(518.,11.289320333896,-2.30027094027665));
#90099=CARTESIAN_POINT('Origin',(518.,12.1586535775562,-2.53320808086892));
#90100=CARTESIAN_POINT('',(527.,11.7525454562834,-2.42439173773414));
#90101=CARTESIAN_POINT('Origin',(518.,10.5406033402369,-3.54903947904034));
#90102=CARTESIAN_POINT('',(527.,11.3901987931398,-3.77668789453883));
#90103=CARTESIAN_POINT('Origin',(527.,0.,0.));
#90104=CARTESIAN_POINT('Origin',(527.,0.,0.));
#90105=CARTESIAN_POINT('Origin',(518.,9.96288198200727,-4.9437822173509));
#90106=CARTESIAN_POINT('Origin',(518.,9.26309883354377,-8.27314933988261));
#90107=CARTESIAN_POINT('',(527.,8.96580705540569,-7.97585756174453));
#90108=CARTESIAN_POINT('Origin',(518.,7.35391052434009,-8.34386001800126));
#90109=CARTESIAN_POINT('',(527.,7.97585756174453,-8.9658070554057));
#90110=CARTESIAN_POINT('Origin',(527.,0.,0.));
#90111=CARTESIAN_POINT('Origin',(518.,6.1562177826491,-9.26288198200727));
#90112=CARTESIAN_POINT('Origin',(527.,0.,0.));
#90113=CARTESIAN_POINT('Origin',(527.,0.,0.));
#90114=CARTESIAN_POINT('',(527.,3.77668789453882,-11.3901987931398));
#90115=CARTESIAN_POINT('Origin',(518.,2.19674332223563,-10.9029500033804));
#90116=CARTESIAN_POINT('',(527.,2.42439173773412,-11.7525454562834));
#90117=CARTESIAN_POINT('Origin',(518.,3.8855042376736,-11.7963069144127));
#90118=CARTESIAN_POINT('Origin',(518.,0.699999999999998,-12.4));
#90119=CARTESIAN_POINT('',(527.,0.699999999999998,-11.9795659353751));
#90120=CARTESIAN_POINT('Origin',(518.,-0.700000000000002,-11.1));
#90121=CARTESIAN_POINT('',(527.,-0.700000000000002,-11.9795659353751));
#90122=CARTESIAN_POINT('Origin',(527.,0.,0.));
#90123=CARTESIAN_POINT('Origin',(518.,-2.19674332223564,-10.9029500033804));
#90124=CARTESIAN_POINT('Origin',(527.,0.,0.));
#90125=CARTESIAN_POINT('Origin',(527.,0.,0.));
#90126=CARTESIAN_POINT('',(527.,-5.38356518503846,-10.7246084263455));
#90127=CARTESIAN_POINT('Origin',(518.,-6.15621778264911,-9.26288198200726));
#90128=CARTESIAN_POINT('',(527.,-6.59600075033667,-10.0246084263455));
#90129=CARTESIAN_POINT('Origin',(518.,-5.5937822173509,-11.088715006927));
#90130=CARTESIAN_POINT('Origin',(518.,-8.27314933988261,-9.26309883354377));
#90131=CARTESIAN_POINT('',(527.,-7.97585756174453,-8.96580705540569));
#90132=CARTESIAN_POINT('Origin',(518.,-8.34386001800126,-7.35391052434009));
#90133=CARTESIAN_POINT('',(527.,-8.9658070554057,-7.97585756174453));
#90134=CARTESIAN_POINT('Origin',(527.,0.,0.));
#90135=CARTESIAN_POINT('Origin',(518.,-9.26288198200727,-6.1562177826491));
#90136=CARTESIAN_POINT('Origin',(527.,0.,0.));
#90137=CARTESIAN_POINT('Origin',(527.,0.,0.));
#90138=CARTESIAN_POINT('',(527.,-11.3901987931398,-3.77668789453882));
#90139=CARTESIAN_POINT('Origin',(518.,-10.9029500033804,-2.19674332223563));
#90140=CARTESIAN_POINT('',(527.,-11.7525454562834,-2.42439173773412));
#90141=CARTESIAN_POINT('Origin',(518.,-11.7963069144127,-3.8855042376736));
#90142=CARTESIAN_POINT('Origin',(518.,-12.4,-0.699999999999998));
#90143=CARTESIAN_POINT('',(527.,-11.9795659353751,-0.699999999999998));
#90144=CARTESIAN_POINT('Origin',(518.,-11.1,0.700000000000001));
#90145=CARTESIAN_POINT('',(527.,-11.9795659353751,0.700000000000002));
#90146=CARTESIAN_POINT('Origin',(527.,0.,0.));
#90147=CARTESIAN_POINT('Origin',(518.,-10.9029500033804,2.19674332223564));
#90148=CARTESIAN_POINT('Origin',(527.,0.,0.));
#90149=CARTESIAN_POINT('Origin',(527.,0.,0.));
#90150=CARTESIAN_POINT('',(527.,-10.7246084263455,5.38356518503846));
#90151=CARTESIAN_POINT('Origin',(518.,-9.26288198200727,6.15621778264911));
#90152=CARTESIAN_POINT('',(527.,-10.0246084263455,6.59600075033667));
#90153=CARTESIAN_POINT('Origin',(518.,-11.088715006927,5.5937822173509));
#90154=CARTESIAN_POINT('Origin',(518.,-9.26309883354377,8.27314933988261));
#90155=CARTESIAN_POINT('',(527.,-8.9658070554057,7.97585756174453));
#90156=CARTESIAN_POINT('Origin',(518.,-7.35391052434009,8.34386001800126));
#90157=CARTESIAN_POINT('',(527.,-7.97585756174453,8.9658070554057));
#90158=CARTESIAN_POINT('Origin',(527.,0.,0.));
#90159=CARTESIAN_POINT('Origin',(518.,-6.1562177826491,9.26288198200727));
#90160=CARTESIAN_POINT('Origin',(527.,0.,0.));
#90161=CARTESIAN_POINT('Origin',(527.,0.,0.));
#90162=CARTESIAN_POINT('',(527.,-3.77668789453882,11.3901987931398));
#90163=CARTESIAN_POINT('Origin',(518.,-2.19674332223563,10.9029500033804));
#90164=CARTESIAN_POINT('',(527.,-2.42439173773413,11.7525454562834));
#90165=CARTESIAN_POINT('Origin',(518.,-3.8855042376736,11.7963069144127));
#90166=CARTESIAN_POINT('Origin',(518.,-0.699999999999999,12.4));
#90167=CARTESIAN_POINT('',(527.,-0.699999999999999,11.9795659353751));
#90168=CARTESIAN_POINT('Origin',(518.,0.700000000000001,11.1));
#90169=CARTESIAN_POINT('',(527.,0.700000000000001,11.9795659353751));
#90170=CARTESIAN_POINT('Origin',(527.,0.,0.));
#90171=CARTESIAN_POINT('Origin',(518.,2.19674332223563,10.9029500033804));
#90172=CARTESIAN_POINT('Origin',(527.,0.,0.));
#90173=CARTESIAN_POINT('Origin',(527.,0.,0.));
#90174=CARTESIAN_POINT('',(527.,5.38356518503846,10.7246084263455));
#90175=CARTESIAN_POINT('Origin',(518.,6.15621778264911,9.26288198200727));
#90176=CARTESIAN_POINT('',(527.,6.59600075033667,10.0246084263455));
#90177=CARTESIAN_POINT('Origin',(518.,5.59378221735089,11.088715006927));
#90178=CARTESIAN_POINT('Origin',(518.,8.27314933988261,9.26309883354377));
#90179=CARTESIAN_POINT('',(527.,7.97585756174453,8.9658070554057));
#90180=CARTESIAN_POINT('Origin',(518.,8.34386001800126,7.35391052434009));
#90181=CARTESIAN_POINT('',(527.,8.9658070554057,7.97585756174453));
#90182=CARTESIAN_POINT('Origin',(527.,0.,0.));
#90183=CARTESIAN_POINT('Origin',(518.,9.26288198200727,6.1562177826491));
#90184=CARTESIAN_POINT('Origin',(527.,0.,0.));
#90185=CARTESIAN_POINT('Origin',(527.,0.,0.));
#90186=CARTESIAN_POINT('',(527.,11.3901987931398,3.77668789453882));
#90187=CARTESIAN_POINT('Origin',(518.,10.9029500033804,2.19674332223563));
#90188=CARTESIAN_POINT('',(527.,11.7525454562834,2.42439173773413));
#90189=CARTESIAN_POINT('Origin',(518.,11.7963069144127,3.8855042376736));
#90190=CARTESIAN_POINT('Origin',(518.,11.1,0.7));
#90191=CARTESIAN_POINT('Origin',(535.7,0.,0.));
#90192=CARTESIAN_POINT('Origin',(527.,0.,0.));
#90351=UNCERTAINTY_MEASURE_WITH_UNIT(LENGTH_MEASURE(0.01),#90375,
'DISTANCE_ACCURACY_VALUE',
'Maximum model space distance between geometric entities at asserted c
onnectivities');
#90355=UNCERTAINTY_MEASURE_WITH_UNIT(LENGTH_MEASURE(0.01),#90375,
'DISTANCE_ACCURACY_VALUE',
'Maximum model space distance between geometric entities at asserted c
onnectivities');
#90370=(
GEOMETRIC_REPRESENTATION_CONTEXT(3)
GLOBAL_UNCERTAINTY_ASSIGNED_CONTEXT((#90351))
GLOBAL_UNIT_ASSIGNED_CONTEXT((#90375,#90377,#90378))
REPRESENTATION_CONTEXT('','3D')
);
#90374=(
GEOMETRIC_REPRESENTATION_CONTEXT(3)
GLOBAL_UNCERTAINTY_ASSIGNED_CONTEXT((#90355))
GLOBAL_UNIT_ASSIGNED_CONTEXT((#90375,#90377,#90378))
REPRESENTATION_CONTEXT('','3D')
);
#90375=(
LENGTH_UNIT()
NAMED_UNIT(*)
SI_UNIT(.MILLI.,.METRE.)
);
#90377=(
NAMED_UNIT(*)
PLANE_ANGLE_UNIT()
SI_UNIT($,.RADIAN.)
);
#90378=(
NAMED_UNIT(*)
SI_UNIT($,.STERADIAN.)
SOLID_ANGLE_UNIT()
);
#90393=SHAPE_DEFINITION_REPRESENTATION(#90411,#90454);
#90411=PRODUCT_DEFINITION_SHAPE('',$,#90473);
#90454=SHAPE_REPRESENTATION('',(#44809),#90370);
#90458=PRODUCT_DEFINITION_CONTEXT('part definition',#90514,'design');
#90473=PRODUCT_DEFINITION('2026-10-11-12-53-14-838','14_Tripod_Spider',
#90491,#90458);
#90491=PRODUCT_DEFINITION_FORMATION('',$,#90530);
#90514=APPLICATION_CONTEXT(
'Core Data for Automotive Mechanical Design Process');
#90515=PRODUCT_CONTEXT('part definition',#90514,'mechanical');
#90530=PRODUCT('2026-10-11-12-53-14-838','14_Tripod_Spider',$,(#90515));
#90667=COLOUR_RGB('Light Blue',0.38,0.62,0.78);
#90668=FILL_AREA_STYLE_COLOUR('',#90667);
#90669=FILL_AREA_STYLE('',(#90668));
#90670=SURFACE_STYLE_FILL_AREA(#90669);
#90671=SURFACE_SIDE_STYLE('',(#90670));
#90672=SURFACE_STYLE_USAGE(.BOTH.,#90671);
#90673=PRESENTATION_STYLE_ASSIGNMENT((#90672));
ENDSEC;
END-ISO-10303-21;
